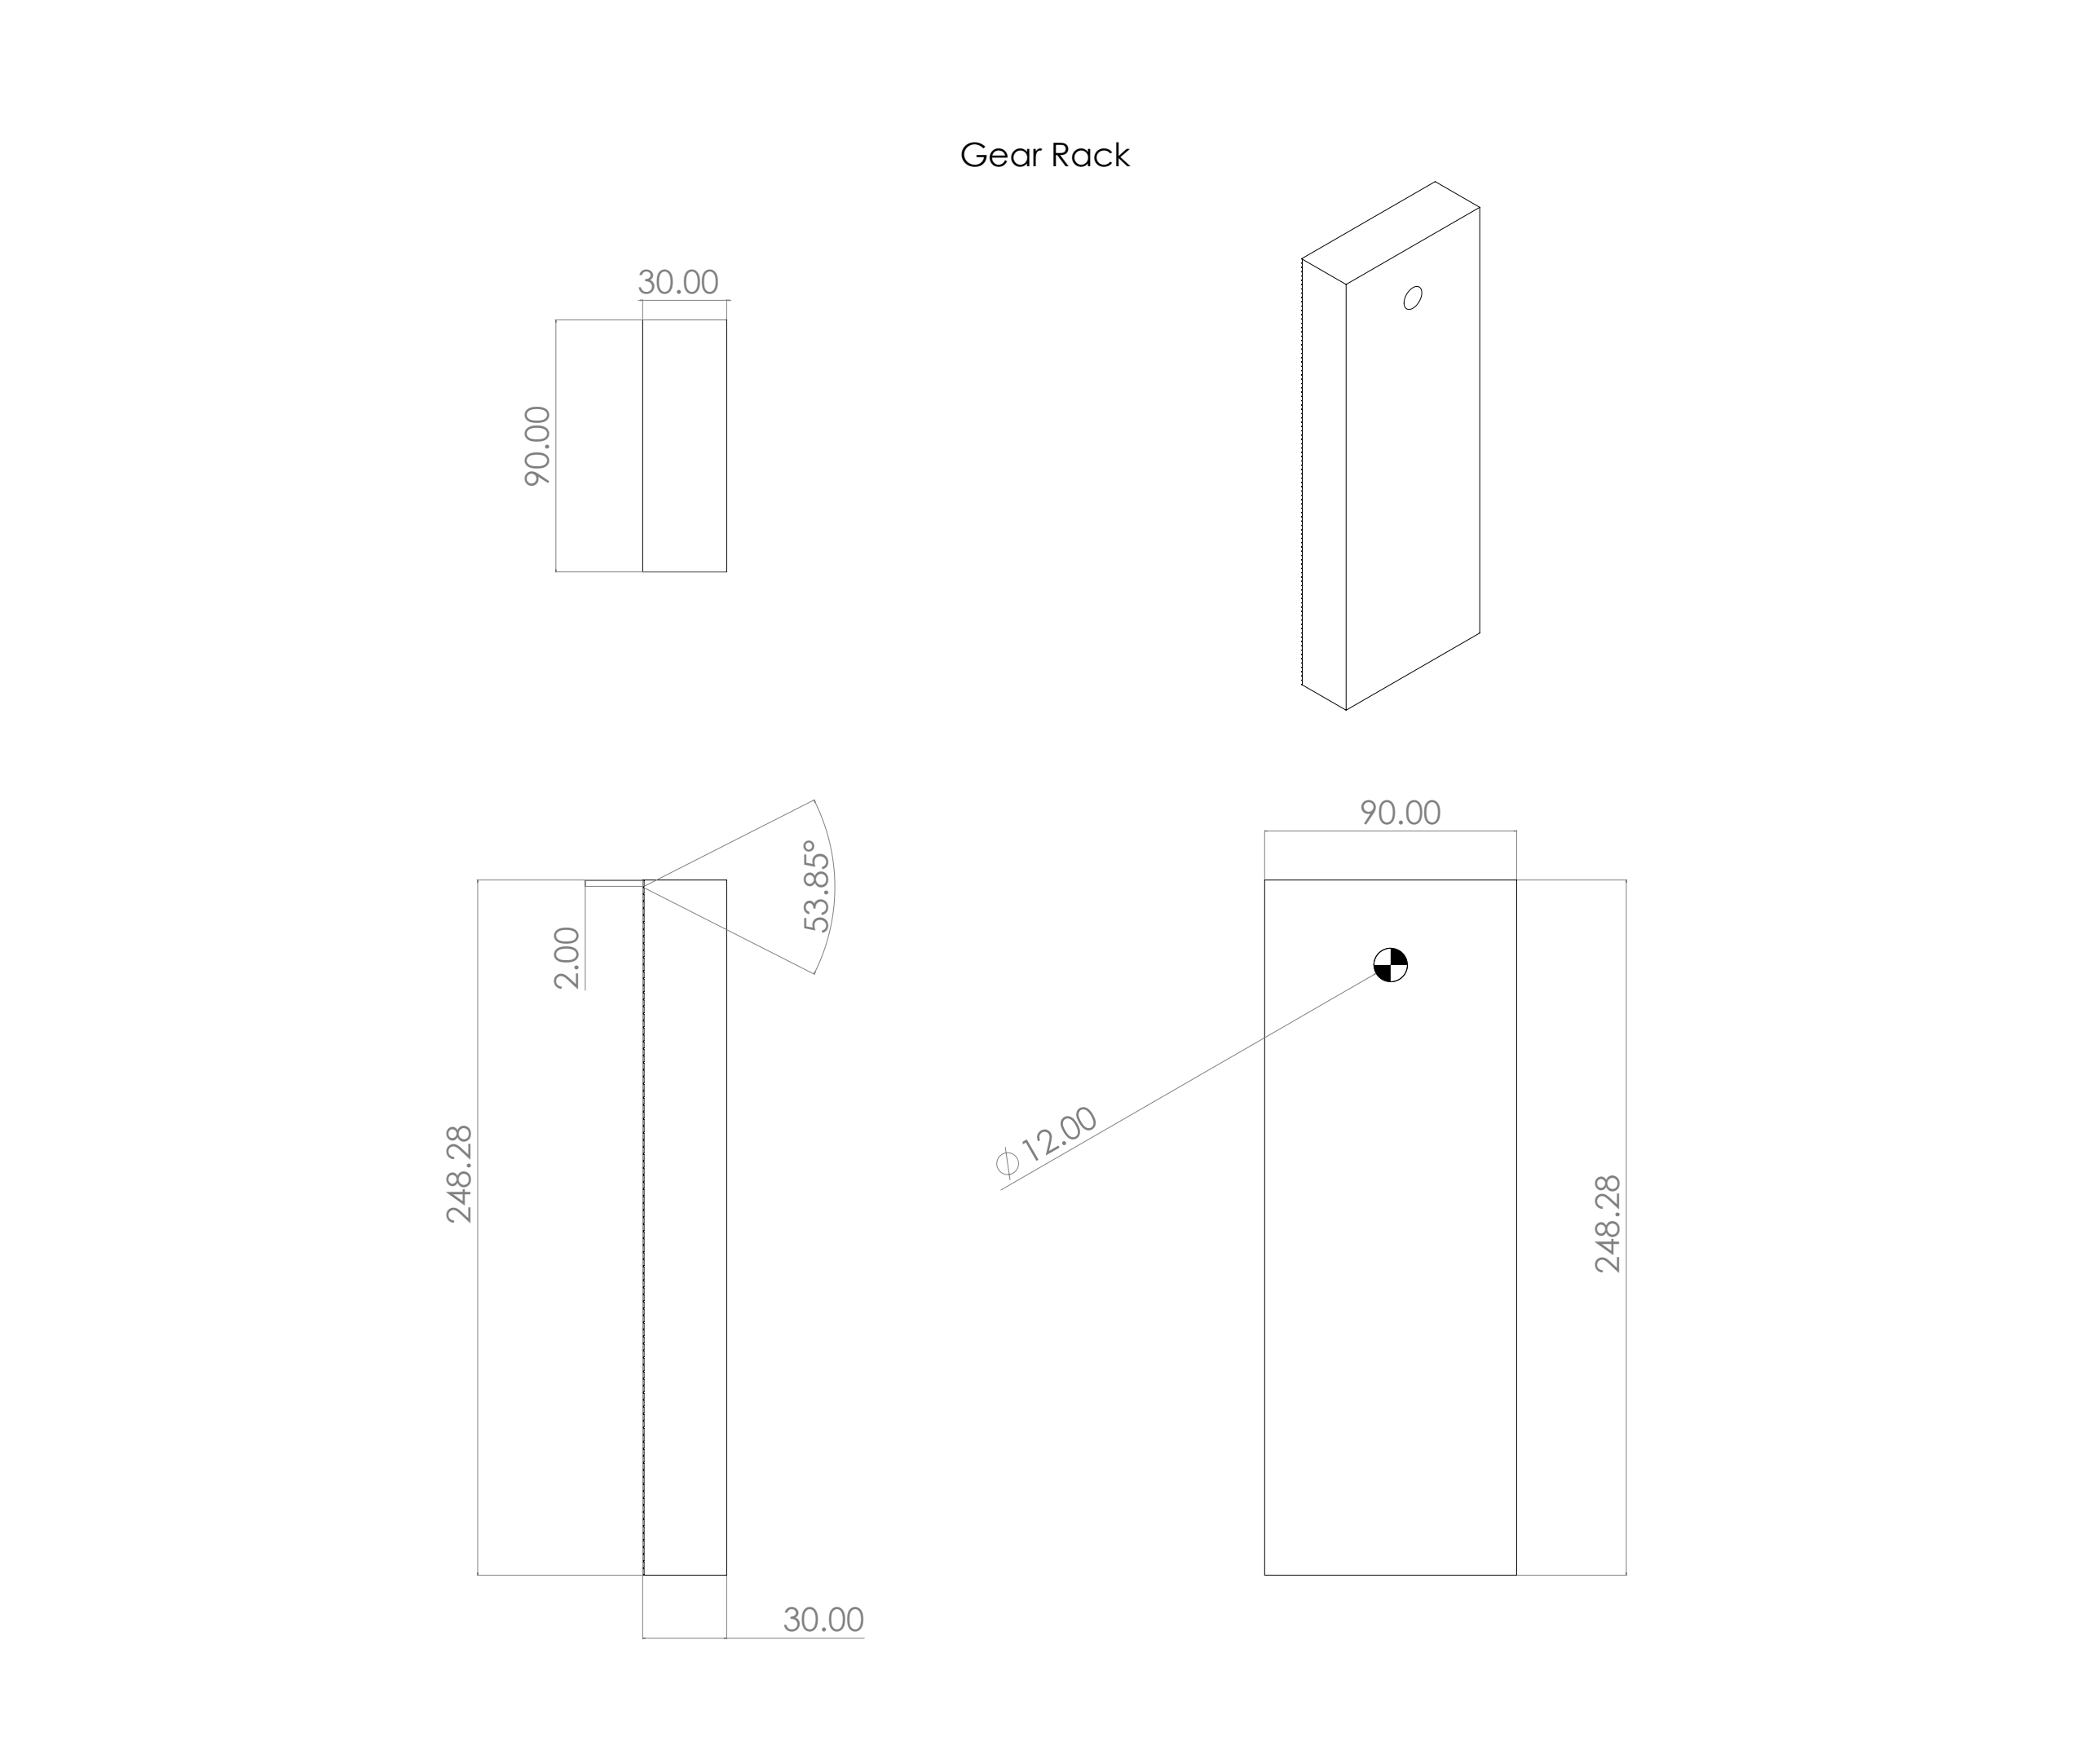
ISO-10303-21;
HEADER;
FILE_DESCRIPTION (('STEP AP214'),
    '1' );
FILE_NAME ('Gear Rack.step',
    '2026-10-24T00:09:50',
    ( '' ),
    ( '' ),
    'SwSTEP 2.0',
    'SolidWorks 2025',
    '' );
FILE_SCHEMA (( 'AUTOMOTIVE_DESIGN' ));
ENDSEC;

DATA;
#4=ORIENTED_EDGE ( 'NONE', *, *, #26664, .T. ) ;
#8=ORIENTED_EDGE ( 'NONE', *, *, #11531, .F. ) ;
#19=EDGE_CURVE ( 'NONE', #26943, #26049, #15367, .T. ) ;
#20=CARTESIAN_POINT ( 'NONE',  ( 157.4999999999998579, 83.32081209086616980, 45.00000000000000000 ) ) ;
#25=CARTESIAN_POINT ( 'NONE',  ( 187.4999999999996305, 288.9665627064425166, 45.00000000000000000 ) ) ;
#27=ORIENTED_EDGE ( 'NONE', *, *, #22527, .F. ) ;
#29=CARTESIAN_POINT ( 'NONE',  ( 157.4999999999998579, 105.8916871584295478, 45.00000000000000000 ) ) ;
#30=CARTESIAN_POINT ( 'NONE',  ( 158.0000000000016485, 50.46449948952111697, 45.00000000000000000 ) ) ;
#31=LINE ( 'NONE', #28308, #26698 ) ;
#33=ORIENTED_EDGE ( 'NONE', *, *, #12258, .T. ) ;
#34=EDGE_CURVE ( 'NONE', #22143, #25491, #9030, .T. ) ;
#35=DIRECTION ( 'NONE',  ( -0.8916010070293783896, -0.4528218681382319422, 0.000000000000000000 ) ) ;
#36=VECTOR ( 'NONE', #4972, 999.9999999999998863 ) ;
#37=CARTESIAN_POINT ( 'NONE',  ( 158.0000000000006821, 140.7479997597746433, 45.00000000000000000 ) ) ;
#39=ORIENTED_EDGE ( 'NONE', *, *, #23270, .T. ) ;
#41=EDGE_CURVE ( 'NONE', #5835, #23775, #13490, .T. ) ;
#48=FACE_OUTER_BOUND ( 'NONE', #22018, .T. ) ;
#49=ORIENTED_EDGE ( 'NONE', *, *, #10620, .T. ) ;
#54=EDGE_CURVE ( 'NONE', #1139, #21808, #13638, .T. ) ;
#56=CARTESIAN_POINT ( 'NONE',  ( 158.0000000000000568, 203.4448749474510407, 45.00000000000000000 ) ) ;
#57=CARTESIAN_POINT ( 'NONE',  ( 158.0000000000006821, 138.7479997597746433, 45.00000000000000000 ) ) ;
#58=DIRECTION ( 'NONE',  ( -0.000000000000000000, -0.000000000000000000, -1.000000000000000000 ) ) ;
#60=LINE ( 'NONE', #17580, #15416 ) ;
#61=VERTEX_POINT ( 'NONE', #7448 ) ;
#62=DIRECTION ( 'NONE',  ( 0.000000000000000000, 0.000000000000000000, 1.000000000000000000 ) ) ;
#64=FACE_OUTER_BOUND ( 'NONE', #25797, .T. ) ;
#65=CARTESIAN_POINT ( 'NONE',  ( 157.4999999999998579, 93.35231212089433939, 45.00000000000000000 ) ) ;
#68=CARTESIAN_POINT ( 'NONE',  ( 157.4999999999998579, 98.36806213590843129, -45.00000000000000000 ) ) ;
#70=VECTOR ( 'NONE', #14918, 1000.000000000000114 ) ;
#77=VECTOR ( 'NONE', #23464, 999.9999999999998863 ) ;
#81=ORIENTED_EDGE ( 'NONE', *, *, #14673, .T. ) ;
#83=VERTEX_POINT ( 'NONE', #22814 ) ;
#85=ORIENTED_EDGE ( 'NONE', *, *, #17813, .T. ) ;
#87=ORIENTED_EDGE ( 'NONE', *, *, #18331, .F. ) ;
#91=AXIS2_PLACEMENT_3D ( 'NONE', #3202, #20878, #24911 ) ;
#92=DIRECTION ( 'NONE',  ( 0.8916010070295410372, -0.4528218681379115873, 0.000000000000000000 ) ) ;
#96=LINE ( 'NONE', #11159, #22961 ) ;
#100=DIRECTION ( 'NONE',  ( 0.000000000000000000, -1.000000000000000000, 0.000000000000000000 ) ) ;
#105=PLANE ( 'NONE',  #22522 ) ;
#106=DIRECTION ( 'NONE',  ( 0.8916010070293283185, 0.4528218681383305855, 0.000000000000000000 ) ) ;
#107=CARTESIAN_POINT ( 'NONE',  ( 158.0000000000012221, 88.59049960963380954, -45.00000000000000000 ) ) ;
#110=ORIENTED_EDGE ( 'NONE', *, *, #7705, .T. ) ;
#111=EDGE_CURVE ( 'NONE', #4742, #22382, #9467, .T. ) ;
#112=VECTOR ( 'NONE', #9793, 1000.000000000000000 ) ;
#114=EDGE_LOOP ( 'NONE', ( #13763, #3696, #24044, #20717 ) ) ;
#116=ORIENTED_EDGE ( 'NONE', *, *, #27781, .F. ) ;
#123=DIRECTION ( 'NONE',  ( 0.8916010070293710621, -0.4528218681382463195, 0.000000000000000000 ) ) ;
#127=VECTOR ( 'NONE', #25950, 1000.000000000000000 ) ;
#129=LINE ( 'NONE', #12656, #21109 ) ;
#131=VECTOR ( 'NONE', #4235, 1000.000000000000000 ) ;
#137=FACE_OUTER_BOUND ( 'NONE', #15642, .T. ) ;
#138=VECTOR ( 'NONE', #24642, 1000.000000000000000 ) ;
#143=LINE ( 'NONE', #23706, #15280 ) ;
#150=DIRECTION ( 'NONE',  ( 0.000000000000000000, -1.000000000000000000, 0.000000000000000000 ) ) ;
#151=ORIENTED_EDGE ( 'NONE', *, *, #11275, .F. ) ;
#152=VERTEX_POINT ( 'NONE', #25244 ) ;
#153=VECTOR ( 'NONE', #12581, 1000.000000000000000 ) ;
#161=CARTESIAN_POINT ( 'NONE',  ( 157.9999999999996589, 279.1890001801680796, 45.00000000000000000 ) ) ;
#162=ORIENTED_EDGE ( 'NONE', *, *, #25176, .F. ) ;
#167=VECTOR ( 'NONE', #6302, 1000.000000000000000 ) ;
#169=EDGE_CURVE ( 'NONE', #1220, #7618, #16907, .T. ) ;
#170=VERTEX_POINT ( 'NONE', #23513 ) ;
#172=DIRECTION ( 'NONE',  ( 0.8916010070298353574, -0.4528218681373320509, 0.000000000000000000 ) ) ;
#174=CARTESIAN_POINT ( 'NONE',  ( 158.0000000000004832, 161.3188748273380213, 45.00000000000000000 ) ) ;
#176=VECTOR ( 'NONE', #1198, 1000.000000000000000 ) ;
#179=LINE ( 'NONE', #13127, #5008 ) ;
#180=ADVANCED_FACE ( 'NONE', ( #3827 ), #7726, .F. ) ;
#189=EDGE_LOOP ( 'NONE', ( #11478, #20043, #1558, #19553 ) ) ;
#190=VECTOR ( 'NONE', #9323, 1000.000000000000227 ) ;
#191=ORIENTED_EDGE ( 'NONE', *, *, #11968, .F. ) ;
#199=CARTESIAN_POINT ( 'NONE',  ( 157.4999999999997442, 253.8563126013445697, -45.00000000000000000 ) ) ;
#200=CARTESIAN_POINT ( 'NONE',  ( 158.0000000000017053, 45.44874947450702507, 45.00000000000000000 ) ) ;
#207=EDGE_LOOP ( 'NONE', ( #12910, #1760, #26526, #6163 ) ) ;
#208=LINE ( 'NONE', #21895, #12696 ) ;
#216=CARTESIAN_POINT ( 'NONE',  ( 158.0000000000001421, 191.4133749174225443, 45.00000000000000000 ) ) ;
#217=LINE ( 'NONE', #22769, #1813 ) ;
#219=ORIENTED_EDGE ( 'NONE', *, *, #15468, .T. ) ;
#222=VECTOR ( 'NONE', #16891, 1000.000000000000000 ) ;
#224=ADVANCED_FACE ( 'NONE', ( #25661 ), #17044, .F. ) ;
#226=VERTEX_POINT ( 'NONE', #23659 ) ;
#228=FACE_OUTER_BOUND ( 'NONE', #26705, .T. ) ;
#229=ORIENTED_EDGE ( 'NONE', *, *, #19889, .T. ) ;
#231=DIRECTION ( 'NONE',  ( 1.000000000000000000, 0.000000000000000000, -0.000000000000000000 ) ) ;
#233=ORIENTED_EDGE ( 'NONE', *, *, #12489, .T. ) ;
#237=VECTOR ( 'NONE', #8756, 1000.000000000000000 ) ;
#244=DIRECTION ( 'NONE',  ( -0.000000000000000000, -0.000000000000000000, -1.000000000000000000 ) ) ;
#247=CARTESIAN_POINT ( 'NONE',  ( 158.0000000000007674, 133.2243747372535267, -45.00000000000000000 ) ) ;
#248=CARTESIAN_POINT ( 'NONE',  ( 158.0000000000003411, 173.8582498648732440, -45.00000000000000000 ) ) ;
#249=LINE ( 'NONE', #6703, #21167 ) ;
#252=ORIENTED_EDGE ( 'NONE', *, *, #25685, .T. ) ;
#258=VECTOR ( 'NONE', #9581, 1000.000000000000000 ) ;
#265=ORIENTED_EDGE ( 'NONE', *, *, #8156, .T. ) ;
#271=CARTESIAN_POINT ( 'NONE',  ( 157.4999999999998579, 183.6358123911478799, 45.00000000000000000 ) ) ;
#273=VECTOR ( 'NONE', #6730, 1000.000000000000000 ) ;
#276=EDGE_CURVE ( 'NONE', #11934, #27327, #6832, .T. ) ;
#278=EDGE_CURVE ( 'NONE', #18107, #2726, #15475, .T. ) ;
#281=PLANE ( 'NONE',  #14960 ) ;
#284=CARTESIAN_POINT ( 'NONE',  ( 157.4999999999998579, 163.5728123310915407, 45.00000000000000000 ) ) ;
#287=LINE ( 'NONE', #25846, #26979 ) ;
#289=LINE ( 'NONE', #2568, #5884 ) ;
#293=ORIENTED_EDGE ( 'NONE', *, *, #15468, .F. ) ;
#296=DIRECTION ( 'NONE',  ( -0.000000000000000000, -0.000000000000000000, -1.000000000000000000 ) ) ;
#298=ORIENTED_EDGE ( 'NONE', *, *, #15430, .T. ) ;
#299=ORIENTED_EDGE ( 'NONE', *, *, #27948, .T. ) ;
#300=VECTOR ( 'NONE', #28359, 1000.000000000000000 ) ;
#302=LINE ( 'NONE', #15395, #9767 ) ;
#306=ORIENTED_EDGE ( 'NONE', *, *, #8739, .F. ) ;
#307=CARTESIAN_POINT ( 'NONE',  ( 157.4999999999996589, 276.4271876689075498, 45.00000000000000000 ) ) ;
#314=ADVANCED_FACE ( 'NONE', ( #8712 ), #4110, .F. ) ;
#321=PLANE ( 'NONE',  #16025 ) ;
#326=DIRECTION ( 'NONE',  ( -0.8916010070300282031, 0.4528218681369524101, 0.000000000000000000 ) ) ;
#329=ORIENTED_EDGE ( 'NONE', *, *, #12094, .T. ) ;
#330=ORIENTED_EDGE ( 'NONE', *, *, #4768, .T. ) ;
#333=ORIENTED_EDGE ( 'NONE', *, *, #4508, .T. ) ;
#334=VECTOR ( 'NONE', #5178, 1000.000000000000000 ) ;
#344=ADVANCED_FACE ( 'NONE', ( #18569 ), #902, .F. ) ;
#345=FACE_OUTER_BOUND ( 'NONE', #10535, .T. ) ;
#346=DIRECTION ( 'NONE',  ( 1.000000000000000000, 0.000000000000000000, -0.000000000000000000 ) ) ;
#350=PLANE ( 'NONE',  #14058 ) ;
#351=ORIENTED_EDGE ( 'NONE', *, *, #20821, .F. ) ;
#353=LINE ( 'NONE', #9111, #26676 ) ;
#354=CARTESIAN_POINT ( 'NONE',  ( 158.0000000000009095, 118.6849996997183041, -45.00000000000000000 ) ) ;
#355=CARTESIAN_POINT ( 'NONE',  ( 158.0000000000011937, 91.09837461714084839, 45.00000000000000000 ) ) ;
#357=ORIENTED_EDGE ( 'NONE', *, *, #17681, .T. ) ;
#358=CARTESIAN_POINT ( 'NONE',  ( 157.4999999999998579, 75.79718706834503905, -45.00000000000000000 ) ) ;
#359=ORIENTED_EDGE ( 'NONE', *, *, #19187, .F. ) ;
#360=LINE ( 'NONE', #2786, #27655 ) ;
#363=ORIENTED_EDGE ( 'NONE', *, *, #1797, .T. ) ;
#364=DIRECTION ( 'NONE',  ( -0.000000000000000000, -0.000000000000000000, -1.000000000000000000 ) ) ;
#367=CARTESIAN_POINT ( 'NONE',  ( 158.0000000000009948, 110.6534996696901345, 45.00000000000000000 ) ) ;
#369=DIRECTION ( 'NONE',  ( 0.4528218681382713551, -0.8916010070293584056, 0.000000000000000000 ) ) ;
#372=VERTEX_POINT ( 'NONE', #14405 ) ;
#374=ORIENTED_EDGE ( 'NONE', *, *, #24300, .F. ) ;
#375=VECTOR ( 'NONE', #26131, 1000.000000000000000 ) ;
#376=EDGE_CURVE ( 'NONE', #12778, #5204, #20994, .T. ) ;
#378=VERTEX_POINT ( 'NONE', #12116 ) ;
#382=DIRECTION ( 'NONE',  ( 0.4528218681372921939, 0.8916010070298556744, -0.000000000000000000 ) ) ;
#386=EDGE_CURVE ( 'NONE', #7620, #226, #11835, .T. ) ;
#387=VECTOR ( 'NONE', #7151, 1000.000000000000000 ) ;
#389=LINE ( 'NONE', #22364, #14037 ) ;
#390=CARTESIAN_POINT ( 'NONE',  ( 158.0000000000001990, 188.3976249024084666, 45.00000000000000000 ) ) ;
#391=LINE ( 'NONE', #13469, #619 ) ;
#392=EDGE_LOOP ( 'NONE', ( #28228, #13403, #15144, #3135 ) ) ;
#394=AXIS2_PLACEMENT_3D ( 'NONE', #22078, #2964, #5263 ) ;
#397=DIRECTION ( 'NONE',  ( -0.8916010070293711731, 0.4528218681382463751, 0.000000000000000000 ) ) ;
#405=ORIENTED_EDGE ( 'NONE', *, *, #27601, .F. ) ;
#410=VERTEX_POINT ( 'NONE', #9531 ) ;
#412=PLANE ( 'NONE',  #4933 ) ;
#413=LINE ( 'NONE', #26684, #6547 ) ;
#418=EDGE_CURVE ( 'NONE', #905, #12668, #18291, .T. ) ;
#422=EDGE_CURVE ( 'NONE', #9422, #12999, #20714, .T. ) ;
#423=CARTESIAN_POINT ( 'NONE',  ( 158.0000000000015348, 58.49599951954928656, -45.00000000000000000 ) ) ;
#424=CARTESIAN_POINT ( 'NONE',  ( 158.0000000000016485, 48.46449948952110987, -45.00000000000000000 ) ) ;
#432=CARTESIAN_POINT ( 'NONE',  ( 158.0000000000015632, 57.98812451204224061, 45.00000000000000000 ) ) ;
#435=EDGE_LOOP ( 'NONE', ( #624, #23156, #10826, #824 ) ) ;
#436=EDGE_CURVE ( 'NONE', #9697, #410, #7928, .T. ) ;
#437=DIRECTION ( 'NONE',  ( -0.000000000000000000, 0.000000000000000000, -1.000000000000000000 ) ) ;
#448=EDGE_CURVE ( 'NONE', #7332, #22290, #1039, .T. ) ;
#450=LINE ( 'NONE', #307, #16398 ) ;
#454=DIRECTION ( 'NONE',  ( 0.000000000000000000, -1.000000000000000000, 0.000000000000000000 ) ) ;
#455=LINE ( 'NONE', #4177, #5667 ) ;
#456=VECTOR ( 'NONE', #13195, 1000.000000000000000 ) ;
#458=LINE ( 'NONE', #9217, #23812 ) ;
#461=DIRECTION ( 'NONE',  ( 1.000000000000000000, 0.000000000000000000, -0.000000000000000000 ) ) ;
#464=CARTESIAN_POINT ( 'NONE',  ( 158.0000000000012790, 83.57474959461971764, -45.00000000000000000 ) ) ;
#465=VERTEX_POINT ( 'NONE', #23870 ) ;
#477=VERTEX_POINT ( 'NONE', #6332 ) ;
#478=ORIENTED_EDGE ( 'NONE', *, *, #3698, .F. ) ;
#479=DIRECTION ( 'NONE',  ( -0.8916010070298252543, 0.4528218681373520904, 0.000000000000000000 ) ) ;
#482=CARTESIAN_POINT ( 'NONE',  ( 157.4999999999998579, 63.25781203080982351, 45.00000000000000000 ) ) ;
#485=VECTOR ( 'NONE', #5220, 999.9999999999998863 ) ;
#486=EDGE_CURVE ( 'NONE', #2468, #22451, #19269, .T. ) ;
#487=CARTESIAN_POINT ( 'NONE',  ( 158.0000000000007390, 135.7322497447605656, -45.00000000000000000 ) ) ;
#495=EDGE_CURVE ( 'NONE', #465, #26764, #24012, .T. ) ;
#497=DIRECTION ( 'NONE',  ( -0.8916010070293783896, -0.4528218681382319422, 0.000000000000000000 ) ) ;
#503=DIRECTION ( 'NONE',  ( -0.000000000000000000, -0.000000000000000000, -1.000000000000000000 ) ) ;
#507=CARTESIAN_POINT ( 'NONE',  ( 158.0000000000009663, 113.1613746771971876, 45.00000000000000000 ) ) ;
#510=ADVANCED_FACE ( 'NONE', ( #1873 ), #18986, .F. ) ;
#513=EDGE_LOOP ( 'NONE', ( #20470, #9702, #23689, #21030 ) ) ;
#514=EDGE_CURVE ( 'NONE', #16325, #12071, #12961, .T. ) ;
#518=PLANE ( 'NONE',  #26438 ) ;
#524=LINE ( 'NONE', #27357, #13105 ) ;
#526=CARTESIAN_POINT ( 'NONE',  ( 158.0000000000002274, 183.8897498949014278, 45.00000000000000000 ) ) ;
#532=CARTESIAN_POINT ( 'NONE',  ( 157.4999999999998579, 105.8916871584295478, -45.00000000000000000 ) ) ;
#534=LINE ( 'NONE', #11755, #24010 ) ;
#537=CARTESIAN_POINT ( 'NONE',  ( 157.4999999999998010, 241.3169375638095460, -45.00000000000000000 ) ) ;
#540=CARTESIAN_POINT ( 'NONE',  ( 157.4999999999998579, 191.1594374136689964, -45.00000000000000000 ) ) ;
#542=PLANE ( 'NONE',  #20720 ) ;
#543=VERTEX_POINT ( 'NONE', #17395 ) ;
#546=EDGE_CURVE ( 'NONE', #991, #20740, #6197, .T. ) ;
#547=CARTESIAN_POINT ( 'NONE',  ( 157.4999999999998579, 153.5413123010633853, 45.00000000000000000 ) ) ;
#548=VERTEX_POINT ( 'NONE', #21136 ) ;
#552=ORIENTED_EDGE ( 'NONE', *, *, #17681, .F. ) ;
#563=CARTESIAN_POINT ( 'NONE',  ( 157.9999999999996874, 268.6496251426330559, -45.00000000000000000 ) ) ;
#564=LINE ( 'NONE', #17941, #18623 ) ;
#569=CARTESIAN_POINT ( 'NONE',  ( 157.9999999999998010, 238.5551250525490161, 45.00000000000000000 ) ) ;
#571=VECTOR ( 'NONE', #26169, 1000.000000000000227 ) ;
#574=CARTESIAN_POINT ( 'NONE',  ( 158.0000000000013358, 78.55899957960562574, -45.00000000000000000 ) ) ;
#577=ORIENTED_EDGE ( 'NONE', *, *, #22638, .T. ) ;
#579=DIRECTION ( 'NONE',  ( -0.8916010070293783896, -0.4528218681382319422, 0.000000000000000000 ) ) ;
#580=AXIS2_PLACEMENT_3D ( 'NONE', #3424, #12354, #8027 ) ;
#582=ORIENTED_EDGE ( 'NONE', *, *, #19199, .T. ) ;
#583=VERTEX_POINT ( 'NONE', #15541 ) ;
#585=EDGE_CURVE ( 'NONE', #16172, #22496, #15834, .T. ) ;
#588=CARTESIAN_POINT ( 'NONE',  ( 157.9999999999998010, 236.5551250525490161, -45.00000000000000000 ) ) ;
#590=EDGE_LOOP ( 'NONE', ( #18071, #20954, #25827, #7929 ) ) ;
#602=EDGE_CURVE ( 'NONE', #11526, #18196, #21990, .T. ) ;
#608=EDGE_CURVE ( 'NONE', #5724, #21166, #15684, .T. ) ;
#615=VECTOR ( 'NONE', #20884, 1000.000000000000114 ) ;
#619=VECTOR ( 'NONE', #22222, 1000.000000000000000 ) ;
#620=VERTEX_POINT ( 'NONE', #11079 ) ;
#624=ORIENTED_EDGE ( 'NONE', *, *, #701, .T. ) ;
#628=DIRECTION ( 'NONE',  ( 0.4528218681370924092, 0.8916010070299572599, -0.000000000000000000 ) ) ;
#632=VECTOR ( 'NONE', #24895, 1000.000000000000000 ) ;
#633=DIRECTION ( 'NONE',  ( 1.000000000000000000, 0.000000000000000000, -0.000000000000000000 ) ) ;
#643=CARTESIAN_POINT ( 'NONE',  ( 158.0000000000003126, 176.3661248723802828, 45.00000000000000000 ) ) ;
#646=ORIENTED_EDGE ( 'NONE', *, *, #18826, .T. ) ;
#648=ORIENTED_EDGE ( 'NONE', *, *, #18190, .T. ) ;
#650=LINE ( 'NONE', #20465, #20665 ) ;
#652=ORIENTED_EDGE ( 'NONE', *, *, #23081, .T. ) ;
#655=VECTOR ( 'NONE', #25630, 1000.000000000000000 ) ;
#659=ORIENTED_EDGE ( 'NONE', *, *, #1539, .T. ) ;
#660=VECTOR ( 'NONE', #1060, 1000.000000000000114 ) ;
#664=EDGE_CURVE ( 'NONE', #22382, #5522, #13383, .T. ) ;
#666=ORIENTED_EDGE ( 'NONE', *, *, #14204, .T. ) ;
#670=EDGE_CURVE ( 'NONE', #15969, #22271, #11226, .T. ) ;
#679=CARTESIAN_POINT ( 'NONE',  ( 158.0000000000009379, 116.1771246922112653, 45.00000000000000000 ) ) ;
#685=DIRECTION ( 'NONE',  ( 1.000000000000000000, 0.000000000000000000, -0.000000000000000000 ) ) ;
#689=VERTEX_POINT ( 'NONE', #9212 ) ;
#692=VECTOR ( 'NONE', #27394, 1000.000000000000114 ) ;
#693=ORIENTED_EDGE ( 'NONE', *, *, #10754, .F. ) ;
#695=VERTEX_POINT ( 'NONE', #161 ) ;
#697=ORIENTED_EDGE ( 'NONE', *, *, #18565, .F. ) ;
#699=DIRECTION ( 'NONE',  ( 0.4528218681376512400, -0.8916010070296733758, 0.000000000000000000 ) ) ;
#701=EDGE_CURVE ( 'NONE', #9383, #10330, #21856, .T. ) ;
#711=CARTESIAN_POINT ( 'NONE',  ( 157.4999999999998579, 105.8916871584295478, 45.00000000000000000 ) ) ;
#712=CARTESIAN_POINT ( 'NONE',  ( 157.4999999999998579, 188.6515624061619576, 45.00000000000000000 ) ) ;
#713=CARTESIAN_POINT ( 'NONE',  ( 157.4999999999998579, 75.79718706834503905, 45.00000000000000000 ) ) ;
#723=ORIENTED_EDGE ( 'NONE', *, *, #775, .T. ) ;
#725=ORIENTED_EDGE ( 'NONE', *, *, #13975, .T. ) ;
#727=FACE_OUTER_BOUND ( 'NONE', #4250, .T. ) ;
#729=VERTEX_POINT ( 'NONE', #20 ) ;
#730=ORIENTED_EDGE ( 'NONE', *, *, #11239, .F. ) ;
#733=VECTOR ( 'NONE', #6685, 1000.000000000000227 ) ;
#734=CARTESIAN_POINT ( 'NONE',  ( 158.0000000000005400, 156.3031248123239436, 45.00000000000000000 ) ) ;
#735=EDGE_CURVE ( 'NONE', #14776, #17184, #8778, .T. ) ;
#736=CARTESIAN_POINT ( 'NONE',  ( 157.9999999999996589, 276.1732501651540588, 45.00000000000000000 ) ) ;
#738=AXIS2_PLACEMENT_3D ( 'NONE', #16780, #14771, #23524 ) ;
#741=LINE ( 'NONE', #5326, #18696 ) ;
#744=ADVANCED_FACE ( 'NONE', ( #5030 ), #27419, .F. ) ;
#745=LINE ( 'NONE', #26587, #14618 ) ;
#747=LINE ( 'NONE', #24592, #112 ) ;
#748=CARTESIAN_POINT ( 'NONE',  ( 157.4999999999998295, 228.7775625262745223, 45.00000000000000000 ) ) ;
#749=VERTEX_POINT ( 'NONE', #25137 ) ;
#753=CARTESIAN_POINT ( 'NONE',  ( 158.0000000000009095, 118.6849996997183041, 45.00000000000000000 ) ) ;
#756=ORIENTED_EDGE ( 'NONE', *, *, #4498, .T. ) ;
#758=EDGE_CURVE ( 'NONE', #11111, #19970, #7626, .T. ) ;
#759=LINE ( 'NONE', #16277, #22117 ) ;
#767=FACE_OUTER_BOUND ( 'NONE', #3565, .T. ) ;
#768=ORIENTED_EDGE ( 'NONE', *, *, #27927, .F. ) ;
#775=EDGE_CURVE ( 'NONE', #20816, #23826, #7896, .T. ) ;
#778=ORIENTED_EDGE ( 'NONE', *, *, #27716, .F. ) ;
#784=EDGE_LOOP ( 'NONE', ( #27213, #18467, #26244, #20332 ) ) ;
#785=DIRECTION ( 'NONE',  ( 0.000000000000000000, -1.000000000000000000, 0.000000000000000000 ) ) ;
#787=LINE ( 'NONE', #12142, #8871 ) ;
#791=DIRECTION ( 'NONE',  ( -0.000000000000000000, -0.000000000000000000, -1.000000000000000000 ) ) ;
#793=VECTOR ( 'NONE', #14680, 1000.000000000000000 ) ;
#794=EDGE_CURVE ( 'NONE', #15105, #2405, #20829, .T. ) ;
#798=ORIENTED_EDGE ( 'NONE', *, *, #12480, .F. ) ;
#799=EDGE_CURVE ( 'NONE', #12071, #26896, #5455, .T. ) ;
#800=VERTEX_POINT ( 'NONE', #13821 ) ;
#805=ORIENTED_EDGE ( 'NONE', *, *, #5908, .F. ) ;
#806=ORIENTED_EDGE ( 'NONE', *, *, #17778, .T. ) ;
#813=FACE_OUTER_BOUND ( 'NONE', #28354, .T. ) ;
#814=CARTESIAN_POINT ( 'NONE',  ( 158.0000000000003126, 176.3661248723802828, 45.00000000000000000 ) ) ;
#816=EDGE_CURVE ( 'NONE', #10360, #6691, #22989, .T. ) ;
#818=DIRECTION ( 'NONE',  ( 0.8916010070293510781, -0.4528218681382856770, 0.000000000000000000 ) ) ;
#824=ORIENTED_EDGE ( 'NONE', *, *, #23421, .T. ) ;
#826=LINE ( 'NONE', #12322, #17561 ) ;
#828=CARTESIAN_POINT ( 'NONE',  ( 158.0000000000009095, 118.6849996997183041, -45.00000000000000000 ) ) ;
#829=ORIENTED_EDGE ( 'NONE', *, *, #22521, .F. ) ;
#833=ORIENTED_EDGE ( 'NONE', *, *, #27551, .T. ) ;
#836=LINE ( 'NONE', #15335, #13752 ) ;
#837=DIRECTION ( 'NONE',  ( 0.8916010070295106171, -0.4528218681379715393, 0.000000000000000000 ) ) ;
#838=VECTOR ( 'NONE', #12878, 1000.000000000000000 ) ;
#839=DIRECTION ( 'NONE',  ( 0.8916010070300181001, -0.4528218681369723941, 0.000000000000000000 ) ) ;
#843=AXIS2_PLACEMENT_3D ( 'NONE', #16057, #23075, #9861 ) ;
#845=DIRECTION ( 'NONE',  ( 0.8916010070293383105, -0.4528218681383106015, 0.000000000000000000 ) ) ;
#849=DIRECTION ( 'NONE',  ( 1.000000000000000000, 0.000000000000000000, -0.000000000000000000 ) ) ;
#855=VERTEX_POINT ( 'NONE', #3153 ) ;
#856=ORIENTED_EDGE ( 'NONE', *, *, #8614, .F. ) ;
#857=DIRECTION ( 'NONE',  ( -0.000000000000000000, -0.000000000000000000, -1.000000000000000000 ) ) ;
#858=VECTOR ( 'NONE', #5187, 1000.000000000000227 ) ;
#867=VECTOR ( 'NONE', #14346, 1000.000000000000227 ) ;
#869=ORIENTED_EDGE ( 'NONE', *, *, #14849, .F. ) ;
#872=DIRECTION ( 'NONE',  ( -0.8916010070299673629, 0.4528218681370723142, 0.000000000000000000 ) ) ;
#876=PLANE ( 'NONE',  #27398 ) ;
#879=FACE_OUTER_BOUND ( 'NONE', #7048, .T. ) ;
#880=FACE_OUTER_BOUND ( 'NONE', #24338, .T. ) ;
#882=FACE_OUTER_BOUND ( 'NONE', #28083, .T. ) ;
#883=VERTEX_POINT ( 'NONE', #24724 ) ;
#885=EDGE_CURVE ( 'NONE', #13594, #27610, #20406, .T. ) ;
#890=ORIENTED_EDGE ( 'NONE', *, *, #18434, .F. ) ;
#892=AXIS2_PLACEMENT_3D ( 'NONE', #17470, #382, #19632 ) ;
#897=ORIENTED_EDGE ( 'NONE', *, *, #21725, .F. ) ;
#898=CARTESIAN_POINT ( 'NONE',  ( 157.9999999999998010, 236.0472500450420341, 45.00000000000000000 ) ) ;
#899=VECTOR ( 'NONE', #15523, 1000.000000000000000 ) ;
#901=DIRECTION ( 'NONE',  ( 0.000000000000000000, -1.000000000000000000, 0.000000000000000000 ) ) ;
#902=PLANE ( 'NONE',  #17386 ) ;
#904=LINE ( 'NONE', #22604, #27037 ) ;
#905=VERTEX_POINT ( 'NONE', #16805 ) ;
#906=CARTESIAN_POINT ( 'NONE',  ( 157.4999999999998579, 125.9546872184859012, -45.00000000000000000 ) ) ;
#908=FACE_OUTER_BOUND ( 'NONE', #24115, .T. ) ;
#918=DIRECTION ( 'NONE',  ( 0.000000000000000000, -1.000000000000000000, 0.000000000000000000 ) ) ;
#923=ORIENTED_EDGE ( 'NONE', *, *, #23688, .T. ) ;
#924=EDGE_CURVE ( 'NONE', #19307, #27610, #27839, .T. ) ;
#926=DIRECTION ( 'NONE',  ( -0.8916010070293409751, -0.4528218681383056610, 0.000000000000000000 ) ) ;
#927=CARTESIAN_POINT ( 'NONE',  ( 158.0000000000008527, 123.7007497147323960, 45.00000000000000000 ) ) ;
#930=ORIENTED_EDGE ( 'NONE', *, *, #5858, .F. ) ;
#931=CARTESIAN_POINT ( 'NONE',  ( 158.0000000000012221, 88.59049960963380954, 45.00000000000000000 ) ) ;
#934=ORIENTED_EDGE ( 'NONE', *, *, #23204, .T. ) ;
#935=CARTESIAN_POINT ( 'NONE',  ( 157.4999999999998579, 171.0964373536126573, -45.00000000000000000 ) ) ;
#936=ORIENTED_EDGE ( 'NONE', *, *, #5812, .F. ) ;
#939=ADVANCED_FACE ( 'NONE', ( #16943 ), #28267, .F. ) ;
#940=ORIENTED_EDGE ( 'NONE', *, *, #27692, .F. ) ;
#941=ORIENTED_EDGE ( 'NONE', *, *, #23394, .T. ) ;
#942=CARTESIAN_POINT ( 'NONE',  ( 158.0000000000014495, 66.01962454207041731, 45.00000000000000000 ) ) ;
#949=DIRECTION ( 'NONE',  ( 0.000000000000000000, -1.000000000000000000, 0.000000000000000000 ) ) ;
#954=LINE ( 'NONE', #12451, #19901 ) ;
#956=EDGE_CURVE ( 'NONE', #7560, #13193, #23407, .T. ) ;
#957=AXIS2_PLACEMENT_3D ( 'NONE', #27536, #849, #25400 ) ;
#958=DIRECTION ( 'NONE',  ( 0.4528218681379303501, -0.8916010070295316003, 0.000000000000000000 ) ) ;
#959=DIRECTION ( 'NONE',  ( 0.000000000000000000, -1.000000000000000000, 0.000000000000000000 ) ) ;
#965=ORIENTED_EDGE ( 'NONE', *, *, #5174, .F. ) ;
#966=DIRECTION ( 'NONE',  ( -0.000000000000000000, -0.000000000000000000, -1.000000000000000000 ) ) ;
#969=VERTEX_POINT ( 'NONE', #17222 ) ;
#972=CARTESIAN_POINT ( 'NONE',  ( 157.9999999999996589, 278.6811251726610976, 45.00000000000000000 ) ) ;
#975=FACE_OUTER_BOUND ( 'NONE', #15503, .T. ) ;
#976=DIRECTION ( 'NONE',  ( -0.000000000000000000, 0.000000000000000000, -1.000000000000000000 ) ) ;
#981=CARTESIAN_POINT ( 'NONE',  ( 158.0000000000016769, 47.95662448201407102, 45.00000000000000000 ) ) ;
#982=DIRECTION ( 'NONE',  ( -0.000000000000000000, 0.000000000000000000, -1.000000000000000000 ) ) ;
#983=EDGE_CURVE ( 'NONE', #14755, #9116, #3862, .T. ) ;
#991=VERTEX_POINT ( 'NONE', #4002 ) ;
#992=ORIENTED_EDGE ( 'NONE', *, *, #15561, .F. ) ;
#996=VECTOR ( 'NONE', #5623, 1000.000000000000000 ) ;
#1003=EDGE_CURVE ( 'NONE', #18388, #2119, #10337, .T. ) ;
#1005=CARTESIAN_POINT ( 'NONE',  ( 157.9999999999999716, 210.9684999699701393, 45.00000000000000000 ) ) ;
#1007=AXIS2_PLACEMENT_3D ( 'NONE', #4086, #12870, #21613 ) ;
#1013=CARTESIAN_POINT ( 'NONE',  ( 157.9999999999997442, 254.1102501050980322, 45.00000000000000000 ) ) ;
#1016=ADVANCED_FACE ( 'NONE', ( #21677 ), #10767, .F. ) ;
#1021=LINE ( 'NONE', #26890, #24051 ) ;
#1022=ORIENTED_EDGE ( 'NONE', *, *, #15495, .T. ) ;
#1023=CARTESIAN_POINT ( 'NONE',  ( 157.9999999999998010, 238.5551250525490161, 45.00000000000000000 ) ) ;
#1025=CARTESIAN_POINT ( 'NONE',  ( 158.0000000000009948, 108.6534996696901345, 45.00000000000000000 ) ) ;
#1035=ORIENTED_EDGE ( 'NONE', *, *, #2765, .F. ) ;
#1039=LINE ( 'NONE', #9809, #10502 ) ;
#1042=ORIENTED_EDGE ( 'NONE', *, *, #1210, .T. ) ;
#1043=DIRECTION ( 'NONE',  ( 0.8916010070293584056, -0.4528218681382712996, 0.000000000000000000 ) ) ;
#1044=ADVANCED_FACE ( 'NONE', ( #22244 ), #4850, .F. ) ;
#1047=DIRECTION ( 'NONE',  ( 0.8916010070298258094, 0.4528218681373508137, 0.000000000000000000 ) ) ;
#1049=CARTESIAN_POINT ( 'NONE',  ( 157.9999999999998295, 226.0157500150140208, -45.00000000000000000 ) ) ;
#1052=FACE_OUTER_BOUND ( 'NONE', #20368, .T. ) ;
#1056=CARTESIAN_POINT ( 'NONE',  ( 157.4999999999996874, 271.4114376538935289, 45.00000000000000000 ) ) ;
#1057=ADVANCED_FACE ( 'NONE', ( #26541 ), #2408, .F. ) ;
#1060=DIRECTION ( 'NONE',  ( -0.8916010070297446521, -0.4528218681375106858, 0.000000000000000000 ) ) ;
#1066=PLANE ( 'NONE',  #8262 ) ;
#1067=LINE ( 'NONE', #21162, #5729 ) ;
#1069=LINE ( 'NONE', #18869, #7867 ) ;
#1073=EDGE_LOOP ( 'NONE', ( #5385, #17781, #693, #27335 ) ) ;
#1076=FACE_OUTER_BOUND ( 'NONE', #21023, .T. ) ;
#1078=AXIS2_PLACEMENT_3D ( 'NONE', #16858, #26030, #8234 ) ;
#1086=DIRECTION ( 'NONE',  ( 0.4528218681371510290, -0.8916010070299273949, 0.000000000000000000 ) ) ;
#1088=DIRECTION ( 'NONE',  ( -0.000000000000000000, -0.000000000000000000, -1.000000000000000000 ) ) ;
#1089=LINE ( 'NONE', #13758, #13150 ) ;
#1091=LINE ( 'NONE', #12310, #4041 ) ;
#1095=EDGE_CURVE ( 'NONE', #18723, #12774, #4427, .T. ) ;
#1101=VECTOR ( 'NONE', #18023, 1000.000000000000000 ) ;
#1103=FACE_OUTER_BOUND ( 'NONE', #1724, .T. ) ;
#1104=ORIENTED_EDGE ( 'NONE', *, *, #11937, .F. ) ;
#1106=EDGE_LOOP ( 'NONE', ( #25794, #23031, #16354, #299 ) ) ;
#1108=ORIENTED_EDGE ( 'NONE', *, *, #8766, .T. ) ;
#1109=ADVANCED_FACE ( 'NONE', ( #4709 ), #13494, .F. ) ;
#1110=ORIENTED_EDGE ( 'NONE', *, *, #10106, .T. ) ;
#1111=VERTEX_POINT ( 'NONE', #20083 ) ;
#1114=VECTOR ( 'NONE', #25456, 1000.000000000000000 ) ;
#1119=CARTESIAN_POINT ( 'NONE',  ( 157.4999999999997442, 251.3484375938375024, 45.00000000000000000 ) ) ;
#1127=EDGE_LOOP ( 'NONE', ( #28264, #5730, #17065, #9026 ) ) ;
#1129=LINE ( 'NONE', #5860, #6839 ) ;
#1132=VERTEX_POINT ( 'NONE', #26686 ) ;
#1133=ORIENTED_EDGE ( 'NONE', *, *, #12866, .F. ) ;
#1134=VECTOR ( 'NONE', #17507, 1000.000000000000000 ) ;
#1137=ORIENTED_EDGE ( 'NONE', *, *, #10876, .F. ) ;
#1138=AXIS2_PLACEMENT_3D ( 'NONE', #15635, #24526, #24378 ) ;
#1139=VERTEX_POINT ( 'NONE', #23978 ) ;
#1140=ORIENTED_EDGE ( 'NONE', *, *, #15633, .F. ) ;
#1142=DIRECTION ( 'NONE',  ( -0.000000000000000000, -0.000000000000000000, -1.000000000000000000 ) ) ;
#1144=DIRECTION ( 'NONE',  ( -0.000000000000000000, 0.000000000000000000, -1.000000000000000000 ) ) ;
#1149=EDGE_CURVE ( 'NONE', #12999, #26726, #19664, .T. ) ;
#1151=LINE ( 'NONE', #27287, #12102 ) ;
#1155=DIRECTION ( 'NONE',  ( -0.8916010070298455714, 0.4528218681373120669, 0.000000000000000000 ) ) ;
#1158=CARTESIAN_POINT ( 'NONE',  ( 158.0000000000013642, 76.05112457209858690, -45.00000000000000000 ) ) ;
#1160=FACE_OUTER_BOUND ( 'NONE', #21524, .T. ) ;
#1161=ORIENTED_EDGE ( 'NONE', *, *, #20118, .T. ) ;
#1169=VECTOR ( 'NONE', #12343, 1000.000000000000114 ) ;
#1173=ORIENTED_EDGE ( 'NONE', *, *, #21099, .F. ) ;
#1175=VECTOR ( 'NONE', #2149, 1000.000000000000000 ) ;
#1176=VERTEX_POINT ( 'NONE', #7595 ) ;
#1177=DIRECTION ( 'NONE',  ( 1.000000000000000000, 0.000000000000000000, -0.000000000000000000 ) ) ;
#1178=ADVANCED_FACE ( 'NONE', ( #975 ), #7163, .F. ) ;
#1179=LINE ( 'NONE', #2764, #6588 ) ;
#1180=EDGE_CURVE ( 'NONE', #20032, #27491, #12053, .T. ) ;
#1188=PLANE ( 'NONE',  #15906 ) ;
#1189=FACE_OUTER_BOUND ( 'NONE', #15125, .T. ) ;
#1191=CARTESIAN_POINT ( 'NONE',  ( 158.0000000000006537, 143.7637497747887210, 45.00000000000000000 ) ) ;
#1195=VECTOR ( 'NONE', #9893, 999.9999999999998863 ) ;
#1198=DIRECTION ( 'NONE',  ( 0.000000000000000000, -1.000000000000000000, 0.000000000000000000 ) ) ;
#1200=CARTESIAN_POINT ( 'NONE',  ( 158.0000000000002558, 181.3818748873943889, 45.00000000000000000 ) ) ;
#1203=DIRECTION ( 'NONE',  ( 0.000000000000000000, -1.000000000000000000, 0.000000000000000000 ) ) ;
#1204=CARTESIAN_POINT ( 'NONE',  ( 157.4999999999994600, 216.2381874887387880, 45.00000000000000000 ) ) ;
#1205=LINE ( 'NONE', #27617, #12642 ) ;
#1210=EDGE_CURVE ( 'NONE', #1637, #378, #24687, .T. ) ;
#1213=VERTEX_POINT ( 'NONE', #25106 ) ;
#1215=VERTEX_POINT ( 'NONE', #5423 ) ;
#1217=LINE ( 'NONE', #19159, #2597 ) ;
#1220=VERTEX_POINT ( 'NONE', #27527 ) ;
#1221=AXIS2_PLACEMENT_3D ( 'NONE', #23489, #21469, #12729 ) ;
#1228=LINE ( 'NONE', #27227, #22752 ) ;
#1230=LINE ( 'NONE', #8267, #18652 ) ;
#1231=LINE ( 'NONE', #27231, #25754 ) ;
#1232=CARTESIAN_POINT ( 'NONE',  ( 157.4999999999998579, 70.78143705333094715, 45.00000000000000000 ) ) ;
#1237=DIRECTION ( 'NONE',  ( 0.8916010070299476009, 0.4528218681371110610, 0.000000000000000000 ) ) ;
#1243=ADVANCED_FACE ( 'NONE', ( #8010 ), #21077, .F. ) ;
#1245=EDGE_LOOP ( 'NONE', ( #25978, #17736, #1694, #18857 ) ) ;
#1246=CARTESIAN_POINT ( 'NONE',  ( 157.9999999999997726, 241.5708750675630370, 45.00000000000000000 ) ) ;
#1247=VERTEX_POINT ( 'NONE', #25391 ) ;
#1248=ORIENTED_EDGE ( 'NONE', *, *, #11493, .F. ) ;
#1253=AXIS2_PLACEMENT_3D ( 'NONE', #5028, #2731, #7342 ) ;
#1255=LINE ( 'NONE', #14202, #4246 ) ;
#1257=ADVANCED_FACE ( 'NONE', ( #23241 ), #3544, .F. ) ;
#1261=LINE ( 'NONE', #14075, #17692 ) ;
#1262=DIRECTION ( 'NONE',  ( -0.8916010070293584056, -0.4528218681382712996, 0.000000000000000000 ) ) ;
#1268=EDGE_CURVE ( 'NONE', #17639, #6857, #22211, .T. ) ;
#1276=CARTESIAN_POINT ( 'NONE',  ( 157.4999999999998579, 133.4783122410070462, 45.00000000000000000 ) ) ;
#1278=ORIENTED_EDGE ( 'NONE', *, *, #5594, .F. ) ;
#1280=ORIENTED_EDGE ( 'NONE', *, *, #8213, .T. ) ;
#1282=ORIENTED_EDGE ( 'NONE', *, *, #6019, .F. ) ;
#1287=VECTOR ( 'NONE', #11569, 1000.000000000000114 ) ;
#1290=LINE ( 'NONE', #16530, #20353 ) ;
#1293=LINE ( 'NONE', #10066, #1770 ) ;
#1298=LINE ( 'NONE', #23416, #27454 ) ;
#1299=DIRECTION ( 'NONE',  ( 0.4528218681383106015, 0.8916010070293384215, -0.000000000000000000 ) ) ;
#1301=EDGE_LOOP ( 'NONE', ( #17738, #10843, #12432, #22637 ) ) ;
#1307=EDGE_LOOP ( 'NONE', ( #3003, #20995, #26783, #10191 ) ) ;
#1313=VERTEX_POINT ( 'NONE', #10737 ) ;
#1314=ORIENTED_EDGE ( 'NONE', *, *, #22173, .F. ) ;
#1319=ORIENTED_EDGE ( 'NONE', *, *, #26487, .F. ) ;
#1322=ORIENTED_EDGE ( 'NONE', *, *, #21568, .T. ) ;
#1325=AXIS2_PLACEMENT_3D ( 'NONE', #11381, #2888, #5185 ) ;
#1327=FACE_OUTER_BOUND ( 'NONE', #26257, .T. ) ;
#1328=LINE ( 'NONE', #10097, #20457 ) ;
#1330=VECTOR ( 'NONE', #18427, 1000.000000000000000 ) ;
#1334=PLANE ( 'NONE',  #24695 ) ;
#1336=CARTESIAN_POINT ( 'NONE',  ( 158.0000000000010232, 106.1456246621830957, -45.00000000000000000 ) ) ;
#1337=DIRECTION ( 'NONE',  ( 0.000000000000000000, -1.000000000000000000, 0.000000000000000000 ) ) ;
#1338=ORIENTED_EDGE ( 'NONE', *, *, #20073, .T. ) ;
#1340=DIRECTION ( 'NONE',  ( -0.000000000000000000, -0.000000000000000000, -1.000000000000000000 ) ) ;
#1347=VERTEX_POINT ( 'NONE', #26229 ) ;
#1349=VECTOR ( 'NONE', #19200, 1000.000000000000000 ) ;
#1351=ORIENTED_EDGE ( 'NONE', *, *, #1668, .F. ) ;
#1353=CARTESIAN_POINT ( 'NONE',  ( 187.4999999999996305, 40.68693696324645970, 45.00000000000000000 ) ) ;
#1356=VERTEX_POINT ( 'NONE', #6560 ) ;
#1363=LINE ( 'NONE', #16328, #16208 ) ;
#1365=EDGE_CURVE ( 'NONE', #5280, #14759, #17614, .T. ) ;
#1367=DIRECTION ( 'NONE',  ( 0.8916010070295719014, -0.4528218681378510246, 0.000000000000000000 ) ) ;
#1370=DIRECTION ( 'NONE',  ( -0.000000000000000000, -0.000000000000000000, -1.000000000000000000 ) ) ;
#1371=CARTESIAN_POINT ( 'NONE',  ( 157.9999999999996305, 286.2047501951820436, 45.00000000000000000 ) ) ;
#1380=EDGE_CURVE ( 'NONE', #2545, #17167, #15192, .T. ) ;
#1382=DIRECTION ( 'NONE',  ( 0.8916010070300383061, -0.4528218681369324261, 0.000000000000000000 ) ) ;
#1384=LINE ( 'NONE', #10152, #19373 ) ;
#1387=VERTEX_POINT ( 'NONE', #28234 ) ;
#1392=ORIENTED_EDGE ( 'NONE', *, *, #17687, .F. ) ;
#1398=LINE ( 'NONE', #17195, #2292 ) ;
#1399=CARTESIAN_POINT ( 'NONE',  ( 157.4999999999998579, 191.1594374136689964, 45.00000000000000000 ) ) ;
#1400=EDGE_CURVE ( 'NONE', #16387, #24950, #26086, .T. ) ;
#1405=LINE ( 'NONE', #10177, #13351 ) ;
#1406=CARTESIAN_POINT ( 'NONE',  ( 158.0000000000007390, 135.7322497447605656, 45.00000000000000000 ) ) ;
#1410=EDGE_CURVE ( 'NONE', #13433, #14089, #4258, .T. ) ;
#1413=ORIENTED_EDGE ( 'NONE', *, *, #22527, .T. ) ;
#1420=VERTEX_POINT ( 'NONE', #16047 ) ;
#1424=VECTOR ( 'NONE', #10347, 1000.000000000000000 ) ;
#1428=EDGE_CURVE ( 'NONE', #11694, #24469, #24800, .T. ) ;
#1431=DIRECTION ( 'NONE',  ( -0.000000000000000000, -0.000000000000000000, -1.000000000000000000 ) ) ;
#1434=LINE ( 'NONE', #10346, #2698 ) ;
#1436=LINE ( 'NONE', #20978, #10652 ) ;
#1437=ORIENTED_EDGE ( 'NONE', *, *, #22794, .T. ) ;
#1438=VECTOR ( 'NONE', #8418, 1000.000000000000000 ) ;
#1441=EDGE_CURVE ( 'NONE', #27071, #21404, #16329, .T. ) ;
#1444=VERTEX_POINT ( 'NONE', #7129 ) ;
#1453=DIRECTION ( 'NONE',  ( 0.4528218681382713551, 0.8916010070293584056, -0.000000000000000000 ) ) ;
#1454=EDGE_CURVE ( 'NONE', #6404, #25224, #9712, .T. ) ;
#1455=VECTOR ( 'NONE', #19141, 1000.000000000000000 ) ;
#1456=DIRECTION ( 'NONE',  ( -0.000000000000000000, -0.000000000000000000, -1.000000000000000000 ) ) ;
#1458=ORIENTED_EDGE ( 'NONE', *, *, #9523, .F. ) ;
#1461=VECTOR ( 'NONE', #24885, 1000.000000000000000 ) ;
#1465=DIRECTION ( 'NONE',  ( 0.8916010070297547552, 0.4528218681374907018, 0.000000000000000000 ) ) ;
#1473=DIRECTION ( 'NONE',  ( 1.000000000000000000, -0.000000000000000000, -0.000000000000000000 ) ) ;
#1474=DIRECTION ( 'NONE',  ( -0.8916010070298258094, -0.4528218681373508137, 0.000000000000000000 ) ) ;
#1477=ORIENTED_EDGE ( 'NONE', *, *, #23081, .F. ) ;
#1480=VERTEX_POINT ( 'NONE', #7274 ) ;
#1483=DIRECTION ( 'NONE',  ( -0.000000000000000000, -0.000000000000000000, -1.000000000000000000 ) ) ;
#1489=ORIENTED_EDGE ( 'NONE', *, *, #27303, .F. ) ;
#1490=VECTOR ( 'NONE', #17807, 1000.000000000000000 ) ;
#1494=ORIENTED_EDGE ( 'NONE', *, *, #12522, .F. ) ;
#1496=ORIENTED_EDGE ( 'NONE', *, *, #26575, .T. ) ;
#1499=AXIS2_PLACEMENT_3D ( 'NONE', #7927, #16556, #3745 ) ;
#1500=LINE ( 'NONE', #14726, #16224 ) ;
#1502=VECTOR ( 'NONE', #13508, 1000.000000000000000 ) ;
#1503=CARTESIAN_POINT ( 'NONE',  ( 158.0000000000012506, 88.08262460212675649, 45.00000000000000000 ) ) ;
#1505=LINE ( 'NONE', #25358, #23863 ) ;
#1507=VECTOR ( 'NONE', #23226, 1000.000000000000000 ) ;
#1509=CARTESIAN_POINT ( 'NONE',  ( 157.4999999999998579, 158.5570623160774630, -45.00000000000000000 ) ) ;
#1511=LINE ( 'NONE', #14593, #11785 ) ;
#1512=LINE ( 'NONE', #3944, #4648 ) ;
#1517=DIRECTION ( 'NONE',  ( 0.4528218681383106015, 0.8916010070293384215, -0.000000000000000000 ) ) ;
#1521=ORIENTED_EDGE ( 'NONE', *, *, #20800, .F. ) ;
#1525=ORIENTED_EDGE ( 'NONE', *, *, #23009, .F. ) ;
#1526=ADVANCED_FACE ( 'NONE', ( #5388 ), #5107, .F. ) ;
#1531=LINE ( 'NONE', #10581, #12226 ) ;
#1533=EDGE_CURVE ( 'NONE', #27544, #6317, #524, .T. ) ;
#1534=VERTEX_POINT ( 'NONE', #14171 ) ;
#1537=DIRECTION ( 'NONE',  ( 0.8916010070296530587, 0.4528218681376912080, 0.000000000000000000 ) ) ;
#1539=EDGE_CURVE ( 'NONE', #18389, #14865, #22924, .T. ) ;
#1546=VECTOR ( 'NONE', #16501, 1000.000000000000000 ) ;
#1555=PLANE ( 'NONE',  #27926 ) ;
#1557=ORIENTED_EDGE ( 'NONE', *, *, #9327, .F. ) ;
#1558=ORIENTED_EDGE ( 'NONE', *, *, #24325, .F. ) ;
#1560=ORIENTED_EDGE ( 'NONE', *, *, #25133, .T. ) ;
#1561=ORIENTED_EDGE ( 'NONE', *, *, #19792, .F. ) ;
#1562=ORIENTED_EDGE ( 'NONE', *, *, #20866, .T. ) ;
#1566=VECTOR ( 'NONE', #4191, 1000.000000000000000 ) ;
#1568=VERTEX_POINT ( 'NONE', #14449 ) ;
#1573=CARTESIAN_POINT ( 'NONE',  ( 158.0000000000017337, 42.94087446699998623, 45.00000000000000000 ) ) ;
#1576=PLANE ( 'NONE',  #17380 ) ;
#1581=CARTESIAN_POINT ( 'NONE',  ( 158.0000000000004547, 165.8267498348450886, 45.00000000000000000 ) ) ;
#1584=ORIENTED_EDGE ( 'NONE', *, *, #16537, .F. ) ;
#1585=DIRECTION ( 'NONE',  ( -0.000000000000000000, -0.000000000000000000, -1.000000000000000000 ) ) ;
#1587=ORIENTED_EDGE ( 'NONE', *, *, #169, .F. ) ;
#1589=ORIENTED_EDGE ( 'NONE', *, *, #23458, .F. ) ;
#1591=DIRECTION ( 'NONE',  ( 0.4528218681372521703, 0.8916010070298759915, -0.000000000000000000 ) ) ;
#1592=DIRECTION ( 'NONE',  ( -0.8916010070294808632, -0.4528218681380302146, 0.000000000000000000 ) ) ;
#1593=ORIENTED_EDGE ( 'NONE', *, *, #22913, .T. ) ;
#1594=AXIS2_PLACEMENT_3D ( 'NONE', #11454, #27087, #16189 ) ;
#1597=CARTESIAN_POINT ( 'NONE',  ( 157.9999999999997726, 243.5708750675630370, -45.00000000000000000 ) ) ;
#1598=CARTESIAN_POINT ( 'NONE',  ( 157.4999999999998579, 65.76568703831686946, 45.00000000000000000 ) ) ;
#1599=DIRECTION ( 'NONE',  ( -0.8916010070297953893, -0.4528218681374107657, 0.000000000000000000 ) ) ;
#1602=VERTEX_POINT ( 'NONE', #25629 ) ;
#1605=EDGE_CURVE ( 'NONE', #1132, #25965, #23343, .T. ) ;
#1608=PLANE ( 'NONE',  #17319 ) ;
#1612=CARTESIAN_POINT ( 'NONE',  ( 158.0000000000014211, 71.03537455708449500, 45.00000000000000000 ) ) ;
#1614=PLANE ( 'NONE',  #24868 ) ;
#1615=LINE ( 'NONE', #19142, #16708 ) ;
#1626=PLANE ( 'NONE',  #24440 ) ;
#1627=VECTOR ( 'NONE', #17436, 1000.000000000000000 ) ;
#1628=EDGE_LOOP ( 'NONE', ( #28305, #27759, #13384, #15254 ) ) ;
#1633=LINE ( 'NONE', #10545, #15004 ) ;
#1637=VERTEX_POINT ( 'NONE', #23622 ) ;
#1638=AXIS2_PLACEMENT_3D ( 'NONE', #16135, #26603, #15998 ) ;
#1639=CARTESIAN_POINT ( 'NONE',  ( 157.9999999999996305, 281.6968751876750616, 45.00000000000000000 ) ) ;
#1640=EDGE_CURVE ( 'NONE', #13707, #5522, #3935, .T. ) ;
#1642=DIRECTION ( 'NONE',  ( 0.8916010070299374979, 0.4528218681371309895, 0.000000000000000000 ) ) ;
#1648=ORIENTED_EDGE ( 'NONE', *, *, #22288, .T. ) ;
#1652=CARTESIAN_POINT ( 'NONE',  ( 158.0000000000000853, 198.4291249324366504, -45.00000000000000000 ) ) ;
#1653=VERTEX_POINT ( 'NONE', #12442 ) ;
#1660=ORIENTED_EDGE ( 'NONE', *, *, #12229, .T. ) ;
#1663=ADVANCED_FACE ( 'NONE', ( #12583 ), #27911, .F. ) ;
#1665=ORIENTED_EDGE ( 'NONE', *, *, #26664, .F. ) ;
#1668=EDGE_CURVE ( 'NONE', #12610, #1602, #6094, .T. ) ;
#1670=VERTEX_POINT ( 'NONE', #14875 ) ;
#1671=FACE_OUTER_BOUND ( 'NONE', #20428, .T. ) ;
#1672=ORIENTED_EDGE ( 'NONE', *, *, #24020, .T. ) ;
#1681=DIRECTION ( 'NONE',  ( 0.8916010070297745171, -0.4528218681374519550, 0.000000000000000000 ) ) ;
#1684=DIRECTION ( 'NONE',  ( 1.000000000000000000, 0.000000000000000000, -0.000000000000000000 ) ) ;
#1685=CARTESIAN_POINT ( 'NONE',  ( 157.9999999999997442, 253.6023750975910502, -45.00000000000000000 ) ) ;
#1688=DIRECTION ( 'NONE',  ( -0.000000000000000000, -0.000000000000000000, -1.000000000000000000 ) ) ;
#1690=DIRECTION ( 'NONE',  ( 0.8916010070293283185, 0.4528218681383305855, 0.000000000000000000 ) ) ;
#1694=ORIENTED_EDGE ( 'NONE', *, *, #19190, .F. ) ;
#1698=ORIENTED_EDGE ( 'NONE', *, *, #3838, .T. ) ;
#1700=AXIS2_PLACEMENT_3D ( 'NONE', #16971, #14830, #16696 ) ;
#1702=CLOSED_SHELL ( 'NONE', ( #5037, #14678, #23234, #5502, #24283, #14938, #2265, #6554, #3871, #2199, #13933, #9365, #2896, #4437, #25882, #26524, #5267, #4378, #12675, #6374, #8968, #4779, #26328, #344, #6068, #9450, #12969, #18762, #20514, #6727, #1875, #10853, #18742, #5392, #13194, #12582, #19277, #18166, #19085, #10440, #18221, #18566, #25618, #12253, #14647, #10464, #17080, #19475, #15268, #9869, #23580, #6182, #21632, #24409, #1526, #6628, #10736, #19240, #3927, #7253, #24780, #18626, #19478, #24983, #23988, #16736, #15592, #10260, #23262, #15724, #26552, #13560, #22249, #180, #22593, #10691, #3798, #23786, #25039, #26910, #4809, #21961, #7831, #14753, #24354, #19010, #19761, #17454, #20021, #7354, #8581, #19145, #314, #2624, #8857, #25494, #939, #25019, #9129, #2966, #27152, #26925, #14259, #12894, #3707, #12651, #19439, #10937, #17272, #5615, #22983, #19660, #26651, #10955, #27873, #5324, #1915, #28026, #21153, #11826, #13205, #6460, #11114, #9036, #18486, #25249, #11745, #7152, #18596, #28329, #25125, #16182, #19441, #16215, #22230, #8313, #15900, #15073, #8508, #9344, #1243, #3247, #25582, #7338, #20421, #23414, #15097, #3922, #13722, #23619, #25027, #1178, #10674, #6214, #9098, #17169, #2398, #14100, #12721, #17965, #5525, #28323, #510, #15748, #26744, #9981, #6234, #23359, #13048, #1044, #6299, #224, #21750, #3083, #21148, #22875, #25886, #15159, #19007, #1057, #6980, #2584, #26022, #4016, #22674, #7351, #21783, #27274, #4794, #17226, #19758, #21928, #27153, #4612, #19467, #13247, #5694, #9082, #9434, #19499, #4868, #25515, #1257, #26488, #26113, #4151, #26822, #3805, #10457, #4468, #21309, #4634, #14273, #21906, #1016, #28194, #8459, #4106, #1109, #5454, #7777, #12803, #2308, #15557, #7607, #2112, #15237, #23165, #3246, #8094, #19637, #13237, #26392, #24327, #27246, #4082, #14612, #27495, #4346, #17624, #20076, #17132, #18759, #6232, #9507, #18288, #2132, #10414, #7489, #27770, #3054, #4015, #20011, #26666, #24896, #16228, #15401, #4271, #21454, #2267, #6874, #23913, #8462, #15657, #3665, #23687, #14364, #4337, #24772, #22826, #21896, #3302, #22051, #25792, #27461, #16196, #17007, #744, #25723, #17686, #20797, #16970, #1663, #24481, #27557, #6400, #25152, #23760, #16430, #25953, #7550, #12743, #21257, #9536, #28213, #16597, #25935, #5106, #24730, #5420, #4153, #2602, #18380, #9162, #15369, #14626 ) ) ;
#1703=ORIENTED_EDGE ( 'NONE', *, *, #14809, .T. ) ;
#1705=ORIENTED_EDGE ( 'NONE', *, *, #12376, .F. ) ;
#1706=DIRECTION ( 'NONE',  ( 0.8916010070295207202, -0.4528218681379515553, 0.000000000000000000 ) ) ;
#1709=DIRECTION ( 'NONE',  ( 0.8916010070293584056, -0.4528218681382712996, 0.000000000000000000 ) ) ;
#1724=EDGE_LOOP ( 'NONE', ( #4109, #22118, #13477, #16625 ) ) ;
#1726=ORIENTED_EDGE ( 'NONE', *, *, #608, .T. ) ;
#1738=EDGE_LOOP ( 'NONE', ( #12101, #20635, #18877, #24759 ) ) ;
#1740=VECTOR ( 'NONE', #966, 1000.000000000000000 ) ;
#1741=CARTESIAN_POINT ( 'NONE',  ( 158.0000000000010232, 106.1456246621830957, -45.00000000000000000 ) ) ;
#1744=VECTOR ( 'NONE', #26376, 1000.000000000000000 ) ;
#1747=CARTESIAN_POINT ( 'NONE',  ( 157.4999999999998579, 78.30506207585207790, 45.00000000000000000 ) ) ;
#1749=CARTESIAN_POINT ( 'NONE',  ( 157.4999999999998295, 228.7775625262745223, -45.00000000000000000 ) ) ;
#1755=DIRECTION ( 'NONE',  ( 0.8916010070294395629, -0.4528218681381114274, 0.000000000000000000 ) ) ;
#1757=ORIENTED_EDGE ( 'NONE', *, *, #20832, .T. ) ;
#1759=FACE_OUTER_BOUND ( 'NONE', #21101, .T. ) ;
#1760=ORIENTED_EDGE ( 'NONE', *, *, #5776, .F. ) ;
#1761=EDGE_CURVE ( 'NONE', #21329, #13313, #21888, .T. ) ;
#1769=VECTOR ( 'NONE', #4087, 1000.000000000000000 ) ;
#1770=VECTOR ( 'NONE', #27706, 1000.000000000000000 ) ;
#1771=ORIENTED_EDGE ( 'NONE', *, *, #23602, .T. ) ;
#1776=PLANE ( 'NONE',  #8728 ) ;
#1778=CARTESIAN_POINT ( 'NONE',  ( 157.4999999999997726, 246.3326875788235384, -45.00000000000000000 ) ) ;
#1779=EDGE_CURVE ( 'NONE', #9971, #24116, #6235, .T. ) ;
#1781=ORIENTED_EDGE ( 'NONE', *, *, #17710, .F. ) ;
#1783=LINE ( 'NONE', #3806, #16806 ) ;
#1786=CARTESIAN_POINT ( 'NONE',  ( 157.4999999999998579, 196.1751874286831026, 45.00000000000000000 ) ) ;
#1787=DIRECTION ( 'NONE',  ( -0.8916010070293383105, -0.4528218681383106015, 0.000000000000000000 ) ) ;
#1793=PLANE ( 'NONE',  #9859 ) ;
#1795=VERTEX_POINT ( 'NONE', #17718 ) ;
#1796=VECTOR ( 'NONE', #3292, 1000.000000000000000 ) ;
#1797=EDGE_CURVE ( 'NONE', #18321, #16168, #19453, .T. ) ;
#1798=LINE ( 'NONE', #17313, #12537 ) ;
#1801=CARTESIAN_POINT ( 'NONE',  ( 157.9999999999997726, 243.5708750675630370, 45.00000000000000000 ) ) ;
#1805=VECTOR ( 'NONE', #9490, 1000.000000000000114 ) ;
#1806=VECTOR ( 'NONE', #25098, 1000.000000000000000 ) ;
#1813=VECTOR ( 'NONE', #24340, 1000.000000000000114 ) ;
#1823=DIRECTION ( 'NONE',  ( -0.8916010070293584056, 0.4528218681382713551, 0.000000000000000000 ) ) ;
#1825=DIRECTION ( 'NONE',  ( 0.8916010070293584056, -0.4528218681382712996, 0.000000000000000000 ) ) ;
#1827=VECTOR ( 'NONE', #25631, 1000.000000000000000 ) ;
#1828=CARTESIAN_POINT ( 'NONE',  ( 158.0000000000011937, 93.09837461714084839, -45.00000000000000000 ) ) ;
#1829=DIRECTION ( 'NONE',  ( -0.8916010070296936929, -0.4528218681376112165, 0.000000000000000000 ) ) ;
#1830=CARTESIAN_POINT ( 'NONE',  ( 157.9999999999996874, 266.6496251426330559, 45.00000000000000000 ) ) ;
#1835=ORIENTED_EDGE ( 'NONE', *, *, #7098, .T. ) ;
#1836=ORIENTED_EDGE ( 'NONE', *, *, #4245, .T. ) ;
#1837=ORIENTED_EDGE ( 'NONE', *, *, #8083, .F. ) ;
#1839=EDGE_LOOP ( 'NONE', ( #24486, #23427, #15466, #10507 ) ) ;
#1841=DIRECTION ( 'NONE',  ( 0.000000000000000000, -1.000000000000000000, 0.000000000000000000 ) ) ;
#1845=DIRECTION ( 'NONE',  ( 0.4528218681377511601, 0.8916010070296226386, -0.000000000000000000 ) ) ;
#1847=AXIS2_PLACEMENT_3D ( 'NONE', #23597, #26024, #27887 ) ;
#1850=CARTESIAN_POINT ( 'NONE',  ( 158.0000000000003411, 175.8582498648732440, 45.00000000000000000 ) ) ;
#1857=ORIENTED_EDGE ( 'NONE', *, *, #15799, .T. ) ;
#1860=DIRECTION ( 'NONE',  ( -0.8916010070293783896, 0.4528218681382319422, 0.000000000000000000 ) ) ;
#1864=ORIENTED_EDGE ( 'NONE', *, *, #11211, .F. ) ;
#1867=EDGE_CURVE ( 'NONE', #20330, #25368, #19872, .T. ) ;
#1873=FACE_OUTER_BOUND ( 'NONE', #25346, .T. ) ;
#1874=VERTEX_POINT ( 'NONE', #13418 ) ;
#1875=ADVANCED_FACE ( 'NONE', ( #345 ), #14134, .F. ) ;
#1880=EDGE_CURVE ( 'NONE', #16325, #26049, #22463, .T. ) ;
#1881=VECTOR ( 'NONE', #15054, 1000.000000000000000 ) ;
#1883=DIRECTION ( 'NONE',  ( -0.8916010070299268397, 0.4528218681371523058, 0.000000000000000000 ) ) ;
#1886=CARTESIAN_POINT ( 'NONE',  ( 157.4999999999996589, 281.4429376839215138, -45.00000000000000000 ) ) ;
#1888=EDGE_LOOP ( 'NONE', ( #7302, #12887 ) ) ;
#1890=LINE ( 'NONE', #24028, #11986 ) ;
#1891=LINE ( 'NONE', #10668, #22112 ) ;
#1893=ORIENTED_EDGE ( 'NONE', *, *, #17759, .T. ) ;
#1894=LINE ( 'NONE', #19851, #17393 ) ;
#1898=ORIENTED_EDGE ( 'NONE', *, *, #11888, .T. ) ;
#1900=DIRECTION ( 'NONE',  ( -0.000000000000000000, -0.000000000000000000, -1.000000000000000000 ) ) ;
#1902=AXIS2_PLACEMENT_3D ( 'NONE', #7946, #10109, #6209 ) ;
#1905=VERTEX_POINT ( 'NONE', #22318 ) ;
#1906=VECTOR ( 'NONE', #23751, 1000.000000000000000 ) ;
#1908=VERTEX_POINT ( 'NONE', #16150 ) ;
#1911=EDGE_CURVE ( 'NONE', #10196, #24950, #3053, .T. ) ;
#1915=ADVANCED_FACE ( 'NONE', ( #908 ), #24473, .F. ) ;
#1917=LINE ( 'NONE', #10698, #3383 ) ;
#1922=ORIENTED_EDGE ( 'NONE', *, *, #27086, .T. ) ;
#1925=CARTESIAN_POINT ( 'NONE',  ( 157.4999999999998579, 123.4468122109788482, 45.00000000000000000 ) ) ;
#1926=VECTOR ( 'NONE', #10361, 1000.000000000000000 ) ;
#1928=CARTESIAN_POINT ( 'NONE',  ( 157.9999999999999147, 213.9842499849850697, -45.00000000000000000 ) ) ;
#1933=CARTESIAN_POINT ( 'NONE',  ( 157.4999999999998579, 65.76568703831686946, 45.00000000000000000 ) ) ;
#1934=CARTESIAN_POINT ( 'NONE',  ( 158.0000000000002558, 183.3818748873943889, -45.00000000000000000 ) ) ;
#1935=CARTESIAN_POINT ( 'NONE',  ( 157.4999999999998010, 241.3169375638095460, 45.00000000000000000 ) ) ;
#1938=ORIENTED_EDGE ( 'NONE', *, *, #7675, .F. ) ;
#1942=ORIENTED_EDGE ( 'NONE', *, *, #3569, .F. ) ;
#1943=VERTEX_POINT ( 'NONE', #4921 ) ;
#1949=ORIENTED_EDGE ( 'NONE', *, *, #2985, .F. ) ;
#1952=LINE ( 'NONE', #12471, #4085 ) ;
#1953=DIRECTION ( 'NONE',  ( -0.8916010070296124246, 0.4528218681377710886, 0.000000000000000000 ) ) ;
#1956=DIRECTION ( 'NONE',  ( -0.000000000000000000, 0.000000000000000000, -1.000000000000000000 ) ) ;
#1960=EDGE_CURVE ( 'NONE', #19398, #28117, #22608, .T. ) ;
#1963=DIRECTION ( 'NONE',  ( -0.8916010070299875689, 0.4528218681370324017, 0.000000000000000000 ) ) ;
#1965=PLANE ( 'NONE',  #18741 ) ;
#1968=VECTOR ( 'NONE', #7525, 1000.000000000000000 ) ;
#1970=CARTESIAN_POINT ( 'NONE',  ( 158.0000000000009663, 113.1613746771971876, 45.00000000000000000 ) ) ;
#1975=EDGE_CURVE ( 'NONE', #3327, #9386, #24902, .T. ) ;
#1979=ORIENTED_EDGE ( 'NONE', *, *, #26840, .T. ) ;
#1981=VERTEX_POINT ( 'NONE', #9398 ) ;
#1982=VERTEX_POINT ( 'NONE', #20445 ) ;
#1983=ORIENTED_EDGE ( 'NONE', *, *, #10135, .F. ) ;
#1985=ORIENTED_EDGE ( 'NONE', *, *, #28042, .T. ) ;
#1986=VECTOR ( 'NONE', #24400, 1000.000000000000000 ) ;
#1987=CARTESIAN_POINT ( 'NONE',  ( 158.0000000000001705, 190.9054999099155054, 45.00000000000000000 ) ) ;
#1989=DIRECTION ( 'NONE',  ( 0.8916010070293383105, -0.4528218681383106015, 0.000000000000000000 ) ) ;
#1996=EDGE_CURVE ( 'NONE', #19047, #23530, #18298, .T. ) ;
#1998=LINE ( 'NONE', #8899, #22392 ) ;
#1999=DIRECTION ( 'NONE',  ( 1.000000000000000000, 0.000000000000000000, -0.000000000000000000 ) ) ;
#2006=VECTOR ( 'NONE', #26913, 1000.000000000000227 ) ;
#2011=VECTOR ( 'NONE', #1337, 1000.000000000000000 ) ;
#2015=EDGE_CURVE ( 'NONE', #21206, #27854, #20721, .T. ) ;
#2017=PLANE ( 'NONE',  #8080 ) ;
#2022=LINE ( 'NONE', #10798, #27634 ) ;
#2023=VECTOR ( 'NONE', #1142, 1000.000000000000000 ) ;
#2025=ORIENTED_EDGE ( 'NONE', *, *, #1880, .T. ) ;
#2029=DIRECTION ( 'NONE',  ( 0.000000000000000000, -1.000000000000000000, 0.000000000000000000 ) ) ;
#2034=ORIENTED_EDGE ( 'NONE', *, *, #19694, .T. ) ;
#2036=FACE_OUTER_BOUND ( 'NONE', #4668, .T. ) ;
#2039=ORIENTED_EDGE ( 'NONE', *, *, #19310, .F. ) ;
#2047=EDGE_CURVE ( 'NONE', #13726, #5026, #18575, .T. ) ;
#2048=CARTESIAN_POINT ( 'NONE',  ( 157.4999999999998579, 193.6673124211760353, 45.00000000000000000 ) ) ;
#2051=ORIENTED_EDGE ( 'NONE', *, *, #11624, .T. ) ;
#2053=ORIENTED_EDGE ( 'NONE', *, *, #2765, .T. ) ;
#2054=FACE_OUTER_BOUND ( 'NONE', #7891, .T. ) ;
#2067=EDGE_LOOP ( 'NONE', ( #1560, #12873, #23006, #5591 ) ) ;
#2072=DIRECTION ( 'NONE',  ( 0.000000000000000000, -1.000000000000000000, 0.000000000000000000 ) ) ;
#2077=DIRECTION ( 'NONE',  ( -0.8916010070293384215, 0.4528218681383106015, 0.000000000000000000 ) ) ;
#2078=DIRECTION ( 'NONE',  ( 0.8916010070294199119, 0.4528218681381501742, 0.000000000000000000 ) ) ;
#2079=DIRECTION ( 'NONE',  ( 0.4528218681381700472, -0.8916010070294099199, 0.000000000000000000 ) ) ;
#2081=VERTEX_POINT ( 'NONE', #23305 ) ;
#2086=DIRECTION ( 'NONE',  ( 0.000000000000000000, -1.000000000000000000, 0.000000000000000000 ) ) ;
#2087=EDGE_LOOP ( 'NONE', ( #4456, #24594, #552, #27769 ) ) ;
#2088=AXIS2_PLACEMENT_3D ( 'NONE', #6259, #23790, #2363 ) ;
#2093=ORIENTED_EDGE ( 'NONE', *, *, #23944, .T. ) ;
#2097=DIRECTION ( 'NONE',  ( -0.8916010070294605461, -0.4528218681380702382, 0.000000000000000000 ) ) ;
#2099=PLANE ( 'NONE',  #25254 ) ;
#2102=FACE_OUTER_BOUND ( 'NONE', #2087, .T. ) ;
#2105=EDGE_CURVE ( 'NONE', #6230, #3625, #10237, .T. ) ;
#2107=FACE_OUTER_BOUND ( 'NONE', #26223, .T. ) ;
#2109=VECTOR ( 'NONE', #6827, 1000.000000000000227 ) ;
#2110=EDGE_LOOP ( 'NONE', ( #12716, #23879, #5558, #10573 ) ) ;
#2111=DIRECTION ( 'NONE',  ( -0.000000000000000000, 0.000000000000000000, -1.000000000000000000 ) ) ;
#2112=ADVANCED_FACE ( 'NONE', ( #4297 ), #26126, .F. ) ;
#2113=LINE ( 'NONE', #10750, #15570 ) ;
#2115=AXIS2_PLACEMENT_3D ( 'NONE', #26238, #17621, #22363 ) ;
#2119=VERTEX_POINT ( 'NONE', #14274 ) ;
#2123=VERTEX_POINT ( 'NONE', #12124 ) ;
#2124=EDGE_CURVE ( 'NONE', #22290, #17151, #18849, .T. ) ;
#2125=ORIENTED_EDGE ( 'NONE', *, *, #4425, .T. ) ;
#2131=CARTESIAN_POINT ( 'NONE',  ( 157.9999999999996589, 279.1890001801680796, 45.00000000000000000 ) ) ;
#2132=ADVANCED_FACE ( 'NONE', ( #28272 ), #7797, .F. ) ;
#2134=DIRECTION ( 'NONE',  ( -0.000000000000000000, -0.000000000000000000, -1.000000000000000000 ) ) ;
#2138=DIRECTION ( 'NONE',  ( 0.4528218681382319422, 0.8916010070293783896, -0.000000000000000000 ) ) ;
#2146=EDGE_LOOP ( 'NONE', ( #5903, #27907, #19160, #4136 ) ) ;
#2147=AXIS2_PLACEMENT_3D ( 'NONE', #7925, #1177, #18702 ) ;
#2149=DIRECTION ( 'NONE',  ( 0.8916010070296733758, -0.4528218681376511845, 0.000000000000000000 ) ) ;
#2150=ORIENTED_EDGE ( 'NONE', *, *, #26551, .F. ) ;
#2157=FACE_OUTER_BOUND ( 'NONE', #3072, .T. ) ;
#2161=ORIENTED_EDGE ( 'NONE', *, *, #12174, .T. ) ;
#2163=ORIENTED_EDGE ( 'NONE', *, *, #23541, .F. ) ;
#2164=AXIS2_PLACEMENT_3D ( 'NONE', #17497, #17357, #21675 ) ;
#2165=LINE ( 'NONE', #20122, #16244 ) ;
#2167=LINE ( 'NONE', #25, #5708 ) ;
#2169=EDGE_CURVE ( 'NONE', #27071, #14580, #10770, .T. ) ;
#2176=ORIENTED_EDGE ( 'NONE', *, *, #8706, .F. ) ;
#2177=CARTESIAN_POINT ( 'NONE',  ( 157.4999999999998579, 45.70268697826052318, 45.00000000000000000 ) ) ;
#2185=ORIENTED_EDGE ( 'NONE', *, *, #19938, .F. ) ;
#2186=ORIENTED_EDGE ( 'NONE', *, *, #278, .T. ) ;
#2188=PLANE ( 'NONE',  #12575 ) ;
#2190=EDGE_LOOP ( 'NONE', ( #11825, #16793, #16024, #14263 ) ) ;
#2197=EDGE_CURVE ( 'NONE', #4442, #24279, #18091, .T. ) ;
#2199=ADVANCED_FACE ( 'NONE', ( #24548 ), #17791, .F. ) ;
#2202=EDGE_LOOP ( 'NONE', ( #8838, #14033, #21840, #5413 ) ) ;
#2205=DIRECTION ( 'NONE',  ( 0.4528218681382519262, -0.8916010070293682865, 0.000000000000000000 ) ) ;
#2208=PLANE ( 'NONE',  #21967 ) ;
#2209=VECTOR ( 'NONE', #5749, 1000.000000000000000 ) ;
#2212=CARTESIAN_POINT ( 'NONE',  ( 157.4999999999996305, 283.9508126914284958, -45.00000000000000000 ) ) ;
#2213=DIRECTION ( 'NONE',  ( 0.8916010070294098089, 0.4528218681381699917, 0.000000000000000000 ) ) ;
#2215=ORIENTED_EDGE ( 'NONE', *, *, #16315, .T. ) ;
#2219=EDGE_CURVE ( 'NONE', #5556, #2475, #2413, .T. ) ;
#2221=VECTOR ( 'NONE', #20588, 1000.000000000000000 ) ;
#2222=ORIENTED_EDGE ( 'NONE', *, *, #8741, .F. ) ;
#2223=ORIENTED_EDGE ( 'NONE', *, *, #794, .T. ) ;
#2225=EDGE_CURVE ( 'NONE', #26896, #21202, #2272, .T. ) ;
#2233=DIRECTION ( 'NONE',  ( -0.8916010070295112833, -0.4528218681379702626, 0.000000000000000000 ) ) ;
#2238=PLANE ( 'NONE',  #28064 ) ;
#2240=CARTESIAN_POINT ( 'NONE',  ( 157.4999999999998579, 138.4940622560211239, -45.00000000000000000 ) ) ;
#2241=CARTESIAN_POINT ( 'NONE',  ( 157.4999999999998579, 183.6358123911478799, 45.00000000000000000 ) ) ;
#2243=CARTESIAN_POINT ( 'NONE',  ( 158.0000000000008527, 125.7007497147323818, 45.00000000000000000 ) ) ;
#2244=LINE ( 'NONE', #11027, #18518 ) ;
#2250=DIRECTION ( 'NONE',  ( 1.000000000000000000, 0.000000000000000000, -0.000000000000000000 ) ) ;
#2252=ORIENTED_EDGE ( 'NONE', *, *, #26243, .F. ) ;
#2253=VECTOR ( 'NONE', #12899, 1000.000000000000000 ) ;
#2256=ORIENTED_EDGE ( 'NONE', *, *, #24363, .F. ) ;
#2259=ORIENTED_EDGE ( 'NONE', *, *, #19337, .T. ) ;
#2261=ORIENTED_EDGE ( 'NONE', *, *, #16658, .F. ) ;
#2265=ADVANCED_FACE ( 'NONE', ( #4714 ), #281, .F. ) ;
#2267=ADVANCED_FACE ( 'NONE', ( #22248 ), #19806, .F. ) ;
#2271=CARTESIAN_POINT ( 'NONE',  ( 157.4999999999998579, 153.5413123010633853, 45.00000000000000000 ) ) ;
#2272=LINE ( 'NONE', #11196, #26887 ) ;
#2273=VECTOR ( 'NONE', #1585, 1000.000000000000000 ) ;
#2275=LINE ( 'NONE', #24263, #2562 ) ;
#2277=LINE ( 'NONE', #25988, #14141 ) ;
#2282=CARTESIAN_POINT ( 'NONE',  ( 158.0000000000004263, 166.3346248423521274, 45.00000000000000000 ) ) ;
#2283=LINE ( 'NONE', #19815, #21231 ) ;
#2284=ORIENTED_EDGE ( 'NONE', *, *, #18083, .F. ) ;
#2287=DIRECTION ( 'NONE',  ( 0.8916010070299267287, -0.4528218681371523058, 0.000000000000000000 ) ) ;
#2289=ORIENTED_EDGE ( 'NONE', *, *, #14950, .T. ) ;
#2292=VECTOR ( 'NONE', #21360, 1000.000000000000000 ) ;
#2293=FACE_OUTER_BOUND ( 'NONE', #20733, .T. ) ;
#2297=EDGE_CURVE ( 'NONE', #6857, #21241, #564, .T. ) ;
#2300=ORIENTED_EDGE ( 'NONE', *, *, #5170, .T. ) ;
#2305=VERTEX_POINT ( 'NONE', #9328 ) ;
#2308=ADVANCED_FACE ( 'NONE', ( #4431 ), #13217, .F. ) ;
#2309=DIRECTION ( 'NONE',  ( 0.8916010070297643031, -0.4528218681374719945, 0.000000000000000000 ) ) ;
#2312=CARTESIAN_POINT ( 'NONE',  ( 158.0000000000016485, 48.46449948952110987, 45.00000000000000000 ) ) ;
#2314=ORIENTED_EDGE ( 'NONE', *, *, #16923, .F. ) ;
#2315=DIRECTION ( 'NONE',  ( -0.8916010070298258094, -0.4528218681373508137, 0.000000000000000000 ) ) ;
#2320=DIRECTION ( 'NONE',  ( 0.000000000000000000, 0.000000000000000000, 1.000000000000000000 ) ) ;
#2323=EDGE_CURVE ( 'NONE', #4885, #25224, #1261, .T. ) ;
#2326=VERTEX_POINT ( 'NONE', #7598 ) ;
#2334=CARTESIAN_POINT ( 'NONE',  ( 158.0000000000006821, 138.7479997597746433, 45.00000000000000000 ) ) ;
#2335=VECTOR ( 'NONE', #10779, 1000.000000000000000 ) ;
#2337=LINE ( 'NONE', #20160, #8911 ) ;
#2338=LINE ( 'NONE', #11118, #10822 ) ;
#2339=DIRECTION ( 'NONE',  ( 1.000000000000000000, 0.000000000000000000, -0.000000000000000000 ) ) ;
#2341=DIRECTION ( 'NONE',  ( 0.8916010070293409751, 0.4528218681383056610, 0.000000000000000000 ) ) ;
#2344=DIRECTION ( 'NONE',  ( -0.8916010070294808632, -0.4528218681380302146, 0.000000000000000000 ) ) ;
#2348=ORIENTED_EDGE ( 'NONE', *, *, #21810, .T. ) ;
#2349=PLANE ( 'NONE',  #8686 ) ;
#2350=ORIENTED_EDGE ( 'NONE', *, *, #20216, .T. ) ;
#2352=PLANE ( 'NONE',  #12553 ) ;
#2356=DIRECTION ( 'NONE',  ( -0.000000000000000000, -0.000000000000000000, -1.000000000000000000 ) ) ;
#2361=LINE ( 'NONE', #22199, #26753 ) ;
#2362=ORIENTED_EDGE ( 'NONE', *, *, #6195, .F. ) ;
#2363=DIRECTION ( 'NONE',  ( 0.8916010070293384215, 0.4528218681383106015, 0.000000000000000000 ) ) ;
#2367=EDGE_CURVE ( 'NONE', #19053, #19430, #18514, .T. ) ;
#2368=CARTESIAN_POINT ( 'NONE',  ( 157.9999999999996589, 281.1890001801680796, 45.00000000000000000 ) ) ;
#2369=EDGE_CURVE ( 'NONE', #4844, #19307, #27531, .T. ) ;
#2371=VERTEX_POINT ( 'NONE', #12057 ) ;
#2375=CARTESIAN_POINT ( 'NONE',  ( 158.0000000000003695, 173.3503748573662051, 45.00000000000000000 ) ) ;
#2376=CARTESIAN_POINT ( 'NONE',  ( 158.0000000000003979, 168.8424998498591663, 45.00000000000000000 ) ) ;
#2380=CARTESIAN_POINT ( 'NONE',  ( 157.4999999999998579, 130.9704372334999789, 45.00000000000000000 ) ) ;
#2382=PLANE ( 'NONE',  #4391 ) ;
#2383=LINE ( 'NONE', #390, #12473 ) ;
#2384=FACE_OUTER_BOUND ( 'NONE', #23508, .T. ) ;
#2387=FACE_OUTER_BOUND ( 'NONE', #11764, .T. ) ;
#2388=CARTESIAN_POINT ( 'NONE',  ( 158.0000000000008527, 125.7007497147323818, -45.00000000000000000 ) ) ;
#2394=CARTESIAN_POINT ( 'NONE',  ( 158.0000000000008242, 126.2086247222394206, 45.00000000000000000 ) ) ;
#2395=ORIENTED_EDGE ( 'NONE', *, *, #3174, .F. ) ;
#2398=ADVANCED_FACE ( 'NONE', ( #16503 ), #5572, .F. ) ;
#2399=AXIS2_PLACEMENT_3D ( 'NONE', #6474, #4591, #17246 ) ;
#2400=ORIENTED_EDGE ( 'NONE', *, *, #10977, .F. ) ;
#2405=VERTEX_POINT ( 'NONE', #6138 ) ;
#2407=CARTESIAN_POINT ( 'NONE',  ( 158.0000000000016485, 48.46449948952110987, 45.00000000000000000 ) ) ;
#2408=PLANE ( 'NONE',  #18350 ) ;
#2413=LINE ( 'NONE', #11053, #273 ) ;
#2415=DIRECTION ( 'NONE',  ( 0.8916010070297439860, -0.4528218681375119070, 0.000000000000000000 ) ) ;
#2418=CARTESIAN_POINT ( 'NONE',  ( 157.4999999999998010, 238.8090625563025071, 45.00000000000000000 ) ) ;
#2420=AXIS2_PLACEMENT_3D ( 'NONE', #16589, #18182, #27211 ) ;
#2422=FACE_OUTER_BOUND ( 'NONE', #26292, .T. ) ;
#2423=CARTESIAN_POINT ( 'NONE',  ( 157.4999999999998579, 163.5728123310915407, -45.00000000000000000 ) ) ;
#2430=PLANE ( 'NONE',  #21216 ) ;
#2432=EDGE_LOOP ( 'NONE', ( #11207, #2400, #2694, #11717 ) ) ;
#2433=ORIENTED_EDGE ( 'NONE', *, *, #21835, .T. ) ;
#2437=VECTOR ( 'NONE', #18315, 1000.000000000000000 ) ;
#2440=EDGE_CURVE ( 'NONE', #13140, #21319, #25669, .T. ) ;
#2441=ORIENTED_EDGE ( 'NONE', *, *, #26628, .T. ) ;
#2444=DIRECTION ( 'NONE',  ( 0.8916010070298759915, -0.4528218681372521703, 0.000000000000000000 ) ) ;
#2451=ORIENTED_EDGE ( 'NONE', *, *, #8729, .F. ) ;
#2452=FACE_OUTER_BOUND ( 'NONE', #26418, .T. ) ;
#2455=LINE ( 'NONE', #11241, #12022 ) ;
#2458=EDGE_LOOP ( 'NONE', ( #3140, #24563, #17382, #22591 ) ) ;
#2459=DIRECTION ( 'NONE',  ( -0.000000000000000000, -0.000000000000000000, -1.000000000000000000 ) ) ;
#2466=LINE ( 'NONE', #11255, #21190 ) ;
#2468=VERTEX_POINT ( 'NONE', #11311 ) ;
#2473=CARTESIAN_POINT ( 'NONE',  ( 157.4999999999998579, 48.21056198576756202, 45.00000000000000000 ) ) ;
#2474=ORIENTED_EDGE ( 'NONE', *, *, #4505, .T. ) ;
#2475=VERTEX_POINT ( 'NONE', #2380 ) ;
#2479=LINE ( 'NONE', #24618, #2006 ) ;
#2481=CARTESIAN_POINT ( 'NONE',  ( 157.4999999999998579, 148.5255622860493077, 45.00000000000000000 ) ) ;
#2482=EDGE_CURVE ( 'NONE', #7477, #12854, #26372, .T. ) ;
#2483=PLANE ( 'NONE',  #10574 ) ;
#2485=VERTEX_POINT ( 'NONE', #11160 ) ;
#2487=DIRECTION ( 'NONE',  ( -0.8916010070293711731, 0.4528218681382463751, 0.000000000000000000 ) ) ;
#2489=LINE ( 'NONE', #355, #13034 ) ;
#2492=PLANE ( 'NONE',  #18775 ) ;
#2499=LINE ( 'NONE', #11289, #12946 ) ;
#2500=VECTOR ( 'NONE', #3983, 1000.000000000000114 ) ;
#2503=ORIENTED_EDGE ( 'NONE', *, *, #5389, .T. ) ;
#2505=EDGE_LOOP ( 'NONE', ( #25413, #21714, #11992, #1413 ) ) ;
#2506=ORIENTED_EDGE ( 'NONE', *, *, #14809, .F. ) ;
#2511=ORIENTED_EDGE ( 'NONE', *, *, #17869, .T. ) ;
#2512=ORIENTED_EDGE ( 'NONE', *, *, #21278, .F. ) ;
#2516=CARTESIAN_POINT ( 'NONE',  ( 158.0000000000003695, 171.3503748573662051, 45.00000000000000000 ) ) ;
#2518=EDGE_CURVE ( 'NONE', #4042, #12076, #28372, .T. ) ;
#2520=CARTESIAN_POINT ( 'NONE',  ( 158.0000000000005684, 151.2873747973098659, 45.00000000000000000 ) ) ;
#2522=LINE ( 'NONE', #20055, #15925 ) ;
#2523=CARTESIAN_POINT ( 'NONE',  ( 158.0000000000004547, 163.8267498348450886, -45.00000000000000000 ) ) ;
#2524=DIRECTION ( 'NONE',  ( -0.000000000000000000, -0.000000000000000000, -1.000000000000000000 ) ) ;
#2526=LINE ( 'NONE', #11317, #4741 ) ;
#2529=DIRECTION ( 'NONE',  ( -0.000000000000000000, 0.000000000000000000, -1.000000000000000000 ) ) ;
#2531=DIRECTION ( 'NONE',  ( 0.8916010070295316003, 0.4528218681379303501, 0.000000000000000000 ) ) ;
#2535=PLANE ( 'NONE',  #5122 ) ;
#2538=VECTOR ( 'NONE', #14754, 1000.000000000000000 ) ;
#2539=DIRECTION ( 'NONE',  ( -0.8916010070293783896, 0.4528218681382319422, 0.000000000000000000 ) ) ;
#2540=ORIENTED_EDGE ( 'NONE', *, *, #25553, .F. ) ;
#2541=PLANE ( 'NONE',  #19229 ) ;
#2544=ORIENTED_EDGE ( 'NONE', *, *, #9974, .F. ) ;
#2545=VERTEX_POINT ( 'NONE', #11021 ) ;
#2546=EDGE_CURVE ( 'NONE', #17690, #17812, #22215, .T. ) ;
#2547=ORIENTED_EDGE ( 'NONE', *, *, #10246, .T. ) ;
#2548=VERTEX_POINT ( 'NONE', #2520 ) ;
#2551=CARTESIAN_POINT ( 'NONE',  ( 157.4999999999997726, 246.3326875788235384, -45.00000000000000000 ) ) ;
#2552=CARTESIAN_POINT ( 'NONE',  ( 158.0000000000009948, 110.6534996696901345, 45.00000000000000000 ) ) ;
#2553=VECTOR ( 'NONE', #18994, 1000.000000000000227 ) ;
#2555=AXIS2_PLACEMENT_3D ( 'NONE', #17000, #3360, #27765 ) ;
#2559=CARTESIAN_POINT ( 'NONE',  ( 157.4999999999998579, 75.79718706834503905, 45.00000000000000000 ) ) ;
#2561=DIRECTION ( 'NONE',  ( 0.8916010070293383105, -0.4528218681383106015, 0.000000000000000000 ) ) ;
#2562=VECTOR ( 'NONE', #2415, 1000.000000000000227 ) ;
#2568=CARTESIAN_POINT ( 'NONE',  ( 157.4999999999998579, 70.78143705333094715, -45.00000000000000000 ) ) ;
#2569=CARTESIAN_POINT ( 'NONE',  ( 157.9999999999998863, 218.4921249924925348, 45.00000000000000000 ) ) ;
#2579=EDGE_LOOP ( 'NONE', ( #9769, #6866, #219 ) ) ;
#2581=ORIENTED_EDGE ( 'NONE', *, *, #25702, .T. ) ;
#2582=CARTESIAN_POINT ( 'NONE',  ( 158.0000000000011653, 95.60624962464788723, 45.00000000000000000 ) ) ;
#2583=DIRECTION ( 'NONE',  ( 0.8916010070293584056, -0.4528218681382712996, 0.000000000000000000 ) ) ;
#2584=ADVANCED_FACE ( 'NONE', ( #15769 ), #8719, .F. ) ;
#2585=VERTEX_POINT ( 'NONE', #6563 ) ;
#2588=LINE ( 'NONE', #11370, #27832 ) ;
#2597=VECTOR ( 'NONE', #8108, 1000.000000000000000 ) ;
#2600=ORIENTED_EDGE ( 'NONE', *, *, #12084, .T. ) ;
#2601=LINE ( 'NONE', #9651, #18752 ) ;
#2602=ADVANCED_FACE ( 'NONE', ( #11748 ), #18342, .F. ) ;
#2604=LINE ( 'NONE', #15847, #15708 ) ;
#2606=EDGE_LOOP ( 'NONE', ( #8460, #6398, #1942, #7606 ) ) ;
#2607=CARTESIAN_POINT ( 'NONE',  ( 158.0000000000016769, 45.95662448201407102, 45.00000000000000000 ) ) ;
#2609=CARTESIAN_POINT ( 'NONE',  ( 158.0000000000005969, 150.7794997898028271, 45.00000000000000000 ) ) ;
#2610=EDGE_LOOP ( 'NONE', ( #18879, #22337, #17926, #19287 ) ) ;
#2613=CARTESIAN_POINT ( 'NONE',  ( 157.9999999999997158, 256.6181251126050711, -45.00000000000000000 ) ) ;
#2616=ORIENTED_EDGE ( 'NONE', *, *, #4768, .F. ) ;
#2618=VECTOR ( 'NONE', #17782, 1000.000000000000227 ) ;
#2619=DIRECTION ( 'NONE',  ( -0.000000000000000000, -0.000000000000000000, -1.000000000000000000 ) ) ;
#2622=EDGE_LOOP ( 'NONE', ( #6693, #15964, #9841, #25577 ) ) ;
#2624=ADVANCED_FACE ( 'NONE', ( #5396 ), #9441, .F. ) ;
#2629=LINE ( 'NONE', #18579, #19751 ) ;
#2631=AXIS2_PLACEMENT_3D ( 'NONE', #16120, #11677, #24731 ) ;
#2633=LINE ( 'NONE', #27057, #8637 ) ;
#2636=CARTESIAN_POINT ( 'NONE',  ( 158.0000000000013074, 83.06687458711267880, -45.00000000000000000 ) ) ;
#2637=DIRECTION ( 'NONE',  ( -0.000000000000000000, 0.000000000000000000, -1.000000000000000000 ) ) ;
#2638=CARTESIAN_POINT ( 'NONE',  ( 157.9999999999996589, 271.6653751576470768, 45.00000000000000000 ) ) ;
#2643=EDGE_CURVE ( 'NONE', #14501, #16770, #18055, .T. ) ;
#2644=DIRECTION ( 'NONE',  ( -0.8916010070293783896, 0.4528218681382319422, 0.000000000000000000 ) ) ;
#2645=FACE_OUTER_BOUND ( 'NONE', #28388, .T. ) ;
#2647=VERTEX_POINT ( 'NONE', #13904 ) ;
#2648=CARTESIAN_POINT ( 'NONE',  ( 157.9999999999998010, 234.0472500450420341, 45.00000000000000000 ) ) ;
#2650=ORIENTED_EDGE ( 'NONE', *, *, #12288, .T. ) ;
#2653=DIRECTION ( 'NONE',  ( 0.8916010070293584056, 0.4528218681382713551, 0.000000000000000000 ) ) ;
#2655=EDGE_CURVE ( 'NONE', #23386, #26778, #26812, .T. ) ;
#2658=ORIENTED_EDGE ( 'NONE', *, *, #3507, .F. ) ;
#2659=VECTOR ( 'NONE', #22110, 1000.000000000000000 ) ;
#2668=DIRECTION ( 'NONE',  ( 0.4528218681377111920, 0.8916010070296429557, -0.000000000000000000 ) ) ;
#2678=EDGE_CURVE ( 'NONE', #26178, #16274, #14311, .T. ) ;
#2683=DIRECTION ( 'NONE',  ( 0.8916010070297244461, 0.4528218681375507093, 0.000000000000000000 ) ) ;
#2685=DIRECTION ( 'NONE',  ( 0.4528218681376112720, -0.8916010070296936929, 0.000000000000000000 ) ) ;
#2689=ORIENTED_EDGE ( 'NONE', *, *, #2015, .F. ) ;
#2690=EDGE_CURVE ( 'NONE', #8556, #9050, #1228, .T. ) ;
#2692=ORIENTED_EDGE ( 'NONE', *, *, #7895, .F. ) ;
#2694=ORIENTED_EDGE ( 'NONE', *, *, #22102, .F. ) ;
#2696=CARTESIAN_POINT ( 'NONE',  ( 158.0000000000016485, 50.46449948952111697, 45.00000000000000000 ) ) ;
#2698=VECTOR ( 'NONE', #25850, 1000.000000000000000 ) ;
#2702=CARTESIAN_POINT ( 'NONE',  ( 157.9999999999998863, 218.4921249924925348, -45.00000000000000000 ) ) ;
#2705=DIRECTION ( 'NONE',  ( 0.8916010070295817824, -0.4528218681378317623, 0.000000000000000000 ) ) ;
#2709=DIRECTION ( 'NONE',  ( 0.8916010070294598799, -0.4528218681380714594, 0.000000000000000000 ) ) ;
#2719=ORIENTED_EDGE ( 'NONE', *, *, #19437, .F. ) ;
#2722=LINE ( 'NONE', #15961, #25807 ) ;
#2723=VERTEX_POINT ( 'NONE', #3233 ) ;
#2726=VERTEX_POINT ( 'NONE', #12019 ) ;
#2727=LINE ( 'NONE', #24857, #11603 ) ;
#2729=ORIENTED_EDGE ( 'NONE', *, *, #25118, .T. ) ;
#2731=DIRECTION ( 'NONE',  ( 0.4528218681381114274, 0.8916010070294396739, -0.000000000000000000 ) ) ;
#2733=VECTOR ( 'NONE', #15131, 1000.000000000000000 ) ;
#2738=VECTOR ( 'NONE', #20211, 1000.000000000000000 ) ;
#2742=ORIENTED_EDGE ( 'NONE', *, *, #20084, .T. ) ;
#2743=CARTESIAN_POINT ( 'NONE',  ( 157.4999999999998579, 173.6043123611196961, 45.00000000000000000 ) ) ;
#2744=CARTESIAN_POINT ( 'NONE',  ( 157.4999999999998579, 186.1436873986549188, -45.00000000000000000 ) ) ;
#2747=ORIENTED_EDGE ( 'NONE', *, *, #18498, .F. ) ;
#2749=VECTOR ( 'NONE', #22212, 1000.000000000000000 ) ;
#2752=CARTESIAN_POINT ( 'NONE',  ( 157.9999999999996589, 276.1732501651540588, 45.00000000000000000 ) ) ;
#2754=EDGE_LOOP ( 'NONE', ( #2125, #21029, #23401, #26672 ) ) ;
#2755=AXIS2_PLACEMENT_3D ( 'NONE', #10625, #15513, #6729 ) ;
#2756=CARTESIAN_POINT ( 'NONE',  ( 158.0000000000011084, 100.6219996396619791, -45.00000000000000000 ) ) ;
#2759=EDGE_CURVE ( 'NONE', #21594, #12113, #12588, .T. ) ;
#2760=ORIENTED_EDGE ( 'NONE', *, *, #14624, .F. ) ;
#2763=EDGE_CURVE ( 'NONE', #9667, #19459, #5816, .T. ) ;
#2764=CARTESIAN_POINT ( 'NONE',  ( 157.9999999999998010, 238.5551250525490161, 45.00000000000000000 ) ) ;
#2765=EDGE_CURVE ( 'NONE', #16796, #20071, #12306, .T. ) ;
#2766=EDGE_LOOP ( 'NONE', ( #16076, #1248, #23199, #17925 ) ) ;
#2767=CARTESIAN_POINT ( 'NONE',  ( 158.0000000000006253, 146.2716247822957598, -45.00000000000000000 ) ) ;
#2768=VERTEX_POINT ( 'NONE', #12726 ) ;
#2769=DIRECTION ( 'NONE',  ( -0.000000000000000000, -0.000000000000000000, -1.000000000000000000 ) ) ;
#2775=DIRECTION ( 'NONE',  ( -0.8916010070296940260, -0.4528218681376106058, 0.000000000000000000 ) ) ;
#2776=VECTOR ( 'NONE', #15227, 1000.000000000000000 ) ;
#2781=DIRECTION ( 'NONE',  ( 0.4528218681375306698, -0.8916010070297345491, 0.000000000000000000 ) ) ;
#2786=CARTESIAN_POINT ( 'NONE',  ( 157.9999999999997726, 246.0787500750700474, 45.00000000000000000 ) ) ;
#2789=ORIENTED_EDGE ( 'NONE', *, *, #758, .F. ) ;
#2794=EDGE_CURVE ( 'NONE', #16382, #12868, #16604, .T. ) ;
#2795=VECTOR ( 'NONE', #23029, 1000.000000000000000 ) ;
#2797=ORIENTED_EDGE ( 'NONE', *, *, #24019, .F. ) ;
#2799=VERTEX_POINT ( 'NONE', #19169 ) ;
#2806=ORIENTED_EDGE ( 'NONE', *, *, #28361, .T. ) ;
#2809=DIRECTION ( 'NONE',  ( 0.4528218681376712240, -0.8916010070296632728, 0.000000000000000000 ) ) ;
#2810=CARTESIAN_POINT ( 'NONE',  ( 157.4999999999998579, 141.0019372635281627, 45.00000000000000000 ) ) ;
#2811=CARTESIAN_POINT ( 'NONE',  ( 187.4999999999996305, 40.68693696324645970, 45.00000000000000000 ) ) ;
#2816=CARTESIAN_POINT ( 'NONE',  ( 158.0000000000017053, 45.44874947450702507, 45.00000000000000000 ) ) ;
#2820=FACE_OUTER_BOUND ( 'NONE', #14547, .T. ) ;
#2836=AXIS2_PLACEMENT_3D ( 'NONE', #4769, #6783, #21876 ) ;
#2840=LINE ( 'NONE', #20225, #20756 ) ;
#2856=EDGE_CURVE ( 'NONE', #16854, #11176, #25917, .T. ) ;
#2859=DIRECTION ( 'NONE',  ( -0.000000000000000000, -0.000000000000000000, -1.000000000000000000 ) ) ;
#2861=CARTESIAN_POINT ( 'NONE',  ( 157.4999999999998295, 218.7460624962465090, 45.00000000000000000 ) ) ;
#2869=ORIENTED_EDGE ( 'NONE', *, *, #26398, .T. ) ;
#2871=CARTESIAN_POINT ( 'NONE',  ( 157.9999999999996874, 264.1417501351260171, 45.00000000000000000 ) ) ;
#2877=DIRECTION ( 'NONE',  ( 0.8916010070293584056, -0.4528218681382712996, 0.000000000000000000 ) ) ;
#2880=VECTOR ( 'NONE', #26856, 1000.000000000000114 ) ;
#2881=CARTESIAN_POINT ( 'NONE',  ( 157.4999999999998579, 88.33656210588026170, 45.00000000000000000 ) ) ;
#2882=ORIENTED_EDGE ( 'NONE', *, *, #28094, .F. ) ;
#2883=LINE ( 'NONE', #26579, #15567 ) ;
#2888=DIRECTION ( 'NONE',  ( 0.4528218681369517995, -0.8916010070300285362, 0.000000000000000000 ) ) ;
#2892=DIRECTION ( 'NONE',  ( -0.8916010070295820045, -0.4528218681378310406, 0.000000000000000000 ) ) ;
#2894=PLANE ( 'NONE',  #6162 ) ;
#2896=ADVANCED_FACE ( 'NONE', ( #15306 ), #350, .F. ) ;
#2914=PLANE ( 'NONE',  #24752 ) ;
#2920=CARTESIAN_POINT ( 'NONE',  ( 157.4999999999998010, 238.8090625563025071, -45.00000000000000000 ) ) ;
#2926=ORIENTED_EDGE ( 'NONE', *, *, #20422, .F. ) ;
#2928=EDGE_CURVE ( 'NONE', #26764, #20915, #60, .T. ) ;
#2931=LINE ( 'NONE', #25742, #1566 ) ;
#2933=LINE ( 'NONE', #11854, #21069 ) ;
#2942=ORIENTED_EDGE ( 'NONE', *, *, #14191, .T. ) ;
#2949=CARTESIAN_POINT ( 'NONE',  ( 157.9999999999998295, 228.5236250225210313, 45.00000000000000000 ) ) ;
#2950=VERTEX_POINT ( 'NONE', #8548 ) ;
#2953=DIRECTION ( 'NONE',  ( 0.8916010070298968637, 0.4528218681372110366, 0.000000000000000000 ) ) ;
#2955=DIRECTION ( 'NONE',  ( 0.8916010070297643031, -0.4528218681374719945, 0.000000000000000000 ) ) ;
#2957=LINE ( 'NONE', #20486, #13333 ) ;
#2958=CARTESIAN_POINT ( 'NONE',  ( 158.0000000000006537, 143.2558747672816821, 45.00000000000000000 ) ) ;
#2959=DIRECTION ( 'NONE',  ( -0.000000000000000000, -0.000000000000000000, -1.000000000000000000 ) ) ;
#2961=LINE ( 'NONE', #3094, #258 ) ;
#2964=DIRECTION ( 'NONE',  ( 1.000000000000000000, -0.000000000000000000, -0.000000000000000000 ) ) ;
#2965=VERTEX_POINT ( 'NONE', #13013 ) ;
#2966=ADVANCED_FACE ( 'NONE', ( #4494 ), #22036, .F. ) ;
#2969=CARTESIAN_POINT ( 'NONE',  ( 157.4999999999998579, 48.21056198576756202, -45.00000000000000000 ) ) ;
#2970=DIRECTION ( 'NONE',  ( -0.000000000000000000, -0.000000000000000000, -1.000000000000000000 ) ) ;
#2971=ORIENTED_EDGE ( 'NONE', *, *, #602, .F. ) ;
#2974=CARTESIAN_POINT ( 'NONE',  ( 157.4999999999998579, 161.0649373235845019, 45.00000000000000000 ) ) ;
#2975=VECTOR ( 'NONE', #26273, 1000.000000000000000 ) ;
#2978=ORIENTED_EDGE ( 'NONE', *, *, #3119, .F. ) ;
#2985=EDGE_CURVE ( 'NONE', #26387, #28088, #26470, .T. ) ;
#2993=DIRECTION ( 'NONE',  ( 1.000000000000000000, 0.000000000000000000, -0.000000000000000000 ) ) ;
#2994=CARTESIAN_POINT ( 'NONE',  ( 157.4999999999998579, 186.1436873986549188, 45.00000000000000000 ) ) ;
#2995=CARTESIAN_POINT ( 'NONE',  ( 157.9999999999997726, 246.0787500750700474, -45.00000000000000000 ) ) ;
#3002=ORIENTED_EDGE ( 'NONE', *, *, #21641, .F. ) ;
#3003=ORIENTED_EDGE ( 'NONE', *, *, #16317, .T. ) ;
#3006=ORIENTED_EDGE ( 'NONE', *, *, #13984, .F. ) ;
#3007=EDGE_LOOP ( 'NONE', ( #25067, #14646, #11977, #22024 ) ) ;
#3008=CARTESIAN_POINT ( 'NONE',  ( 158.0000000000004547, 165.8267498348450886, 45.00000000000000000 ) ) ;
#3013=DIRECTION ( 'NONE',  ( 0.4528218681371123377, 0.8916010070299471568, -0.000000000000000000 ) ) ;
#3016=EDGE_CURVE ( 'NONE', #9494, #17780, #13574, .T. ) ;
#3021=EDGE_CURVE ( 'NONE', #21473, #465, #15162, .T. ) ;
#3025=LINE ( 'NONE', #11815, #5441 ) ;
#3028=FACE_OUTER_BOUND ( 'NONE', #17339, .T. ) ;
#3030=VECTOR ( 'NONE', #28227, 1000.000000000000000 ) ;
#3031=CARTESIAN_POINT ( 'NONE',  ( 157.9999999999998579, 223.5078750075070104, -45.00000000000000000 ) ) ;
#3041=VERTEX_POINT ( 'NONE', #10841 ) ;
#3049=EDGE_LOOP ( 'NONE', ( #7544, #24574, #24216, #1672 ) ) ;
#3051=CARTESIAN_POINT ( 'NONE',  ( 158.0000000000002842, 180.8739998798873501, 45.00000000000000000 ) ) ;
#3053=LINE ( 'NONE', #9103, #18156 ) ;
#3054=ADVANCED_FACE ( 'NONE', ( #5361 ), #16433, .F. ) ;
#3058=CARTESIAN_POINT ( 'NONE',  ( 157.4999999999997158, 258.8720626163585621, 45.00000000000000000 ) ) ;
#3061=DIRECTION ( 'NONE',  ( 0.4528218681383106015, -0.8916010070293384215, 0.000000000000000000 ) ) ;
#3062=LINE ( 'NONE', #25054, #4201 ) ;
#3064=EDGE_LOOP ( 'NONE', ( #24679, #9834, #9074, #1280 ) ) ;
#3066=ORIENTED_EDGE ( 'NONE', *, *, #8083, .T. ) ;
#3067=CARTESIAN_POINT ( 'NONE',  ( 158.0000000000007105, 136.2401247522676044, 45.00000000000000000 ) ) ;
#3072=EDGE_LOOP ( 'NONE', ( #18178, #16627, #23320, #26522 ) ) ;
#3079=LINE ( 'NONE', #16039, #11336 ) ;
#3081=VERTEX_POINT ( 'NONE', #9253 ) ;
#3083=ADVANCED_FACE ( 'NONE', ( #15877 ), #25050, .F. ) ;
#3084=DIRECTION ( 'NONE',  ( 0.4528218681375507093, -0.8916010070297244461, 0.000000000000000000 ) ) ;
#3085=EDGE_CURVE ( 'NONE', #24784, #22271, #7388, .T. ) ;
#3086=DIRECTION ( 'NONE',  ( -0.8916010070291696676, -0.4528218681386429467, 0.000000000000000000 ) ) ;
#3087=CARTESIAN_POINT ( 'NONE',  ( 157.9999999999998010, 234.0472500450420341, 45.00000000000000000 ) ) ;
#3094=CARTESIAN_POINT ( 'NONE',  ( 158.0000000000005400, 153.7952498048169048, 45.00000000000000000 ) ) ;
#3098=ORIENTED_EDGE ( 'NONE', *, *, #12175, .F. ) ;
#3099=CARTESIAN_POINT ( 'NONE',  ( 158.0000000000012221, 88.59049960963380954, 45.00000000000000000 ) ) ;
#3100=CARTESIAN_POINT ( 'NONE',  ( 158.0000000000015064, 61.00387452705632541, 45.00000000000000000 ) ) ;
#3102=ORIENTED_EDGE ( 'NONE', *, *, #25457, .T. ) ;
#3104=PLANE ( 'NONE',  #24460 ) ;
#3105=VERTEX_POINT ( 'NONE', #16015 ) ;
#3106=EDGE_CURVE ( 'NONE', #24374, #14709, #11566, .T. ) ;
#3107=CARTESIAN_POINT ( 'NONE',  ( 157.4999999999998579, 110.9074371734436255, 45.00000000000000000 ) ) ;
#3116=EDGE_CURVE ( 'NONE', #12076, #20506, #14007, .T. ) ;
#3119=EDGE_CURVE ( 'NONE', #26387, #27071, #27326, .T. ) ;
#3127=LINE ( 'NONE', #13942, #692 ) ;
#3134=CARTESIAN_POINT ( 'NONE',  ( 158.0000000000014779, 65.51174953456337846, 45.00000000000000000 ) ) ;
#3135=ORIENTED_EDGE ( 'NONE', *, *, #21874, .T. ) ;
#3136=ORIENTED_EDGE ( 'NONE', *, *, #25118, .F. ) ;
#3139=EDGE_LOOP ( 'NONE', ( #20259, #24153, #27974, #18916 ) ) ;
#3140=ORIENTED_EDGE ( 'NONE', *, *, #25473, .T. ) ;
#3141=EDGE_CURVE ( 'NONE', #25239, #18389, #20454, .T. ) ;
#3150=CARTESIAN_POINT ( 'NONE',  ( 157.4999999999998579, 113.4153121809506786, 45.00000000000000000 ) ) ;
#3153=CARTESIAN_POINT ( 'NONE',  ( 157.4999999999996589, 273.9193126614005678, 45.00000000000000000 ) ) ;
#3158=PLANE ( 'NONE',  #5725 ) ;
#3161=AXIS2_PLACEMENT_3D ( 'NONE', #6603, #4723, #24270 ) ;
#3162=DIRECTION ( 'NONE',  ( 0.4528218681383106015, -0.8916010070293384215, 0.000000000000000000 ) ) ;
#3167=LINE ( 'NONE', #9656, #23842 ) ;
#3174=EDGE_CURVE ( 'NONE', #5095, #17304, #27603, .T. ) ;
#3175=EDGE_CURVE ( 'NONE', #27514, #5337, #19000, .T. ) ;
#3178=DIRECTION ( 'NONE',  ( 0.000000000000000000, -1.000000000000000000, 0.000000000000000000 ) ) ;
#3180=VECTOR ( 'NONE', #10372, 1000.000000000000000 ) ;
#3181=ORIENTED_EDGE ( 'NONE', *, *, #8775, .T. ) ;
#3184=CARTESIAN_POINT ( 'NONE',  ( 158.0000000000007958, 130.7164997297464595, 45.00000000000000000 ) ) ;
#3186=ORIENTED_EDGE ( 'NONE', *, *, #27187, .T. ) ;
#3188=ORIENTED_EDGE ( 'NONE', *, *, #11568, .T. ) ;
#3194=LINE ( 'NONE', #7663, #13532 ) ;
#3195=LINE ( 'NONE', #27877, #14968 ) ;
#3196=DIRECTION ( 'NONE',  ( -0.000000000000000000, -0.000000000000000000, -1.000000000000000000 ) ) ;
#3197=DIRECTION ( 'NONE',  ( -0.000000000000000000, -0.000000000000000000, -1.000000000000000000 ) ) ;
#3198=CARTESIAN_POINT ( 'NONE',  ( 157.9999999999996589, 271.6653751576470768, 45.00000000000000000 ) ) ;
#3200=VECTOR ( 'NONE', #7699, 1000.000000000000000 ) ;
#3202=CARTESIAN_POINT ( 'NONE',  ( 157.9999999999997158, 261.6338751276190351, 45.00000000000000000 ) ) ;
#3203=FACE_OUTER_BOUND ( 'NONE', #3895, .T. ) ;
#3205=EDGE_CURVE ( 'NONE', #11076, #15637, #18257, .T. ) ;
#3206=LINE ( 'NONE', #25188, #27014 ) ;
#3207=VECTOR ( 'NONE', #22991, 1000.000000000000000 ) ;
#3208=ORIENTED_EDGE ( 'NONE', *, *, #15670, .F. ) ;
#3209=EDGE_CURVE ( 'NONE', #7922, #6186, #22844, .T. ) ;
#3214=CARTESIAN_POINT ( 'NONE',  ( 157.4999999999997726, 248.8405625863305204, 45.00000000000000000 ) ) ;
#3219=ORIENTED_EDGE ( 'NONE', *, *, #9095, .F. ) ;
#3221=DIRECTION ( 'NONE',  ( 0.8916010070295511403, -0.4528218681378915478, 0.000000000000000000 ) ) ;
#3223=VECTOR ( 'NONE', #11605, 1000.000000000000000 ) ;
#3227=VECTOR ( 'NONE', #9449, 1000.000000000000000 ) ;
#3231=DIRECTION ( 'NONE',  ( 0.4528218681386429467, -0.8916010070291696676, 0.000000000000000000 ) ) ;
#3232=LINE ( 'NONE', #11747, #9676 ) ;
#3233=CARTESIAN_POINT ( 'NONE',  ( 157.9999999999996305, 286.7126252026890256, 45.00000000000000000 ) ) ;
#3234=LINE ( 'NONE', #12020, #3321 ) ;
#3235=DIRECTION ( 'NONE',  ( -0.8916010070293584056, -0.4528218681382712996, 0.000000000000000000 ) ) ;
#3237=CARTESIAN_POINT ( 'NONE',  ( 157.4999999999996589, 278.9350626764145318, 45.00000000000000000 ) ) ;
#3244=LINE ( 'NONE', #11619, #15224 ) ;
#3246=ADVANCED_FACE ( 'NONE', ( #5597 ), #27148, .F. ) ;
#3247=ADVANCED_FACE ( 'NONE', ( #5176 ), #22568, .F. ) ;
#3250=FACE_OUTER_BOUND ( 'NONE', #15423, .T. ) ;
#3251=EDGE_CURVE ( 'NONE', #14501, #26726, #3290, .T. ) ;
#3255=ORIENTED_EDGE ( 'NONE', *, *, #6714, .F. ) ;
#3257=DIRECTION ( 'NONE',  ( -0.8916010070296632728, 0.4528218681376712240, 0.000000000000000000 ) ) ;
#3258=DIRECTION ( 'NONE',  ( 0.4528218681382713551, 0.8916010070293584056, -0.000000000000000000 ) ) ;
#3259=AXIS2_PLACEMENT_3D ( 'NONE', #14736, #14885, #19318 ) ;
#3263=LINE ( 'NONE', #9888, #1546 ) ;
#3265=DIRECTION ( 'NONE',  ( 0.8916010070297446521, 0.4528218681375106858, 0.000000000000000000 ) ) ;
#3266=CARTESIAN_POINT ( 'NONE',  ( 158.0000000000000284, 203.9527499549551806, -45.00000000000000000 ) ) ;
#3269=CARTESIAN_POINT ( 'NONE',  ( 157.4999999999998579, 186.1436873986549188, 45.00000000000000000 ) ) ;
#3276=ORIENTED_EDGE ( 'NONE', *, *, #4426, .F. ) ;
#3280=DIRECTION ( 'NONE',  ( 0.000000000000000000, -1.000000000000000000, 0.000000000000000000 ) ) ;
#3282=VERTEX_POINT ( 'NONE', #16111 ) ;
#3283=ORIENTED_EDGE ( 'NONE', *, *, #1605, .T. ) ;
#3286=ORIENTED_EDGE ( 'NONE', *, *, #11806, .T. ) ;
#3288=EDGE_LOOP ( 'NONE', ( #12041, #27248, #2971, #24568 ) ) ;
#3290=LINE ( 'NONE', #9357, #13528 ) ;
#3292=DIRECTION ( 'NONE',  ( -0.000000000000000000, -0.000000000000000000, -1.000000000000000000 ) ) ;
#3298=PLANE ( 'NONE',  #10930 ) ;
#3302=ADVANCED_FACE ( 'NONE', ( #27283 ), #20403, .F. ) ;
#3305=LINE ( 'NONE', #12099, #4692 ) ;
#3310=EDGE_CURVE ( 'NONE', #2723, #28076, #12080, .T. ) ;
#3312=ORIENTED_EDGE ( 'NONE', *, *, #18313, .F. ) ;
#3315=EDGE_LOOP ( 'NONE', ( #298, #4278, #7540, #20495 ) ) ;
#3317=VECTOR ( 'NONE', #19745, 1000.000000000000000 ) ;
#3319=CARTESIAN_POINT ( 'NONE',  ( 157.9999999999998579, 221.0000000000000284, 45.00000000000000000 ) ) ;
#3320=ORIENTED_EDGE ( 'NONE', *, *, #11587, .T. ) ;
#3321=VECTOR ( 'NONE', #1088, 1000.000000000000000 ) ;
#3322=ORIENTED_EDGE ( 'NONE', *, *, #10106, .F. ) ;
#3323=FACE_OUTER_BOUND ( 'NONE', #6619, .T. ) ;
#3324=VECTOR ( 'NONE', #12427, 1000.000000000000000 ) ;
#3327=VERTEX_POINT ( 'NONE', #22393 ) ;
#3331=DIRECTION ( 'NONE',  ( 0.000000000000000000, -1.000000000000000000, 0.000000000000000000 ) ) ;
#3332=LINE ( 'NONE', #9678, #8007 ) ;
#3333=EDGE_CURVE ( 'NONE', #17412, #14898, #11491, .T. ) ;
#3335=FACE_OUTER_BOUND ( 'NONE', #6771, .T. ) ;
#3336=VECTOR ( 'NONE', #18884, 1000.000000000000000 ) ;
#3337=CARTESIAN_POINT ( 'NONE',  ( 157.9999999999999147, 215.9842499849850697, -45.00000000000000000 ) ) ;
#3340=VERTEX_POINT ( 'NONE', #563 ) ;
#3344=CARTESIAN_POINT ( 'NONE',  ( 157.4999999999996589, 276.4271876689075498, -45.00000000000000000 ) ) ;
#3346=LINE ( 'NONE', #20460, #13963 ) ;
#3347=ORIENTED_EDGE ( 'NONE', *, *, #12084, .F. ) ;
#3351=EDGE_CURVE ( 'NONE', #12823, #2799, #13356, .T. ) ;
#3354=CARTESIAN_POINT ( 'NONE',  ( 158.0000000000008811, 123.1928747072253572, 45.00000000000000000 ) ) ;
#3355=ORIENTED_EDGE ( 'NONE', *, *, #3106, .T. ) ;
#3356=DIRECTION ( 'NONE',  ( 0.000000000000000000, -1.000000000000000000, 0.000000000000000000 ) ) ;
#3358=EDGE_CURVE ( 'NONE', #19001, #4212, #11344, .T. ) ;
#3360=DIRECTION ( 'NONE',  ( 0.4528218681379916899, 0.8916010070295005141, -0.000000000000000000 ) ) ;
#3367=VERTEX_POINT ( 'NONE', #13645 ) ;
#3371=DIRECTION ( 'NONE',  ( -0.000000000000000000, 0.000000000000000000, -1.000000000000000000 ) ) ;
#3381=CARTESIAN_POINT ( 'NONE',  ( 158.0000000000005969, 148.7794997898028271, -45.00000000000000000 ) ) ;
#3383=VECTOR ( 'NONE', #15301, 1000.000000000000000 ) ;
#3386=LINE ( 'NONE', #3668, #10307 ) ;
#3388=AXIS2_PLACEMENT_3D ( 'NONE', #9930, #8873, #4275 ) ;
#3389=ORIENTED_EDGE ( 'NONE', *, *, #3390, .T. ) ;
#3390=EDGE_CURVE ( 'NONE', #8705, #25194, #26980, .T. ) ;
#3391=EDGE_CURVE ( 'NONE', #24175, #3560, #15656, .T. ) ;
#3392=CARTESIAN_POINT ( 'NONE',  ( 157.4999999999998579, 75.79718706834503905, 45.00000000000000000 ) ) ;
#3397=EDGE_LOOP ( 'NONE', ( #27837, #13204, #25032, #12686 ) ) ;
#3398=VERTEX_POINT ( 'NONE', #27124 ) ;
#3399=CARTESIAN_POINT ( 'NONE',  ( 157.4999999999998295, 231.2854375337815327, 45.00000000000000000 ) ) ;
#3409=DIRECTION ( 'NONE',  ( -0.000000000000000000, -0.000000000000000000, -1.000000000000000000 ) ) ;
#3411=DIRECTION ( 'NONE',  ( -0.000000000000000000, -0.000000000000000000, -1.000000000000000000 ) ) ;
#3413=EDGE_CURVE ( 'NONE', #9316, #9313, #24547, .T. ) ;
#3417=ORIENTED_EDGE ( 'NONE', *, *, #3562, .T. ) ;
#3420=CARTESIAN_POINT ( 'NONE',  ( 158.0000000000006821, 138.7479997597746433, -45.00000000000000000 ) ) ;
#3422=EDGE_LOOP ( 'NONE', ( #8605, #10326, #19321, #18529 ) ) ;
#3424=CARTESIAN_POINT ( 'NONE',  ( 157.9999999999996305, 283.6968751876750616, 45.00000000000000000 ) ) ;
#3425=ORIENTED_EDGE ( 'NONE', *, *, #8352, .F. ) ;
#3434=CARTESIAN_POINT ( 'NONE',  ( 157.4999999999997158, 263.8878126313725829, 45.00000000000000000 ) ) ;
#3435=VECTOR ( 'NONE', #23064, 1000.000000000000000 ) ;
#3438=EDGE_CURVE ( 'NONE', #1247, #28076, #26690, .T. ) ;
#3441=CARTESIAN_POINT ( 'NONE',  ( 158.0000000000009948, 110.6534996696901345, -45.00000000000000000 ) ) ;
#3446=CARTESIAN_POINT ( 'NONE',  ( 157.4999999999998579, 201.1909374436971802, 45.00000000000000000 ) ) ;
#3450=CARTESIAN_POINT ( 'NONE',  ( 157.9999999999997726, 241.5708750675630370, 45.00000000000000000 ) ) ;
#3458=ORIENTED_EDGE ( 'NONE', *, *, #20779, .F. ) ;
#3459=CARTESIAN_POINT ( 'NONE',  ( 158.0000000000005400, 153.7952498048169048, -45.00000000000000000 ) ) ;
#3462=ORIENTED_EDGE ( 'NONE', *, *, #12175, .T. ) ;
#3465=ORIENTED_EDGE ( 'NONE', *, *, #2047, .T. ) ;
#3469=ORIENTED_EDGE ( 'NONE', *, *, #18144, .F. ) ;
#3471=CARTESIAN_POINT ( 'NONE',  ( 158.0000000000006537, 145.7637497747887210, -45.00000000000000000 ) ) ;
#3477=AXIS2_PLACEMENT_3D ( 'NONE', #16366, #27392, #3265 ) ;
#3478=DIRECTION ( 'NONE',  ( -0.000000000000000000, -0.000000000000000000, -1.000000000000000000 ) ) ;
#3479=CARTESIAN_POINT ( 'NONE',  ( 158.0000000000000000, 206.4606249624626457, 45.00000000000000000 ) ) ;
#3481=VECTOR ( 'NONE', #17462, 1000.000000000000000 ) ;
#3487=DIRECTION ( 'NONE',  ( -0.000000000000000000, -0.000000000000000000, -1.000000000000000000 ) ) ;
#3489=CARTESIAN_POINT ( 'NONE',  ( 158.0000000000015348, 60.49599951954928656, -45.00000000000000000 ) ) ;
#3490=VERTEX_POINT ( 'NONE', #20802 ) ;
#3492=ORIENTED_EDGE ( 'NONE', *, *, #24622, .F. ) ;
#3497=DIRECTION ( 'NONE',  ( 0.8916010070294503320, 0.4528218681380901667, 0.000000000000000000 ) ) ;
#3498=DIRECTION ( 'NONE',  ( 1.000000000000000000, 0.000000000000000000, -0.000000000000000000 ) ) ;
#3501=LINE ( 'NONE', #7822, #15418 ) ;
#3506=ORIENTED_EDGE ( 'NONE', *, *, #16241, .F. ) ;
#3507=EDGE_CURVE ( 'NONE', #24186, #13425, #22959, .T. ) ;
#3510=ORIENTED_EDGE ( 'NONE', *, *, #25914, .F. ) ;
#3511=FACE_OUTER_BOUND ( 'NONE', #22148, .T. ) ;
#3517=EDGE_CURVE ( 'NONE', #3705, #4742, #23103, .T. ) ;
#3518=CARTESIAN_POINT ( 'NONE',  ( 158.0000000000009948, 110.6534996696901345, 45.00000000000000000 ) ) ;
#3519=CARTESIAN_POINT ( 'NONE',  ( 157.9999999999998010, 233.5393750375350237, -45.00000000000000000 ) ) ;
#3528=ORIENTED_EDGE ( 'NONE', *, *, #22375, .F. ) ;
#3537=EDGE_LOOP ( 'NONE', ( #24567, #26756, #26146, #13562 ) ) ;
#3538=ORIENTED_EDGE ( 'NONE', *, *, #23405, .T. ) ;
#3541=CARTESIAN_POINT ( 'NONE',  ( 158.0000000000001705, 190.9054999099155054, -45.00000000000000000 ) ) ;
#3543=VECTOR ( 'NONE', #20510, 1000.000000000000227 ) ;
#3544=PLANE ( 'NONE',  #19254 ) ;
#3551=CARTESIAN_POINT ( 'NONE',  ( 158.0000000000007674, 133.2243747372535267, 45.00000000000000000 ) ) ;
#3555=ORIENTED_EDGE ( 'NONE', *, *, #12480, .T. ) ;
#3556=VECTOR ( 'NONE', #12408, 1000.000000000000000 ) ;
#3559=ORIENTED_EDGE ( 'NONE', *, *, #15075, .F. ) ;
#3560=VERTEX_POINT ( 'NONE', #10030 ) ;
#3562=EDGE_CURVE ( 'NONE', #8486, #12219, #18648, .T. ) ;
#3564=CARTESIAN_POINT ( 'NONE',  ( 157.4999999999998579, 100.8759371434154701, -45.00000000000000000 ) ) ;
#3565=EDGE_LOOP ( 'NONE', ( #7999, #9561, #19090, #1648 ) ) ;
#3566=ORIENTED_EDGE ( 'NONE', *, *, #6435, .F. ) ;
#3569=EDGE_CURVE ( 'NONE', #17818, #10126, #14487, .T. ) ;
#3570=ORIENTED_EDGE ( 'NONE', *, *, #1441, .T. ) ;
#3573=AXIS2_PLACEMENT_3D ( 'NONE', #1406, #16784, #25676 ) ;
#3574=AXIS2_PLACEMENT_3D ( 'NONE', #29, #26440, #11238 ) ;
#3575=DIRECTION ( 'NONE',  ( -0.8916010070297643031, 0.4528218681374719390, 0.000000000000000000 ) ) ;
#3576=CARTESIAN_POINT ( 'NONE',  ( 158.0000000000014495, 68.01962454207041731, 45.00000000000000000 ) ) ;
#3580=CARTESIAN_POINT ( 'NONE',  ( 157.4999999999996305, 288.9665627064425735, -45.00000000000000000 ) ) ;
#3581=CARTESIAN_POINT ( 'NONE',  ( 158.0000000000013074, 81.06687458711267880, 45.00000000000000000 ) ) ;
#3587=ORIENTED_EDGE ( 'NONE', *, *, #2690, .F. ) ;
#3594=ORIENTED_EDGE ( 'NONE', *, *, #2546, .F. ) ;
#3599=ORIENTED_EDGE ( 'NONE', *, *, #7895, .T. ) ;
#3603=LINE ( 'NONE', #12539, #6998 ) ;
#3604=AXIS2_PLACEMENT_3D ( 'NONE', #4755, #7064, #13687 ) ;
#3608=ORIENTED_EDGE ( 'NONE', *, *, #11326, .F. ) ;
#3609=CARTESIAN_POINT ( 'NONE',  ( 157.9999999999999432, 213.4763749774776045, 45.00000000000000000 ) ) ;
#3610=AXIS2_PLACEMENT_3D ( 'NONE', #3237, #12026, #4230 ) ;
#3612=LINE ( 'NONE', #1741, #5255 ) ;
#3615=VECTOR ( 'NONE', #23912, 1000.000000000000000 ) ;
#3616=VECTOR ( 'NONE', #13110, 1000.000000000000114 ) ;
#3617=CARTESIAN_POINT ( 'NONE',  ( 158.0000000000012506, 88.08262460212675649, 45.00000000000000000 ) ) ;
#3619=ORIENTED_EDGE ( 'NONE', *, *, #8053, .F. ) ;
#3620=EDGE_CURVE ( 'NONE', #27544, #17314, #12339, .T. ) ;
#3623=FACE_OUTER_BOUND ( 'NONE', #22567, .T. ) ;
#3624=LINE ( 'NONE', #10250, #23125 ) ;
#3625=VERTEX_POINT ( 'NONE', #25109 ) ;
#3628=VECTOR ( 'NONE', #785, 1000.000000000000000 ) ;
#3631=DIRECTION ( 'NONE',  ( 0.000000000000000000, -1.000000000000000000, 0.000000000000000000 ) ) ;
#3632=VERTEX_POINT ( 'NONE', #5426 ) ;
#3638=EDGE_CURVE ( 'NONE', #13707, #2371, #24057, .T. ) ;
#3642=EDGE_CURVE ( 'NONE', #9971, #7332, #4637, .T. ) ;
#3644=VERTEX_POINT ( 'NONE', #8816 ) ;
#3646=AXIS2_PLACEMENT_3D ( 'NONE', #18958, #19524, #3575 ) ;
#3648=ORIENTED_EDGE ( 'NONE', *, *, #21408, .F. ) ;
#3650=ORIENTED_EDGE ( 'NONE', *, *, #19190, .T. ) ;
#3656=AXIS2_PLACEMENT_3D ( 'NONE', #24205, #4373, #23925 ) ;
#3660=LINE ( 'NONE', #1925, #5134 ) ;
#3661=DIRECTION ( 'NONE',  ( -0.000000000000000000, -0.000000000000000000, -1.000000000000000000 ) ) ;
#3662=FACE_OUTER_BOUND ( 'NONE', #207, .T. ) ;
#3665=ADVANCED_FACE ( 'NONE', ( #24477 ), #26336, .F. ) ;
#3667=CARTESIAN_POINT ( 'NONE',  ( 157.4999999999998579, 108.3995621659365867, -45.00000000000000000 ) ) ;
#3668=CARTESIAN_POINT ( 'NONE',  ( 157.4999999999998579, 135.9861872485140850, -45.00000000000000000 ) ) ;
#3675=CARTESIAN_POINT ( 'NONE',  ( 157.4999999999998579, 68.27356204582390831, 45.00000000000000000 ) ) ;
#3684=LINE ( 'NONE', #21074, #13291 ) ;
#3690=VECTOR ( 'NONE', #27640, 999.9999999999998863 ) ;
#3691=CARTESIAN_POINT ( 'NONE',  ( 158.0000000000005400, 156.3031248123239436, -45.00000000000000000 ) ) ;
#3695=CARTESIAN_POINT ( 'NONE',  ( 157.4999999999998579, 193.6673124211760353, 45.00000000000000000 ) ) ;
#3696=ORIENTED_EDGE ( 'NONE', *, *, #20832, .F. ) ;
#3697=VECTOR ( 'NONE', #8789, 1000.000000000000114 ) ;
#3698=EDGE_CURVE ( 'NONE', #9601, #543, #22033, .T. ) ;
#3701=VERTEX_POINT ( 'NONE', #10982 ) ;
#3704=ORIENTED_EDGE ( 'NONE', *, *, #21821, .T. ) ;
#3705=VERTEX_POINT ( 'NONE', #6664 ) ;
#3707=ADVANCED_FACE ( 'NONE', ( #4784 ), #23520, .F. ) ;
#3711=VERTEX_POINT ( 'NONE', #19876 ) ;
#3712=ORIENTED_EDGE ( 'NONE', *, *, #7995, .T. ) ;
#3716=DIRECTION ( 'NONE',  ( -0.000000000000000000, -0.000000000000000000, -1.000000000000000000 ) ) ;
#3719=EDGE_CURVE ( 'NONE', #3632, #18947, #24326, .T. ) ;
#3721=DIRECTION ( 'NONE',  ( 1.000000000000000000, 0.000000000000000000, -0.000000000000000000 ) ) ;
#3725=DIRECTION ( 'NONE',  ( 0.4528218681381114274, 0.8916010070294396739, -0.000000000000000000 ) ) ;
#3727=LINE ( 'NONE', #27430, #23966 ) ;
#3729=VECTOR ( 'NONE', #22338, 1000.000000000000000 ) ;
#3735=ORIENTED_EDGE ( 'NONE', *, *, #12256, .F. ) ;
#3736=ORIENTED_EDGE ( 'NONE', *, *, #26187, .F. ) ;
#3738=EDGE_CURVE ( 'NONE', #18572, #23905, #9106, .T. ) ;
#3740=LINE ( 'NONE', #12111, #20474 ) ;
#3741=ORIENTED_EDGE ( 'NONE', *, *, #1380, .F. ) ;
#3742=ORIENTED_EDGE ( 'NONE', *, *, #34, .T. ) ;
#3743=CARTESIAN_POINT ( 'NONE',  ( 158.0000000000013074, 81.06687458711267880, -45.00000000000000000 ) ) ;
#3745=DIRECTION ( 'NONE',  ( 0.8916010070298664436, 0.4528218681372709331, 0.000000000000000000 ) ) ;
#3749=ORIENTED_EDGE ( 'NONE', *, *, #15508, .F. ) ;
#3750=VECTOR ( 'NONE', #10399, 1000.000000000000000 ) ;
#3757=DIRECTION ( 'NONE',  ( -0.000000000000000000, 0.000000000000000000, -1.000000000000000000 ) ) ;
#3758=CARTESIAN_POINT ( 'NONE',  ( 187.4999999999996305, 288.9665627064425166, -45.00000000000000000 ) ) ;
#3761=LINE ( 'NONE', #9957, #17474 ) ;
#3766=DIRECTION ( 'NONE',  ( 0.000000000000000000, -1.000000000000000000, 0.000000000000000000 ) ) ;
#3767=DIRECTION ( 'NONE',  ( 1.000000000000000000, 0.000000000000000000, -0.000000000000000000 ) ) ;
#3771=CARTESIAN_POINT ( 'NONE',  ( 158.0000000000016200, 50.97237449702815582, 45.00000000000000000 ) ) ;
#3772=AXIS2_PLACEMENT_3D ( 'NONE', #26442, #11092, #6637 ) ;
#3784=ORIENTED_EDGE ( 'NONE', *, *, #386, .F. ) ;
#3785=EDGE_CURVE ( 'NONE', #26726, #689, #25048, .T. ) ;
#3788=ORIENTED_EDGE ( 'NONE', *, *, #6781, .T. ) ;
#3790=EDGE_LOOP ( 'NONE', ( #18605, #869, #6825, #26339 ) ) ;
#3792=LINE ( 'NONE', #25908, #18492 ) ;
#3795=DIRECTION ( 'NONE',  ( -1.000000000000000000, 0.000000000000000000, 0.000000000000000000 ) ) ;
#3798=ADVANCED_FACE ( 'NONE', ( #3335 ), #7240, .F. ) ;
#3804=ORIENTED_EDGE ( 'NONE', *, *, #22869, .F. ) ;
#3805=ADVANCED_FACE ( 'NONE', ( #11706 ), #20451, .F. ) ;
#3806=CARTESIAN_POINT ( 'NONE',  ( 158.0000000000007105, 138.2401247522676044, -45.00000000000000000 ) ) ;
#3809=CARTESIAN_POINT ( 'NONE',  ( 158.0000000000000568, 203.4448749474510407, 45.00000000000000000 ) ) ;
#3810=ORIENTED_EDGE ( 'NONE', *, *, #9140, .F. ) ;
#3814=CARTESIAN_POINT ( 'NONE',  ( 157.9999999999997442, 253.6023750975910502, 45.00000000000000000 ) ) ;
#3820=CARTESIAN_POINT ( 'NONE',  ( 157.4999999999996305, 286.4586876989355915, 45.00000000000000000 ) ) ;
#3823=ORIENTED_EDGE ( 'NONE', *, *, #5826, .F. ) ;
#3824=CARTESIAN_POINT ( 'NONE',  ( 157.9999999999997442, 249.0945000900840398, 45.00000000000000000 ) ) ;
#3826=ORIENTED_EDGE ( 'NONE', *, *, #14419, .F. ) ;
#3827=FACE_OUTER_BOUND ( 'NONE', #114, .T. ) ;
#3828=LINE ( 'NONE', #10445, #1349 ) ;
#3829=FACE_OUTER_BOUND ( 'NONE', #21521, .T. ) ;
#3834=DIRECTION ( 'NONE',  ( 0.8916010070296124246, -0.4528218681377710886, 0.000000000000000000 ) ) ;
#3838=EDGE_CURVE ( 'NONE', #23391, #14420, #11983, .T. ) ;
#3841=VECTOR ( 'NONE', #15312, 1000.000000000000114 ) ;
#3842=PLANE ( 'NONE',  #22092 ) ;
#3847=DIRECTION ( 'NONE',  ( 0.4528218681383106015, -0.8916010070293384215, 0.000000000000000000 ) ) ;
#3852=ORIENTED_EDGE ( 'NONE', *, *, #19794, .F. ) ;
#3854=AXIS2_PLACEMENT_3D ( 'NONE', #4782, #346, #15872 ) ;
#3860=FACE_OUTER_BOUND ( 'NONE', #6967, .T. ) ;
#3861=EDGE_CURVE ( 'NONE', #620, #4812, #5073, .T. ) ;
#3862=LINE ( 'NONE', #28128, #27047 ) ;
#3863=CARTESIAN_POINT ( 'NONE',  ( 158.0000000000008527, 123.7007497147323960, 45.00000000000000000 ) ) ;
#3867=CARTESIAN_POINT ( 'NONE',  ( 157.4999999999998579, 50.71843699327460797, 45.00000000000000000 ) ) ;
#3868=CARTESIAN_POINT ( 'NONE',  ( 157.4999999999998579, 93.35231212089433939, 45.00000000000000000 ) ) ;
#3870=VECTOR ( 'NONE', #7383, 1000.000000000000227 ) ;
#3871=ADVANCED_FACE ( 'NONE', ( #7093 ), #18440, .F. ) ;
#3877=ORIENTED_EDGE ( 'NONE', *, *, #27328, .T. ) ;
#3879=LINE ( 'NONE', #13095, #7611 ) ;
#3887=VERTEX_POINT ( 'NONE', #14138 ) ;
#3892=EDGE_CURVE ( 'NONE', #11526, #24469, #22887, .T. ) ;
#3895=EDGE_LOOP ( 'NONE', ( #27175, #6055, #359, #11257 ) ) ;
#3900=CARTESIAN_POINT ( 'NONE',  ( 158.0000000000011937, 91.09837461714084839, -45.00000000000000000 ) ) ;
#3901=DIRECTION ( 'NONE',  ( 0.8916010070295112833, 0.4528218681379702626, 0.000000000000000000 ) ) ;
#3902=PLANE ( 'NONE',  #6914 ) ;
#3903=VERTEX_POINT ( 'NONE', #7665 ) ;
#3906=CYLINDRICAL_SURFACE ( 'NONE', #24238, 6.000000000000005329 ) ;
#3907=LINE ( 'NONE', #28307, #4613 ) ;
#3908=DIRECTION ( 'NONE',  ( 0.4528218681335642870, 0.8916010070317489378, -0.000000000000000000 ) ) ;
#3910=VECTOR ( 'NONE', #14590, 999.9999999999998863 ) ;
#3912=AXIS2_PLACEMENT_3D ( 'NONE', #18204, #7282, #11887 ) ;
#3913=CARTESIAN_POINT ( 'NONE',  ( 157.4999999999998579, 63.25781203080982351, -45.00000000000000000 ) ) ;
#3914=LINE ( 'NONE', #15133, #13940 ) ;
#3921=EDGE_CURVE ( 'NONE', #1653, #4329, #14840, .T. ) ;
#3922=ADVANCED_FACE ( 'NONE', ( #12548 ), #7801, .F. ) ;
#3926=EDGE_LOOP ( 'NONE', ( #4495, #12001, #18599, #329 ) ) ;
#3927=ADVANCED_FACE ( 'NONE', ( #1189 ), #27743, .F. ) ;
#3935=LINE ( 'NONE', #7975, #16766 ) ;
#3943=DIRECTION ( 'NONE',  ( 1.000000000000000000, 0.000000000000000000, -0.000000000000000000 ) ) ;
#3944=CARTESIAN_POINT ( 'NONE',  ( 157.9999999999998579, 221.5078750075070104, 45.00000000000000000 ) ) ;
#3946=CARTESIAN_POINT ( 'NONE',  ( 158.0000000000011937, 91.09837461714084839, 45.00000000000000000 ) ) ;
#3958=CARTESIAN_POINT ( 'NONE',  ( 157.4999999999996874, 266.3956876388795649, -45.00000000000000000 ) ) ;
#3959=ORIENTED_EDGE ( 'NONE', *, *, #6027, .F. ) ;
#3962=ORIENTED_EDGE ( 'NONE', *, *, #22705, .F. ) ;
#3966=EDGE_LOOP ( 'NONE', ( #11123, #5162, #4735, #15504 ) ) ;
#3980=ORIENTED_EDGE ( 'NONE', *, *, #18992, .T. ) ;
#3982=PLANE ( 'NONE',  #26133 ) ;
#3983=DIRECTION ( 'NONE',  ( -0.8916010070293383105, -0.4528218681383106015, 0.000000000000000000 ) ) ;
#3987=EDGE_LOOP ( 'NONE', ( #39, #13071, #2395, #4610 ) ) ;
#3991=EDGE_CURVE ( 'NONE', #10126, #21270, #12690, .T. ) ;
#3997=EDGE_CURVE ( 'NONE', #2768, #11694, #14692, .T. ) ;
#3998=ORIENTED_EDGE ( 'NONE', *, *, #28211, .T. ) ;
#4002=CARTESIAN_POINT ( 'NONE',  ( 158.0000000000007105, 138.2401247522676044, 45.00000000000000000 ) ) ;
#4003=DIRECTION ( 'NONE',  ( -0.000000000000000000, 0.000000000000000000, -1.000000000000000000 ) ) ;
#4006=DIRECTION ( 'NONE',  ( 1.000000000000000000, 0.000000000000000000, -0.000000000000000000 ) ) ;
#4007=VECTOR ( 'NONE', #22680, 1000.000000000000000 ) ;
#4013=ORIENTED_EDGE ( 'NONE', *, *, #9061, .F. ) ;
#4015=ADVANCED_FACE ( 'NONE', ( #18853 ), #1608, .F. ) ;
#4016=ADVANCED_FACE ( 'NONE', ( #10377 ), #25591, .F. ) ;
#4018=ORIENTED_EDGE ( 'NONE', *, *, #18662, .T. ) ;
#4020=ORIENTED_EDGE ( 'NONE', *, *, #16246, .T. ) ;
#4022=VECTOR ( 'NONE', #23990, 1000.000000000000000 ) ;
#4024=DIRECTION ( 'NONE',  ( 0.8916010070293283185, 0.4528218681383305855, 0.000000000000000000 ) ) ;
#4030=EDGE_CURVE ( 'NONE', #9386, #18364, #25734, .T. ) ;
#4032=CARTESIAN_POINT ( 'NONE',  ( 158.0000000000007105, 138.2401247522676044, 45.00000000000000000 ) ) ;
#4033=ORIENTED_EDGE ( 'NONE', *, *, #2219, .F. ) ;
#4039=DIRECTION ( 'NONE',  ( -0.000000000000000000, 0.000000000000000000, -1.000000000000000000 ) ) ;
#4040=DIRECTION ( 'NONE',  ( 0.8916010070293584056, -0.4528218681382712996, 0.000000000000000000 ) ) ;
#4041=VECTOR ( 'NONE', #25504, 1000.000000000000000 ) ;
#4042=VERTEX_POINT ( 'NONE', #12827 ) ;
#4044=AXIS2_PLACEMENT_3D ( 'NONE', #24192, #22178, #21891 ) ;
#4048=ORIENTED_EDGE ( 'NONE', *, *, #12709, .T. ) ;
#4049=CARTESIAN_POINT ( 'NONE',  ( 157.4999999999994600, 213.7303124812313513, 45.00000000000000000 ) ) ;
#4051=DIRECTION ( 'NONE',  ( 0.8916010070293383105, -0.4528218681383106015, 0.000000000000000000 ) ) ;
#4058=LINE ( 'NONE', #12848, #3750 ) ;
#4063=LINE ( 'NONE', #26458, #24164 ) ;
#4064=ORIENTED_EDGE ( 'NONE', *, *, #16923, .T. ) ;
#4070=ORIENTED_EDGE ( 'NONE', *, *, #8217, .F. ) ;
#4071=ORIENTED_EDGE ( 'NONE', *, *, #14135, .F. ) ;
#4073=VECTOR ( 'NONE', #6904, 1000.000000000000000 ) ;
#4076=CARTESIAN_POINT ( 'NONE',  ( 158.0000000000000284, 205.9527499549551806, -45.00000000000000000 ) ) ;
#4082=ADVANCED_FACE ( 'NONE', ( #6340 ), #15122, .F. ) ;
#4085=VECTOR ( 'NONE', #10734, 1000.000000000000000 ) ;
#4086=CARTESIAN_POINT ( 'NONE',  ( 157.9999999999997158, 261.1260001201120531, 45.00000000000000000 ) ) ;
#4087=DIRECTION ( 'NONE',  ( 0.000000000000000000, -1.000000000000000000, 0.000000000000000000 ) ) ;
#4089=ORIENTED_EDGE ( 'NONE', *, *, #25864, .F. ) ;
#4090=LINE ( 'NONE', #18900, #17827 ) ;
#4091=VECTOR ( 'NONE', #5721, 1000.000000000000000 ) ;
#4094=CARTESIAN_POINT ( 'NONE',  ( 157.9999999999998295, 228.5236250225210313, -45.00000000000000000 ) ) ;
#4096=CARTESIAN_POINT ( 'NONE',  ( 157.4999999999998579, 85.82868709837320864, 45.00000000000000000 ) ) ;
#4098=VECTOR ( 'NONE', #16114, 1000.000000000000227 ) ;
#4103=VERTEX_POINT ( 'NONE', #20271 ) ;
#4106=ADVANCED_FACE ( 'NONE', ( #22577 ), #876, .F. ) ;
#4109=ORIENTED_EDGE ( 'NONE', *, *, #9554, .T. ) ;
#4110=PLANE ( 'NONE',  #9070 ) ;
#4112=DIRECTION ( 'NONE',  ( -0.000000000000000000, -0.000000000000000000, -1.000000000000000000 ) ) ;
#4114=CARTESIAN_POINT ( 'NONE',  ( 158.0000000000004832, 163.3188748273380213, 45.00000000000000000 ) ) ;
#4119=DIRECTION ( 'NONE',  ( -0.000000000000000000, -0.000000000000000000, -1.000000000000000000 ) ) ;
#4120=DIRECTION ( 'NONE',  ( -0.000000000000000000, 0.000000000000000000, -1.000000000000000000 ) ) ;
#4126=LINE ( 'NONE', #1828, #456 ) ;
#4136=ORIENTED_EDGE ( 'NONE', *, *, #18117, .T. ) ;
#4140=ORIENTED_EDGE ( 'NONE', *, *, #23688, .F. ) ;
#4142=VECTOR ( 'NONE', #16154, 1000.000000000000000 ) ;
#4149=DIRECTION ( 'NONE',  ( 0.000000000000000000, -1.000000000000000000, 0.000000000000000000 ) ) ;
#4151=ADVANCED_FACE ( 'NONE', ( #27291 ), #16397, .F. ) ;
#4153=ADVANCED_FACE ( 'NONE', ( #20688 ), #25142, .F. ) ;
#4156=DIRECTION ( 'NONE',  ( 0.8916010070298462376, 0.4528218681373109011, 0.000000000000000000 ) ) ;
#4157=ORIENTED_EDGE ( 'NONE', *, *, #14392, .T. ) ;
#4158=ORIENTED_EDGE ( 'NONE', *, *, #608, .F. ) ;
#4162=VERTEX_POINT ( 'NONE', #18544 ) ;
#4165=ORIENTED_EDGE ( 'NONE', *, *, #25110, .T. ) ;
#4177=CARTESIAN_POINT ( 'NONE',  ( 158.0000000000004547, 163.8267498348450886, 45.00000000000000000 ) ) ;
#4178=EDGE_CURVE ( 'NONE', #25624, #4442, #741, .T. ) ;
#4181=CARTESIAN_POINT ( 'NONE',  ( 157.4999999999998579, 95.86018712840139244, 45.00000000000000000 ) ) ;
#4182=VECTOR ( 'NONE', #791, 1000.000000000000000 ) ;
#4183=EDGE_CURVE ( 'NONE', #14116, #11428, #27016, .T. ) ;
#4187=CARTESIAN_POINT ( 'NONE',  ( 157.4999999999998579, 143.5098122710352015, 45.00000000000000000 ) ) ;
#4189=CARTESIAN_POINT ( 'NONE',  ( 157.4999999999997442, 256.3641876088515232, 45.00000000000000000 ) ) ;
#4190=CARTESIAN_POINT ( 'NONE',  ( 158.0000000000007105, 136.2401247522676044, 45.00000000000000000 ) ) ;
#4191=DIRECTION ( 'NONE',  ( -0.000000000000000000, -0.000000000000000000, -1.000000000000000000 ) ) ;
#4192=ORIENTED_EDGE ( 'NONE', *, *, #16697, .T. ) ;
#4199=LINE ( 'NONE', #18248, #13902 ) ;
#4200=EDGE_LOOP ( 'NONE', ( #8700, #27746, #16871, #2025 ) ) ;
#4201=VECTOR ( 'NONE', #20731, 1000.000000000000000 ) ;
#4202=PLANE ( 'NONE',  #2836 ) ;
#4204=ORIENTED_EDGE ( 'NONE', *, *, #18726, .F. ) ;
#4205=AXIS2_PLACEMENT_3D ( 'NONE', #8103, #12289, #21447 ) ;
#4207=ORIENTED_EDGE ( 'NONE', *, *, #4272, .F. ) ;
#4212=VERTEX_POINT ( 'NONE', #7494 ) ;
#4214=ORIENTED_EDGE ( 'NONE', *, *, #28094, .T. ) ;
#4218=CARTESIAN_POINT ( 'NONE',  ( 157.4999999999998579, 98.36806213590843129, 45.00000000000000000 ) ) ;
#4221=CARTESIAN_POINT ( 'NONE',  ( 157.4999999999998579, 63.25781203080982351, 45.00000000000000000 ) ) ;
#4226=CARTESIAN_POINT ( 'NONE',  ( 158.0000000000006537, 143.7637497747887210, 45.00000000000000000 ) ) ;
#4227=EDGE_CURVE ( 'NONE', #27097, #17151, #458, .T. ) ;
#4228=CARTESIAN_POINT ( 'NONE',  ( 158.0000000000014779, 65.51174953456337846, 45.00000000000000000 ) ) ;
#4230=DIRECTION ( 'NONE',  ( -0.8916010070293783896, 0.4528218681382319422, 0.000000000000000000 ) ) ;
#4235=DIRECTION ( 'NONE',  ( 0.000000000000000000, -1.000000000000000000, 0.000000000000000000 ) ) ;
#4236=FACE_OUTER_BOUND ( 'NONE', #9986, .T. ) ;
#4237=CARTESIAN_POINT ( 'NONE',  ( 158.0000000000007958, 128.7164997297464595, 45.00000000000000000 ) ) ;
#4241=LINE ( 'NONE', #25649, #21237 ) ;
#4243=CARTESIAN_POINT ( 'NONE',  ( 157.4999999999998579, 181.1279373836408411, -45.00000000000000000 ) ) ;
#4244=ORIENTED_EDGE ( 'NONE', *, *, #13892, .F. ) ;
#4245=EDGE_CURVE ( 'NONE', #20893, #3887, #24585, .T. ) ;
#4246=VECTOR ( 'NONE', #12334, 1000.000000000000114 ) ;
#4247=ORIENTED_EDGE ( 'NONE', *, *, #3106, .F. ) ;
#4248=LINE ( 'NONE', #23938, #7166 ) ;
#4250=EDGE_LOOP ( 'NONE', ( #17899, #27, #24146, #6205 ) ) ;
#4256=VECTOR ( 'NONE', #4517, 1000.000000000000000 ) ;
#4257=EDGE_CURVE ( 'NONE', #21319, #8486, #23559, .T. ) ;
#4258=LINE ( 'NONE', #21791, #27727 ) ;
#4259=CARTESIAN_POINT ( 'NONE',  ( 157.4999999999997442, 253.8563126013445697, 45.00000000000000000 ) ) ;
#4260=CARTESIAN_POINT ( 'NONE',  ( 158.0000000000017337, 42.94087446699998623, 45.00000000000000000 ) ) ;
#4267=LINE ( 'NONE', #17059, #24938 ) ;
#4271=ADVANCED_FACE ( 'NONE', ( #10206 ), #23276, .F. ) ;
#4272=EDGE_CURVE ( 'NONE', #18330, #12180, #18818, .T. ) ;
#4273=VECTOR ( 'NONE', #24918, 1000.000000000000000 ) ;
#4275=DIRECTION ( 'NONE',  ( 0.8916010070299679180, 0.4528218681370710930, 0.000000000000000000 ) ) ;
#4278=ORIENTED_EDGE ( 'NONE', *, *, #14915, .F. ) ;
#4280=ORIENTED_EDGE ( 'NONE', *, *, #17709, .F. ) ;
#4282=ORIENTED_EDGE ( 'NONE', *, *, #14945, .F. ) ;
#4285=ORIENTED_EDGE ( 'NONE', *, *, #2794, .T. ) ;
#4287=VERTEX_POINT ( 'NONE', #12374 ) ;
#4288=AXIS2_PLACEMENT_3D ( 'NONE', #15263, #8927, #22138 ) ;
#4290=EDGE_CURVE ( 'NONE', #2965, #18534, #1293, .T. ) ;
#4297=FACE_OUTER_BOUND ( 'NONE', #25874, .T. ) ;
#4300=PLANE ( 'NONE',  #12768 ) ;
#4304=LINE ( 'NONE', #16956, #14750 ) ;
#4308=VECTOR ( 'NONE', #22175, 1000.000000000000000 ) ;
#4310=CARTESIAN_POINT ( 'NONE',  ( 157.9999999999997158, 261.1260001201120531, 45.00000000000000000 ) ) ;
#4312=VECTOR ( 'NONE', #26313, 1000.000000000000227 ) ;
#4314=VERTEX_POINT ( 'NONE', #16811 ) ;
#4323=ORIENTED_EDGE ( 'NONE', *, *, #19214, .T. ) ;
#4329=VERTEX_POINT ( 'NONE', #3580 ) ;
#4330=DIRECTION ( 'NONE',  ( 0.8916010070293584056, 0.4528218681382713551, 0.000000000000000000 ) ) ;
#4333=LINE ( 'NONE', #17694, #6953 ) ;
#4334=CARTESIAN_POINT ( 'NONE',  ( 157.9999999999998579, 221.5078750075070104, -45.00000000000000000 ) ) ;
#4337=ADVANCED_FACE ( 'NONE', ( #23412 ), #1576, .F. ) ;
#4341=ORIENTED_EDGE ( 'NONE', *, *, #386, .T. ) ;
#4342=VECTOR ( 'NONE', #26882, 1000.000000000000114 ) ;
#4346=ADVANCED_FACE ( 'NONE', ( #25704 ), #6025, .F. ) ;
#4348=ORIENTED_EDGE ( 'NONE', *, *, #9095, .T. ) ;
#4352=EDGE_CURVE ( 'NONE', #24036, #6606, #19245, .T. ) ;
#4353=ORIENTED_EDGE ( 'NONE', *, *, #26551, .T. ) ;
#4354=EDGE_LOOP ( 'NONE', ( #10832, #19485, #5666, #12241 ) ) ;
#4359=DIRECTION ( 'NONE',  ( -0.000000000000000000, -0.000000000000000000, -1.000000000000000000 ) ) ;
#4360=DIRECTION ( 'NONE',  ( -0.8916010070297041290, -0.4528218681375906218, 0.000000000000000000 ) ) ;
#4363=DIRECTION ( 'NONE',  ( -0.000000000000000000, -0.000000000000000000, -1.000000000000000000 ) ) ;
#4364=ORIENTED_EDGE ( 'NONE', *, *, #26079, .T. ) ;
#4365=DIRECTION ( 'NONE',  ( -0.8916010070293383105, -0.4528218681383106015, 0.000000000000000000 ) ) ;
#4367=DIRECTION ( 'NONE',  ( 0.000000000000000000, -1.000000000000000000, 0.000000000000000000 ) ) ;
#4368=FACE_OUTER_BOUND ( 'NONE', #3397, .T. ) ;
#4369=CARTESIAN_POINT ( 'NONE',  ( 157.9999999999996589, 271.6653751576470768, 45.00000000000000000 ) ) ;
#4370=ORIENTED_EDGE ( 'NONE', *, *, #10270, .F. ) ;
#4371=LINE ( 'NONE', #24487, #25190 ) ;
#4373=DIRECTION ( 'NONE',  ( 0.4528218681380514754, 0.8916010070294700940, -0.000000000000000000 ) ) ;
#4375=LINE ( 'NONE', #6396, #24854 ) ;
#4378=ADVANCED_FACE ( 'NONE', ( #5461 ), #3298, .F. ) ;
#4380=ORIENTED_EDGE ( 'NONE', *, *, #11326, .T. ) ;
#4382=ORIENTED_EDGE ( 'NONE', *, *, #19112, .T. ) ;
#4387=PLANE ( 'NONE',  #10378 ) ;
#4388=EDGE_CURVE ( 'NONE', #22451, #3081, #1998, .T. ) ;
#4389=VERTEX_POINT ( 'NONE', #14948 ) ;
#4391=AXIS2_PLACEMENT_3D ( 'NONE', #4538, #13051, #11162 ) ;
#4392=VERTEX_POINT ( 'NONE', #11201 ) ;
#4397=PLANE ( 'NONE',  #27493 ) ;
#4401=PLANE ( 'NONE',  #19570 ) ;
#4402=CARTESIAN_POINT ( 'NONE',  ( 157.4999999999998579, 55.73418700828869277, 45.00000000000000000 ) ) ;
#4403=PLANE ( 'NONE',  #26656 ) ;
#4404=CARTESIAN_POINT ( 'NONE',  ( 157.9999999999998295, 226.0157500150140208, 45.00000000000000000 ) ) ;
#4405=LINE ( 'NONE', #21507, #26296 ) ;
#4406=AXIS2_PLACEMENT_3D ( 'NONE', #2368, #231, #15609 ) ;
#4408=LINE ( 'NONE', #20061, #24819 ) ;
#4413=VERTEX_POINT ( 'NONE', #2418 ) ;
#4417=CARTESIAN_POINT ( 'NONE',  ( 158.0000000000012790, 83.57474959461971764, 45.00000000000000000 ) ) ;
#4421=ORIENTED_EDGE ( 'NONE', *, *, #21725, .T. ) ;
#4425=EDGE_CURVE ( 'NONE', #11428, #13449, #287, .T. ) ;
#4426=EDGE_CURVE ( 'NONE', #9458, #11694, #17657, .T. ) ;
#4427=LINE ( 'NONE', #8890, #5944 ) ;
#4431=FACE_OUTER_BOUND ( 'NONE', #7617, .T. ) ;
#4433=FACE_OUTER_BOUND ( 'NONE', #5415, .T. ) ;
#4434=DIRECTION ( 'NONE',  ( 0.000000000000000000, -1.000000000000000000, 0.000000000000000000 ) ) ;
#4436=EDGE_CURVE ( 'NONE', #8166, #4103, #9043, .T. ) ;
#4437=ADVANCED_FACE ( 'NONE', ( #26411 ), #21832, .F. ) ;
#4441=DIRECTION ( 'NONE',  ( 1.000000000000000000, -0.000000000000000000, -0.000000000000000000 ) ) ;
#4442=VERTEX_POINT ( 'NONE', #6171 ) ;
#4451=DIRECTION ( 'NONE',  ( -0.8916010070297542001, 0.4528218681374919785, 0.000000000000000000 ) ) ;
#4452=DIRECTION ( 'NONE',  ( -0.8916010070293283185, -0.4528218681383305855, 0.000000000000000000 ) ) ;
#4453=ORIENTED_EDGE ( 'NONE', *, *, #7211, .F. ) ;
#4455=CARTESIAN_POINT ( 'NONE',  ( 158.0000000000003411, 173.8582498648732440, 45.00000000000000000 ) ) ;
#4456=ORIENTED_EDGE ( 'NONE', *, *, #12321, .T. ) ;
#4460=FACE_OUTER_BOUND ( 'NONE', #22710, .T. ) ;
#4462=ORIENTED_EDGE ( 'NONE', *, *, #6713, .F. ) ;
#4467=ORIENTED_EDGE ( 'NONE', *, *, #4257, .F. ) ;
#4468=ADVANCED_FACE ( 'NONE', ( #23701 ), #4300, .F. ) ;
#4471=AXIS2_PLACEMENT_3D ( 'NONE', #19534, #2138, #6734 ) ;
#4476=ORIENTED_EDGE ( 'NONE', *, *, #13852, .F. ) ;
#4479=VERTEX_POINT ( 'NONE', #12934 ) ;
#4483=VECTOR ( 'NONE', #21947, 1000.000000000000114 ) ;
#4485=ORIENTED_EDGE ( 'NONE', *, *, #276, .T. ) ;
#4488=CIRCLE ( 'NONE', #4954, 6.000000000000005329 ) ;
#4491=CARTESIAN_POINT ( 'NONE',  ( 158.0000000000014211, 70.52749954957745615, 45.00000000000000000 ) ) ;
#4492=CARTESIAN_POINT ( 'NONE',  ( 158.0000000000000284, 205.9527499549551806, 45.00000000000000000 ) ) ;
#4494=FACE_OUTER_BOUND ( 'NONE', #13436, .T. ) ;
#4495=ORIENTED_EDGE ( 'NONE', *, *, #8739, .T. ) ;
#4498=EDGE_CURVE ( 'NONE', #14755, #19061, #10914, .T. ) ;
#4500=DIRECTION ( 'NONE',  ( 0.8916010070297345491, 0.4528218681375306698, 0.000000000000000000 ) ) ;
#4501=LINE ( 'NONE', #8972, #25399 ) ;
#4505=EDGE_CURVE ( 'NONE', #4212, #27414, #17508, .T. ) ;
#4507=VECTOR ( 'NONE', #8333, 1000.000000000000000 ) ;
#4508=EDGE_CURVE ( 'NONE', #19398, #22237, #2277, .T. ) ;
#4512=ORIENTED_EDGE ( 'NONE', *, *, #23837, .F. ) ;
#4513=LINE ( 'NONE', #19612, #6035 ) ;
#4517=DIRECTION ( 'NONE',  ( -0.000000000000000000, -0.000000000000000000, -1.000000000000000000 ) ) ;
#4518=ORIENTED_EDGE ( 'NONE', *, *, #9974, .T. ) ;
#4522=ORIENTED_EDGE ( 'NONE', *, *, #13546, .T. ) ;
#4523=LINE ( 'NONE', #13310, #21391 ) ;
#4530=CARTESIAN_POINT ( 'NONE',  ( 157.4999999999996589, 273.9193126614005678, 45.00000000000000000 ) ) ;
#4531=EDGE_CURVE ( 'NONE', #21598, #583, #8617, .T. ) ;
#4536=DIRECTION ( 'NONE',  ( 1.000000000000000000, 0.000000000000000000, -0.000000000000000000 ) ) ;
#4538=CARTESIAN_POINT ( 'NONE',  ( 157.9999999999997442, 256.1102501050980322, 45.00000000000000000 ) ) ;
#4540=LINE ( 'NONE', #15626, #22995 ) ;
#4543=ORIENTED_EDGE ( 'NONE', *, *, #1867, .T. ) ;
#4548=CARTESIAN_POINT ( 'NONE',  ( 157.9999999999997442, 251.6023750975910218, 45.00000000000000000 ) ) ;
#4549=FACE_OUTER_BOUND ( 'NONE', #12039, .T. ) ;
#4553=DIRECTION ( 'NONE',  ( 0.8916010070290389944, -0.4528218681389001854, 0.000000000000000000 ) ) ;
#4556=ORIENTED_EDGE ( 'NONE', *, *, #4352, .T. ) ;
#4557=AXIS2_PLACEMENT_3D ( 'NONE', #482, #628, #13708 ) ;
#4558=ORIENTED_EDGE ( 'NONE', *, *, #1454, .F. ) ;
#4569=DIRECTION ( 'NONE',  ( 0.000000000000000000, -1.000000000000000000, 0.000000000000000000 ) ) ;
#4573=DIRECTION ( 'NONE',  ( -0.000000000000000000, -0.000000000000000000, -1.000000000000000000 ) ) ;
#4577=AXIS2_PLACEMENT_3D ( 'NONE', #5968, #16756, #1237 ) ;
#4580=LINE ( 'NONE', #11205, #9247 ) ;
#4587=LINE ( 'NONE', #13232, #16771 ) ;
#4591=DIRECTION ( 'NONE',  ( 0.4528218681382319422, -0.8916010070293783896, 0.000000000000000000 ) ) ;
#4597=EDGE_CURVE ( 'NONE', #16382, #8245, #20384, .T. ) ;
#4602=EDGE_CURVE ( 'NONE', #12113, #22238, #26549, .T. ) ;
#4605=ORIENTED_EDGE ( 'NONE', *, *, #12094, .F. ) ;
#4606=CARTESIAN_POINT ( 'NONE',  ( 157.4999999999998579, 63.25781203080982351, -45.00000000000000000 ) ) ;
#4609=CARTESIAN_POINT ( 'NONE',  ( 158.0000000000000853, 196.4291249324366504, 45.00000000000000000 ) ) ;
#4610=ORIENTED_EDGE ( 'NONE', *, *, #14135, .T. ) ;
#4612=ADVANCED_FACE ( 'NONE', ( #7028 ), #26850, .F. ) ;
#4613=VECTOR ( 'NONE', #12978, 1000.000000000000114 ) ;
#4616=CARTESIAN_POINT ( 'NONE',  ( 157.4999999999998579, 141.0019372635281627, -45.00000000000000000 ) ) ;
#4617=VERTEX_POINT ( 'NONE', #24698 ) ;
#4618=( NAMED_UNIT ( * ) PLANE_ANGLE_UNIT ( ) SI_UNIT ( $, .RADIAN. ) );
#4619=VERTEX_POINT ( 'NONE', #713 ) ;
#4620=LINE ( 'NONE', #19860, #10635 ) ;
#4621=CARTESIAN_POINT ( 'NONE',  ( 157.4999999999998579, 151.0334372935563465, 45.00000000000000000 ) ) ;
#4623=VERTEX_POINT ( 'NONE', #9482 ) ;
#4625=DIRECTION ( 'NONE',  ( -0.8916010070293383105, -0.4528218681383106015, 0.000000000000000000 ) ) ;
#4634=ADVANCED_FACE ( 'NONE', ( #20525 ), #7462, .F. ) ;
#4635=DIRECTION ( 'NONE',  ( -0.000000000000000000, -0.000000000000000000, -1.000000000000000000 ) ) ;
#4637=LINE ( 'NONE', #27952, #13713 ) ;
#4640=ORIENTED_EDGE ( 'NONE', *, *, #3119, .T. ) ;
#4644=CARTESIAN_POINT ( 'NONE',  ( 158.0000000000005684, 151.2873747973098659, 45.00000000000000000 ) ) ;
#4647=VERTEX_POINT ( 'NONE', #24981 ) ;
#4648=VECTOR ( 'NONE', #27787, 999.9999999999998863 ) ;
#4657=VERTEX_POINT ( 'NONE', #24553 ) ;
#4663=ORIENTED_EDGE ( 'NONE', *, *, #15827, .F. ) ;
#4664=ORIENTED_EDGE ( 'NONE', *, *, #8488, .T. ) ;
#4665=CARTESIAN_POINT ( 'NONE',  ( 158.0000000000006537, 145.7637497747887210, 45.00000000000000000 ) ) ;
#4666=EDGE_LOOP ( 'NONE', ( #24349, #9197, #9281, #2051 ) ) ;
#4668=EDGE_LOOP ( 'NONE', ( #27210, #5943, #23758, #8744 ) ) ;
#4672=VECTOR ( 'NONE', #19004, 1000.000000000000000 ) ;
#4674=CARTESIAN_POINT ( 'NONE',  ( 157.4999999999998579, 158.5570623160774630, 45.00000000000000000 ) ) ;
#4681=DIRECTION ( 'NONE',  ( 1.000000000000000000, 0.000000000000000000, -0.000000000000000000 ) ) ;
#4682=CARTESIAN_POINT ( 'NONE',  ( 158.0000000000015916, 53.48024950453520177, 45.00000000000000000 ) ) ;
#4690=ORIENTED_EDGE ( 'NONE', *, *, #6020, .F. ) ;
#4692=VECTOR ( 'NONE', #19679, 1000.000000000000000 ) ;
#4700=ORIENTED_EDGE ( 'NONE', *, *, #26969, .F. ) ;
#4706=LINE ( 'NONE', #22386, #18014 ) ;
#4709=FACE_OUTER_BOUND ( 'NONE', #16659, .T. ) ;
#4710=LINE ( 'NONE', #13496, #18511 ) ;
#4711=VECTOR ( 'NONE', #10695, 1000.000000000000114 ) ;
#4713=CARTESIAN_POINT ( 'NONE',  ( 157.4999999999998579, 98.36806213590843129, 45.00000000000000000 ) ) ;
#4714=FACE_OUTER_BOUND ( 'NONE', #3139, .T. ) ;
#4716=LINE ( 'NONE', #13500, #27780 ) ;
#4719=CARTESIAN_POINT ( 'NONE',  ( 157.4999999999998579, 115.9231871884577174, 45.00000000000000000 ) ) ;
#4721=AXIS2_PLACEMENT_3D ( 'NONE', #22669, #14189, #9870 ) ;
#4723=DIRECTION ( 'NONE',  ( 0.4528218681376112720, 0.8916010070296936929, -0.000000000000000000 ) ) ;
#4724=CARTESIAN_POINT ( 'NONE',  ( 158.0000000000009379, 118.1771246922112653, 45.00000000000000000 ) ) ;
#4727=ORIENTED_EDGE ( 'NONE', *, *, #19536, .F. ) ;
#4733=ORIENTED_EDGE ( 'NONE', *, *, #22007, .T. ) ;
#4735=ORIENTED_EDGE ( 'NONE', *, *, #20897, .F. ) ;
#4740=VERTEX_POINT ( 'NONE', #3269 ) ;
#4741=VECTOR ( 'NONE', #24665, 1000.000000000000000 ) ;
#4742=VERTEX_POINT ( 'NONE', #7875 ) ;
#4743=DIRECTION ( 'NONE',  ( -0.8916010070298961976, 0.4528218681372121468, 0.000000000000000000 ) ) ;
#4748=CARTESIAN_POINT ( 'NONE',  ( 157.9999999999996589, 273.6653751576470768, -45.00000000000000000 ) ) ;
#4750=CARTESIAN_POINT ( 'NONE',  ( 157.9999999999999147, 213.9842499849850697, 45.00000000000000000 ) ) ;
#4753=AXIS2_PLACEMENT_3D ( 'NONE', #17156, #3795, #6377 ) ;
#4754=ORIENTED_EDGE ( 'NONE', *, *, #19042, .T. ) ;
#4755=CARTESIAN_POINT ( 'NONE',  ( 157.4999999999998579, 156.0491873085704242, 45.00000000000000000 ) ) ;
#4758=VECTOR ( 'NONE', #8691, 1000.000000000000114 ) ;
#4768=EDGE_CURVE ( 'NONE', #22350, #1387, #14631, .T. ) ;
#4769=CARTESIAN_POINT ( 'NONE',  ( 157.4999999999998010, 236.3011875487955251, 45.00000000000000000 ) ) ;
#4771=ORIENTED_EDGE ( 'NONE', *, *, #20496, .F. ) ;
#4772=EDGE_LOOP ( 'NONE', ( #17952, #10584, #25831, #2581 ) ) ;
#4779=ADVANCED_FACE ( 'NONE', ( #27819 ), #27395, .F. ) ;
#4780=EDGE_CURVE ( 'NONE', #2799, #11964, #27681, .T. ) ;
#4782=CARTESIAN_POINT ( 'NONE',  ( 158.0000000000005684, 153.2873747973098659, 45.00000000000000000 ) ) ;
#4784=FACE_OUTER_BOUND ( 'NONE', #15835, .T. ) ;
#4789=DIRECTION ( 'NONE',  ( 0.000000000000000000, -1.000000000000000000, 0.000000000000000000 ) ) ;
#4790=DIRECTION ( 'NONE',  ( -1.850371707708594366E-15, -1.000000000000000000, 0.000000000000000000 ) ) ;
#4793=VECTOR ( 'NONE', #9366, 1000.000000000000000 ) ;
#4794=ADVANCED_FACE ( 'NONE', ( #5998 ), #21085, .F. ) ;
#4795=DIRECTION ( 'NONE',  ( 0.4528218681379715949, 0.8916010070295107282, -0.000000000000000000 ) ) ;
#4796=ORIENTED_EDGE ( 'NONE', *, *, #6909, .F. ) ;
#4801=ORIENTED_EDGE ( 'NONE', *, *, #816, .F. ) ;
#4807=DIRECTION ( 'NONE',  ( 0.8916010070295213863, 0.4528218681379503341, 0.000000000000000000 ) ) ;
#4809=ADVANCED_FACE ( 'NONE', ( #2107 ), #25962, .F. ) ;
#4812=VERTEX_POINT ( 'NONE', #13055 ) ;
#4819=VECTOR ( 'NONE', #13938, 1000.000000000000000 ) ;
#4825=DIRECTION ( 'NONE',  ( -0.000000000000000000, -0.000000000000000000, -1.000000000000000000 ) ) ;
#4826=DIRECTION ( 'NONE',  ( -0.000000000000000000, -0.000000000000000000, -1.000000000000000000 ) ) ;
#4827=PLANE ( 'NONE',  #24851 ) ;
#4832=FACE_OUTER_BOUND ( 'NONE', #8951, .T. ) ;
#4834=VECTOR ( 'NONE', #26465, 1000.000000000000000 ) ;
#4835=CARTESIAN_POINT ( 'NONE',  ( 158.0000000000009663, 111.1613746771971876, 45.00000000000000000 ) ) ;
#4837=VECTOR ( 'NONE', #6279, 1000.000000000000000 ) ;
#4838=EDGE_CURVE ( 'NONE', #19459, #14606, #21934, .T. ) ;
#4840=ORIENTED_EDGE ( 'NONE', *, *, #24958, .T. ) ;
#4844=VERTEX_POINT ( 'NONE', #8589 ) ;
#4849=DIRECTION ( 'NONE',  ( -0.000000000000000000, -0.000000000000000000, -1.000000000000000000 ) ) ;
#4850=PLANE ( 'NONE',  #14666 ) ;
#4854=CARTESIAN_POINT ( 'NONE',  ( 157.9999999999997442, 249.0945000900840398, 45.00000000000000000 ) ) ;
#4856=CARTESIAN_POINT ( 'NONE',  ( 157.9999999999998863, 216.4921249924925348, 45.00000000000000000 ) ) ;
#4857=DIRECTION ( 'NONE',  ( 0.8916010070293384215, 0.4528218681383106015, 0.000000000000000000 ) ) ;
#4861=VECTOR ( 'NONE', #12126, 999.9999999999998863 ) ;
#4863=LINE ( 'NONE', #6341, #22982 ) ;
#4867=DIRECTION ( 'NONE',  ( 0.000000000000000000, -1.000000000000000000, 0.000000000000000000 ) ) ;
#4868=ADVANCED_FACE ( 'NONE', ( #19355 ), #1965, .F. ) ;
#4870=ORIENTED_EDGE ( 'NONE', *, *, #7098, .F. ) ;
#4872=LINE ( 'NONE', #7329, #1805 ) ;
#4875=CARTESIAN_POINT ( 'NONE',  ( 157.4999999999998579, 163.5728123310915407, 45.00000000000000000 ) ) ;
#4879=ORIENTED_EDGE ( 'NONE', *, *, #10062, .F. ) ;
#4884=VERTEX_POINT ( 'NONE', #6569 ) ;
#4885=VERTEX_POINT ( 'NONE', #8864 ) ;
#4887=DIRECTION ( 'NONE',  ( 0.8916010070298151513, -0.4528218681373720744, 0.000000000000000000 ) ) ;
#4888=ORIENTED_EDGE ( 'NONE', *, *, #2763, .F. ) ;
#4890=DIRECTION ( 'NONE',  ( 0.8916010070293584056, -0.4528218681382712996, 0.000000000000000000 ) ) ;
#4891=PLANE ( 'NONE',  #21767 ) ;
#4893=AXIS2_PLACEMENT_3D ( 'NONE', #7966, #21031, #23615 ) ;
#4895=EDGE_CURVE ( 'NONE', #6513, #905, #17627, .T. ) ;
#4898=DIRECTION ( 'NONE',  ( -0.000000000000000000, -0.000000000000000000, -1.000000000000000000 ) ) ;
#4901=DIRECTION ( 'NONE',  ( -0.8916010070293584056, -0.4528218681382712996, 0.000000000000000000 ) ) ;
#4902=VERTEX_POINT ( 'NONE', #23958 ) ;
#4908=EDGE_LOOP ( 'NONE', ( #16731, #13620, #20336, #8023 ) ) ;
#4911=ORIENTED_EDGE ( 'NONE', *, *, #9709, .T. ) ;
#4912=AXIS2_PLACEMENT_3D ( 'NONE', #17822, #20117, #4743 ) ;
#4913=ORIENTED_EDGE ( 'NONE', *, *, #24214, .T. ) ;
#4917=CARTESIAN_POINT ( 'NONE',  ( 157.9999999999998579, 223.5078750075070104, 45.00000000000000000 ) ) ;
#4921=CARTESIAN_POINT ( 'NONE',  ( 157.9999999999997442, 256.1102501050980322, 45.00000000000000000 ) ) ;
#4924=DIRECTION ( 'NONE',  ( -0.000000000000000000, 0.000000000000000000, -1.000000000000000000 ) ) ;
#4925=DIRECTION ( 'NONE',  ( 0.000000000000000000, -1.000000000000000000, 0.000000000000000000 ) ) ;
#4933=AXIS2_PLACEMENT_3D ( 'NONE', #17932, #699, #13348 ) ;
#4935=LINE ( 'NONE', #23037, #3628 ) ;
#4938=PLANE ( 'NONE',  #10539 ) ;
#4941=DIRECTION ( 'NONE',  ( 1.000000000000000000, 0.000000000000000000, -0.000000000000000000 ) ) ;
#4943=ORIENTED_EDGE ( 'NONE', *, *, #2856, .T. ) ;
#4951=CARTESIAN_POINT ( 'NONE',  ( 158.0000000000011084, 100.6219996396619791, 45.00000000000000000 ) ) ;
#4954=AXIS2_PLACEMENT_3D ( 'NONE', #17726, #13017, #62 ) ;
#4959=EDGE_CURVE ( 'NONE', #5337, #26387, #6845, .T. ) ;
#4962=CARTESIAN_POINT ( 'NONE',  ( 158.0000000000000853, 198.9369999399436892, 45.00000000000000000 ) ) ;
#4968=DIRECTION ( 'NONE',  ( 0.8916010070293710621, -0.4528218681382463195, 0.000000000000000000 ) ) ;
#4970=CARTESIAN_POINT ( 'NONE',  ( 157.9999999999998295, 226.5236250225210313, -45.00000000000000000 ) ) ;
#4972=DIRECTION ( 'NONE',  ( 0.8916010070293584056, -0.4528218681382712996, 0.000000000000000000 ) ) ;
#4976=FACE_OUTER_BOUND ( 'NONE', #15902, .T. ) ;
#4979=EDGE_CURVE ( 'NONE', #13140, #15105, #22512, .T. ) ;
#4984=ORIENTED_EDGE ( 'NONE', *, *, #5174, .T. ) ;
#4987=ORIENTED_EDGE ( 'NONE', *, *, #7431, .T. ) ;
#4988=EDGE_LOOP ( 'NONE', ( #26715, #14255, #27110, #24104 ) ) ;
#4996=DIRECTION ( 'NONE',  ( -0.000000000000000000, -0.000000000000000000, -1.000000000000000000 ) ) ;
#4997=VECTOR ( 'NONE', #28015, 1000.000000000000000 ) ;
#4998=EDGE_CURVE ( 'NONE', #26005, #10330, #6990, .T. ) ;
#5008=VECTOR ( 'NONE', #2315, 1000.000000000000114 ) ;
#5012=LINE ( 'NONE', #11061, #8772 ) ;
#5015=VERTEX_POINT ( 'NONE', #18206 ) ;
#5017=VECTOR ( 'NONE', #24239, 1000.000000000000000 ) ;
#5018=FACE_OUTER_BOUND ( 'NONE', #15674, .T. ) ;
#5020=ORIENTED_EDGE ( 'NONE', *, *, #418, .T. ) ;
#5026=VERTEX_POINT ( 'NONE', #22657 ) ;
#5028=CARTESIAN_POINT ( 'NONE',  ( 157.4999999999998579, 198.6830624361901414, 45.00000000000000000 ) ) ;
#5030=FACE_OUTER_BOUND ( 'NONE', #13558, .T. ) ;
#5031=ORIENTED_EDGE ( 'NONE', *, *, #486, .T. ) ;
#5036=VECTOR ( 'NONE', #23355, 1000.000000000000000 ) ;
#5037=ADVANCED_FACE ( 'NONE', ( #2384 ), #25151, .F. ) ;
#5043=DIRECTION ( 'NONE',  ( -0.000000000000000000, 0.000000000000000000, -1.000000000000000000 ) ) ;
#5054=DIRECTION ( 'NONE',  ( 0.000000000000000000, -1.000000000000000000, 0.000000000000000000 ) ) ;
#5060=EDGE_CURVE ( 'NONE', #6335, #7010, #9008, .T. ) ;
#5065=VERTEX_POINT ( 'NONE', #4682 ) ;
#5066=DIRECTION ( 'NONE',  ( 0.4528218681382912836, -0.8916010070293483025, 0.000000000000000000 ) ) ;
#5068=VECTOR ( 'NONE', #17295, 1000.000000000000000 ) ;
#5070=CARTESIAN_POINT ( 'NONE',  ( 158.0000000000010800, 103.1298746471690038, 45.00000000000000000 ) ) ;
#5071=DIRECTION ( 'NONE',  ( -0.000000000000000000, 0.000000000000000000, -1.000000000000000000 ) ) ;
#5073=LINE ( 'NONE', #15874, #26076 ) ;
#5076=DIRECTION ( 'NONE',  ( -0.000000000000000000, -0.000000000000000000, -1.000000000000000000 ) ) ;
#5078=EDGE_LOOP ( 'NONE', ( #10692, #15290, #14872, #333 ) ) ;
#5079=CARTESIAN_POINT ( 'NONE',  ( 157.4999999999998579, 103.3838121509225090, 45.00000000000000000 ) ) ;
#5081=DIRECTION ( 'NONE',  ( -0.8916010070295820045, 0.4528218681378310406, 0.000000000000000000 ) ) ;
#5087=CARTESIAN_POINT ( 'NONE',  ( 157.4999999999997726, 246.3326875788235384, 45.00000000000000000 ) ) ;
#5089=VERTEX_POINT ( 'NONE', #9583 ) ;
#5092=ORIENTED_EDGE ( 'NONE', *, *, #3991, .T. ) ;
#5095=VERTEX_POINT ( 'NONE', #2816 ) ;
#5096=CARTESIAN_POINT ( 'NONE',  ( 157.4999999999994884, 211.2224374737238577, 45.00000000000000000 ) ) ;
#5097=EDGE_LOOP ( 'NONE', ( #23585, #24538, #1561, #3389 ) ) ;
#5101=EDGE_LOOP ( 'NONE', ( #27031, #15018, #23939, #19051 ) ) ;
#5104=ORIENTED_EDGE ( 'NONE', *, *, #22981, .T. ) ;
#5105=CARTESIAN_POINT ( 'NONE',  ( 158.0000000000002842, 178.8739998798873216, 45.00000000000000000 ) ) ;
#5106=ADVANCED_FACE ( 'NONE', ( #15917 ), #24664, .F. ) ;
#5107=PLANE ( 'NONE',  #1594 ) ;
#5110=DIRECTION ( 'NONE',  ( 0.000000000000000000, -1.000000000000000000, 0.000000000000000000 ) ) ;
#5112=EDGE_CURVE ( 'NONE', #13671, #25239, #1091, .T. ) ;
#5122=AXIS2_PLACEMENT_3D ( 'NONE', #4835, #22372, #2683 ) ;
#5125=CARTESIAN_POINT ( 'NONE',  ( 157.9999999999998863, 216.4921249924925348, 45.00000000000000000 ) ) ;
#5127=AXIS2_PLACEMENT_3D ( 'NONE', #27053, #14140, #5221 ) ;
#5129=DIRECTION ( 'NONE',  ( 0.4528218681372721544, 0.8916010070298658885, -0.000000000000000000 ) ) ;
#5130=ORIENTED_EDGE ( 'NONE', *, *, #11875, .F. ) ;
#5134=VECTOR ( 'NONE', #10708, 1000.000000000000000 ) ;
#5135=ORIENTED_EDGE ( 'NONE', *, *, #19792, .T. ) ;
#5136=ORIENTED_EDGE ( 'NONE', *, *, #7953, .F. ) ;
#5141=LINE ( 'NONE', #271, #5620 ) ;
#5142=VECTOR ( 'NONE', #14747, 1000.000000000000114 ) ;
#5145=DIRECTION ( 'NONE',  ( 1.000000000000000000, 0.000000000000000000, -0.000000000000000000 ) ) ;
#5148=DIRECTION ( 'NONE',  ( 0.8916010070298252543, -0.4528218681373520904, 0.000000000000000000 ) ) ;
#5152=FACE_OUTER_BOUND ( 'NONE', #6286, .T. ) ;
#5162=ORIENTED_EDGE ( 'NONE', *, *, #4227, .F. ) ;
#5170=EDGE_CURVE ( 'NONE', #16458, #14195, #16752, .T. ) ;
#5171=DIRECTION ( 'NONE',  ( -0.000000000000000000, -0.000000000000000000, -1.000000000000000000 ) ) ;
#5173=ORIENTED_EDGE ( 'NONE', *, *, #9225, .T. ) ;
#5174=EDGE_CURVE ( 'NONE', #7228, #16274, #14595, .T. ) ;
#5175=ORIENTED_EDGE ( 'NONE', *, *, #15329, .T. ) ;
#5176=FACE_OUTER_BOUND ( 'NONE', #3288, .T. ) ;
#5177=AXIS2_PLACEMENT_3D ( 'NONE', #21215, #12756, #1537 ) ;
#5178=DIRECTION ( 'NONE',  ( -0.000000000000000000, -0.000000000000000000, -1.000000000000000000 ) ) ;
#5179=VECTOR ( 'NONE', #24987, 1000.000000000000000 ) ;
#5182=CARTESIAN_POINT ( 'NONE',  ( 157.4999999999998579, 188.6515624061619576, -45.00000000000000000 ) ) ;
#5184=LINE ( 'NONE', #27289, #4793 ) ;
#5185=DIRECTION ( 'NONE',  ( 0.8916010070300285362, 0.4528218681369517995, 0.000000000000000000 ) ) ;
#5187=DIRECTION ( 'NONE',  ( -0.8916010070291696676, -0.4528218681386429467, 0.000000000000000000 ) ) ;
#5189=DIRECTION ( 'NONE',  ( 0.8916010070293783896, -0.4528218681382319422, 0.000000000000000000 ) ) ;
#5191=ORIENTED_EDGE ( 'NONE', *, *, #25877, .T. ) ;
#5192=DIRECTION ( 'NONE',  ( 1.000000000000000000, -0.000000000000000000, -0.000000000000000000 ) ) ;
#5193=VECTOR ( 'NONE', #6498, 1000.000000000000227 ) ;
#5196=VERTEX_POINT ( 'NONE', #11890 ) ;
#5198=VECTOR ( 'NONE', #18654, 1000.000000000000000 ) ;
#5202=DIRECTION ( 'NONE',  ( -0.000000000000000000, -0.000000000000000000, -1.000000000000000000 ) ) ;
#5204=VERTEX_POINT ( 'NONE', #7839 ) ;
#5208=ORIENTED_EDGE ( 'NONE', *, *, #22819, .F. ) ;
#5211=VECTOR ( 'NONE', #15544, 1000.000000000000000 ) ;
#5212=CARTESIAN_POINT ( 'NONE',  ( 158.0000000000017337, 42.94087446699998623, -45.00000000000000000 ) ) ;
#5215=DIRECTION ( 'NONE',  ( -0.000000000000000000, -0.000000000000000000, -1.000000000000000000 ) ) ;
#5216=DIRECTION ( 'NONE',  ( 0.8916010070293783896, -0.4528218681382319422, 0.000000000000000000 ) ) ;
#5219=DIRECTION ( 'NONE',  ( 0.4528218681375906218, -0.8916010070297041290, 0.000000000000000000 ) ) ;
#5220=DIRECTION ( 'NONE',  ( 0.8916010070296531698, -0.4528218681376911525, 0.000000000000000000 ) ) ;
#5221=DIRECTION ( 'NONE',  ( -0.8916010070298862056, 0.4528218681372321863, 0.000000000000000000 ) ) ;
#5226=CARTESIAN_POINT ( 'NONE',  ( 158.0000000000003979, 168.8424998498591663, 45.00000000000000000 ) ) ;
#5230=VERTEX_POINT ( 'NONE', #7982 ) ;
#5237=EDGE_CURVE ( 'NONE', #1480, #19459, #23351, .T. ) ;
#5244=ORIENTED_EDGE ( 'NONE', *, *, #24325, .T. ) ;
#5247=DIRECTION ( 'NONE',  ( -0.000000000000000000, 0.000000000000000000, -1.000000000000000000 ) ) ;
#5255=VECTOR ( 'NONE', #25733, 1000.000000000000114 ) ;
#5258=DIRECTION ( 'NONE',  ( -0.8916010070293384215, 0.4528218681383106015, 0.000000000000000000 ) ) ;
#5260=DIRECTION ( 'NONE',  ( 0.000000000000000000, -1.000000000000000000, 0.000000000000000000 ) ) ;
#5262=LINE ( 'NONE', #7706, #6028 ) ;
#5263=DIRECTION ( 'NONE',  ( 0.000000000000000000, 0.000000000000000000, -1.000000000000000000 ) ) ;
#5265=ORIENTED_EDGE ( 'NONE', *, *, #25795, .T. ) ;
#5267=ADVANCED_FACE ( 'NONE', ( #20770 ), #22933, .F. ) ;
#5269=CARTESIAN_POINT ( 'NONE',  ( 158.0000000000004547, 163.8267498348450886, 45.00000000000000000 ) ) ;
#5270=DIRECTION ( 'NONE',  ( -0.8916010070295314893, -0.4528218681379303501, 0.000000000000000000 ) ) ;
#5272=VERTEX_POINT ( 'NONE', #15168 ) ;
#5274=ORIENTED_EDGE ( 'NONE', *, *, #13093, .F. ) ;
#5280=VERTEX_POINT ( 'NONE', #17022 ) ;
#5281=VERTEX_POINT ( 'NONE', #17443 ) ;
#5293=VECTOR ( 'NONE', #16010, 1000.000000000000000 ) ;
#5298=VECTOR ( 'NONE', #19213, 1000.000000000000000 ) ;
#5301=CARTESIAN_POINT ( 'NONE',  ( 158.0000000000014211, 73.03537455708450921, 45.00000000000000000 ) ) ;
#5304=VECTOR ( 'NONE', #14957, 1000.000000000000227 ) ;
#5307=PLANE ( 'NONE',  #580 ) ;
#5308=VERTEX_POINT ( 'NONE', #6387 ) ;
#5312=EDGE_CURVE ( 'NONE', #5313, #13707, #23636, .T. ) ;
#5313=VERTEX_POINT ( 'NONE', #10990 ) ;
#5317=VECTOR ( 'NONE', #11866, 1000.000000000000000 ) ;
#5321=VECTOR ( 'NONE', #7664, 1000.000000000000000 ) ;
#5323=EDGE_CURVE ( 'NONE', #28009, #20034, #10422, .T. ) ;
#5324=ADVANCED_FACE ( 'NONE', ( #64 ), #17585, .F. ) ;
#5325=DIRECTION ( 'NONE',  ( 0.4528218681382713551, 0.8916010070293584056, -0.000000000000000000 ) ) ;
#5326=CARTESIAN_POINT ( 'NONE',  ( 158.0000000000001137, 195.9212499249295831, 45.00000000000000000 ) ) ;
#5329=CARTESIAN_POINT ( 'NONE',  ( 157.4999999999998579, 108.3995621659365867, 45.00000000000000000 ) ) ;
#5330=DIRECTION ( 'NONE',  ( 0.4528218681376512400, 0.8916010070296733758, -0.000000000000000000 ) ) ;
#5334=DIRECTION ( 'NONE',  ( 0.8916010070293584056, -0.4528218681382712996, 0.000000000000000000 ) ) ;
#5337=VERTEX_POINT ( 'NONE', #15021 ) ;
#5341=ORIENTED_EDGE ( 'NONE', *, *, #26487, .T. ) ;
#5344=CARTESIAN_POINT ( 'NONE',  ( 157.9999999999999432, 213.4763749774776045, 45.00000000000000000 ) ) ;
#5345=ORIENTED_EDGE ( 'NONE', *, *, #1095, .F. ) ;
#5347=LINE ( 'NONE', #9094, #6274 ) ;
#5348=CARTESIAN_POINT ( 'NONE',  ( 157.4999999999998579, 95.86018712840139244, -45.00000000000000000 ) ) ;
#5350=ORIENTED_EDGE ( 'NONE', *, *, #8213, .F. ) ;
#5351=CARTESIAN_POINT ( 'NONE',  ( 158.0000000000011653, 93.60624962464788723, 45.00000000000000000 ) ) ;
#5352=VERTEX_POINT ( 'NONE', #8269 ) ;
#5353=DIRECTION ( 'NONE',  ( -0.000000000000000000, 0.000000000000000000, -1.000000000000000000 ) ) ;
#5354=DIRECTION ( 'NONE',  ( 0.4528218681383106015, -0.8916010070293384215, 0.000000000000000000 ) ) ;
#5355=CARTESIAN_POINT ( 'NONE',  ( 157.4999999999996305, 283.9508126914284958, 45.00000000000000000 ) ) ;
#5359=EDGE_CURVE ( 'NONE', #1908, #1347, #6529, .T. ) ;
#5361=FACE_OUTER_BOUND ( 'NONE', #6248, .T. ) ;
#5362=EDGE_LOOP ( 'NONE', ( #1496, #23892, #16217, #10021 ) ) ;
#5363=CARTESIAN_POINT ( 'NONE',  ( 157.9999999999997442, 251.6023750975910218, 45.00000000000000000 ) ) ;
#5366=DIRECTION ( 'NONE',  ( -0.000000000000000000, -0.000000000000000000, -1.000000000000000000 ) ) ;
#5369=ORIENTED_EDGE ( 'NONE', *, *, #19830, .T. ) ;
#5372=CARTESIAN_POINT ( 'NONE',  ( 157.4999999999998579, 178.6200623761337738, -45.00000000000000000 ) ) ;
#5373=EDGE_LOOP ( 'NONE', ( #15599, #3528, #9688, #28153 ) ) ;
#5378=VECTOR ( 'NONE', #15647, 1000.000000000000000 ) ;
#5381=VERTEX_POINT ( 'NONE', #17301 ) ;
#5383=DIRECTION ( 'NONE',  ( 0.4528218681369924892, 0.8916010070300079970, -0.000000000000000000 ) ) ;
#5385=ORIENTED_EDGE ( 'NONE', *, *, #17804, .T. ) ;
#5386=ORIENTED_EDGE ( 'NONE', *, *, #1410, .T. ) ;
#5388=FACE_OUTER_BOUND ( 'NONE', #12590, .T. ) ;
#5389=EDGE_CURVE ( 'NONE', #23544, #10546, #19604, .T. ) ;
#5390=DIRECTION ( 'NONE',  ( 0.8916010070296632728, 0.4528218681376712240, 0.000000000000000000 ) ) ;
#5392=ADVANCED_FACE ( 'NONE', ( #4368 ), #13157, .F. ) ;
#5396=FACE_OUTER_BOUND ( 'NONE', #16065, .T. ) ;
#5404=LINE ( 'NONE', #12032, #5036 ) ;
#5405=CARTESIAN_POINT ( 'NONE',  ( 158.0000000000005684, 151.2873747973098659, 45.00000000000000000 ) ) ;
#5406=CARTESIAN_POINT ( 'NONE',  ( 157.9999999999998579, 221.0000000000000284, -45.00000000000000000 ) ) ;
#5407=ORIENTED_EDGE ( 'NONE', *, *, #1761, .F. ) ;
#5409=DIRECTION ( 'NONE',  ( -0.8916010070298658885, 0.4528218681372721544, 0.000000000000000000 ) ) ;
#5411=LINE ( 'NONE', #828, #387 ) ;
#5413=ORIENTED_EDGE ( 'NONE', *, *, #10060, .T. ) ;
#5414=ORIENTED_EDGE ( 'NONE', *, *, #26964, .T. ) ;
#5415=EDGE_LOOP ( 'NONE', ( #7116, #5350, #116, #4064 ) ) ;
#5416=VERTEX_POINT ( 'NONE', #22473 ) ;
#5418=LINE ( 'NONE', #972, #28319 ) ;
#5420=ADVANCED_FACE ( 'NONE', ( #22184 ), #13724, .F. ) ;
#5423=CARTESIAN_POINT ( 'NONE',  ( 157.4999999999998579, 166.0806873385985796, 45.00000000000000000 ) ) ;
#5426=CARTESIAN_POINT ( 'NONE',  ( 157.4999999999998579, 148.5255622860493077, 45.00000000000000000 ) ) ;
#5441=VECTOR ( 'NONE', #9220, 1000.000000000000000 ) ;
#5442=DIRECTION ( 'NONE',  ( 0.8916010070296733758, -0.4528218681376511845, 0.000000000000000000 ) ) ;
#5443=ORIENTED_EDGE ( 'NONE', *, *, #14392, .F. ) ;
#5449=EDGE_CURVE ( 'NONE', #20505, #11364, #26922, .T. ) ;
#5450=ORIENTED_EDGE ( 'NONE', *, *, #25752, .F. ) ;
#5451=CARTESIAN_POINT ( 'NONE',  ( 157.4999999999997726, 248.8405625863305204, -45.00000000000000000 ) ) ;
#5452=LINE ( 'NONE', #14650, #23726 ) ;
#5454=ADVANCED_FACE ( 'NONE', ( #22622 ), #11280, .F. ) ;
#5455=LINE ( 'NONE', #12230, #6399 ) ;
#5457=LINE ( 'NONE', #12234, #3207 ) ;
#5460=CARTESIAN_POINT ( 'NONE',  ( 158.0000000000007390, 133.7322497447605656, -45.00000000000000000 ) ) ;
#5461=FACE_OUTER_BOUND ( 'NONE', #7877, .T. ) ;
#5466=DIRECTION ( 'NONE',  ( -0.000000000000000000, -0.000000000000000000, -1.000000000000000000 ) ) ;
#5467=FACE_OUTER_BOUND ( 'NONE', #16177, .T. ) ;
#5473=CARTESIAN_POINT ( 'NONE',  ( 158.0000000000000000, 206.4606249624626457, -45.00000000000000000 ) ) ;
#5474=ORIENTED_EDGE ( 'NONE', *, *, #7241, .F. ) ;
#5487=DIRECTION ( 'NONE',  ( -0.000000000000000000, -0.000000000000000000, -1.000000000000000000 ) ) ;
#5490=CARTESIAN_POINT ( 'NONE',  ( 157.4999999999998579, 171.0964373536126573, -45.00000000000000000 ) ) ;
#5492=CARTESIAN_POINT ( 'NONE',  ( 158.0000000000006537, 145.7637497747887210, 45.00000000000000000 ) ) ;
#5495=CARTESIAN_POINT ( 'NONE',  ( 158.0000000000015916, 55.48024950453520177, 45.00000000000000000 ) ) ;
#5496=DIRECTION ( 'NONE',  ( 0.8916010070293409751, 0.4528218681383056610, 0.000000000000000000 ) ) ;
#5502=ADVANCED_FACE ( 'NONE', ( #17728 ), #9258, .F. ) ;
#5503=VECTOR ( 'NONE', #24364, 1000.000000000000114 ) ;
#5505=DIRECTION ( 'NONE',  ( -0.000000000000000000, -0.000000000000000000, -1.000000000000000000 ) ) ;
#5510=ORIENTED_EDGE ( 'NONE', *, *, #10062, .T. ) ;
#5522=VERTEX_POINT ( 'NONE', #354 ) ;
#5523=EDGE_CURVE ( 'NONE', #19520, #17350, #11571, .T. ) ;
#5525=ADVANCED_FACE ( 'NONE', ( #18170 ), #7247, .F. ) ;
#5527=ORIENTED_EDGE ( 'NONE', *, *, #20503, .F. ) ;
#5535=CARTESIAN_POINT ( 'NONE',  ( 157.4999999999997158, 261.3799376238655441, -45.00000000000000000 ) ) ;
#5536=LINE ( 'NONE', #4962, #17455 ) ;
#5543=DIRECTION ( 'NONE',  ( 0.000000000000000000, -1.000000000000000000, 0.000000000000000000 ) ) ;
#5544=ORIENTED_EDGE ( 'NONE', *, *, #17499, .F. ) ;
#5556=VERTEX_POINT ( 'NONE', #18308 ) ;
#5558=ORIENTED_EDGE ( 'NONE', *, *, #13406, .F. ) ;
#5561=ORIENTED_EDGE ( 'NONE', *, *, #11675, .F. ) ;
#5565=LINE ( 'NONE', #20513, #10671 ) ;
#5566=VECTOR ( 'NONE', #26512, 1000.000000000000114 ) ;
#5569=VECTOR ( 'NONE', #7744, 1000.000000000000000 ) ;
#5572=PLANE ( 'NONE',  #23221 ) ;
#5575=DIRECTION ( 'NONE',  ( 1.000000000000000000, 0.000000000000000000, -0.000000000000000000 ) ) ;
#5576=DIRECTION ( 'NONE',  ( -0.000000000000000000, -0.000000000000000000, -1.000000000000000000 ) ) ;
#5581=CARTESIAN_POINT ( 'NONE',  ( 157.4999999999998295, 231.2854375337815327, 45.00000000000000000 ) ) ;
#5585=ORIENTED_EDGE ( 'NONE', *, *, #11957, .T. ) ;
#5590=EDGE_CURVE ( 'NONE', #24084, #16325, #27993, .T. ) ;
#5591=ORIENTED_EDGE ( 'NONE', *, *, #12296, .T. ) ;
#5592=EDGE_CURVE ( 'NONE', #14086, #6262, #1298, .T. ) ;
#5594=EDGE_CURVE ( 'NONE', #10330, #7481, #1434, .T. ) ;
#5595=ORIENTED_EDGE ( 'NONE', *, *, #20567, .T. ) ;
#5596=ORIENTED_EDGE ( 'NONE', *, *, #4895, .F. ) ;
#5597=FACE_OUTER_BOUND ( 'NONE', #28263, .T. ) ;
#5611=CARTESIAN_POINT ( 'NONE',  ( 158.0000000000013927, 73.54324956459154805, 45.00000000000000000 ) ) ;
#5615=ADVANCED_FACE ( 'NONE', ( #8048 ), #16817, .F. ) ;
#5619=ORIENTED_EDGE ( 'NONE', *, *, #20861, .T. ) ;
#5620=VECTOR ( 'NONE', #17254, 1000.000000000000000 ) ;
#5623=DIRECTION ( 'NONE',  ( -0.8916010070295820045, -0.4528218681378310406, 0.000000000000000000 ) ) ;
#5626=ORIENTED_EDGE ( 'NONE', *, *, #20964, .T. ) ;
#5629=CARTESIAN_POINT ( 'NONE',  ( 157.4999999999998579, 193.6673124211760353, -45.00000000000000000 ) ) ;
#5633=CARTESIAN_POINT ( 'NONE',  ( 157.9999999999996589, 273.6653751576470768, 45.00000000000000000 ) ) ;
#5634=ORIENTED_EDGE ( 'NONE', *, *, #799, .T. ) ;
#5637=VECTOR ( 'NONE', #5076, 1000.000000000000000 ) ;
#5638=DIRECTION ( 'NONE',  ( -0.000000000000000000, -0.000000000000000000, -1.000000000000000000 ) ) ;
#5639=DIRECTION ( 'NONE',  ( 0.4528218681374907573, -0.8916010070297548662, 0.000000000000000000 ) ) ;
#5642=CARTESIAN_POINT ( 'NONE',  ( 158.0000000000003979, 168.8424998498591663, 45.00000000000000000 ) ) ;
#5644=CARTESIAN_POINT ( 'NONE',  ( 157.4999999999998579, 173.6043123611196961, 45.00000000000000000 ) ) ;
#5650=CARTESIAN_POINT ( 'NONE',  ( 157.4999999999998579, 125.9546872184859012, 45.00000000000000000 ) ) ;
#5652=CARTESIAN_POINT ( 'NONE',  ( 158.0000000000010232, 106.1456246621830957, 45.00000000000000000 ) ) ;
#5655=VERTEX_POINT ( 'NONE', #5226 ) ;
#5657=LINE ( 'NONE', #23184, #26746 ) ;
#5660=VERTEX_POINT ( 'NONE', #23562 ) ;
#5664=DIRECTION ( 'NONE',  ( -0.000000000000000000, -0.000000000000000000, -1.000000000000000000 ) ) ;
#5666=ORIENTED_EDGE ( 'NONE', *, *, #25685, .F. ) ;
#5667=VECTOR ( 'NONE', #9069, 1000.000000000000000 ) ;
#5674=ORIENTED_EDGE ( 'NONE', *, *, #19028, .T. ) ;
#5675=VERTEX_POINT ( 'NONE', #19390 ) ;
#5676=VECTOR ( 'NONE', #18447, 1000.000000000000114 ) ;
#5682=DIRECTION ( 'NONE',  ( -0.000000000000000000, -0.000000000000000000, -1.000000000000000000 ) ) ;
#5685=DIRECTION ( 'NONE',  ( -0.000000000000000000, -0.000000000000000000, -1.000000000000000000 ) ) ;
#5686=CARTESIAN_POINT ( 'NONE',  ( 158.0000000000006253, 148.2716247822957882, 45.00000000000000000 ) ) ;
#5688=DIRECTION ( 'NONE',  ( -0.000000000000000000, 0.000000000000000000, -1.000000000000000000 ) ) ;
#5691=CARTESIAN_POINT ( 'NONE',  ( 158.0000000000010800, 101.1298746471690038, 45.00000000000000000 ) ) ;
#5694=ADVANCED_FACE ( 'NONE', ( #2422 ), #15090, .F. ) ;
#5697=VECTOR ( 'NONE', #16439, 1000.000000000000000 ) ;
#5701=PLANE ( 'NONE',  #10338 ) ;
#5706=ORIENTED_EDGE ( 'NONE', *, *, #14017, .F. ) ;
#5708=VECTOR ( 'NONE', #22141, 1000.000000000000000 ) ;
#5715=LINE ( 'NONE', #18931, #9461 ) ;
#5716=LINE ( 'NONE', #1685, #5298 ) ;
#5719=ORIENTED_EDGE ( 'NONE', *, *, #25282, .T. ) ;
#5721=DIRECTION ( 'NONE',  ( -0.000000000000000000, -0.000000000000000000, -1.000000000000000000 ) ) ;
#5724=VERTEX_POINT ( 'NONE', #8478 ) ;
#5725=AXIS2_PLACEMENT_3D ( 'NONE', #22575, #20269, #27015 ) ;
#5729=VECTOR ( 'NONE', #23323, 1000.000000000000000 ) ;
#5730=ORIENTED_EDGE ( 'NONE', *, *, #25693, .F. ) ;
#5734=LINE ( 'NONE', #9779, #15956 ) ;
#5739=DIRECTION ( 'NONE',  ( -0.000000000000000000, -0.000000000000000000, -1.000000000000000000 ) ) ;
#5741=CARTESIAN_POINT ( 'NONE',  ( 157.9999999999998579, 219.0000000000000284, 45.00000000000000000 ) ) ;
#5749=DIRECTION ( 'NONE',  ( 0.8916010070295820045, -0.4528218681378310406, 0.000000000000000000 ) ) ;
#5753=CARTESIAN_POINT ( 'NONE',  ( 157.9999999999998579, 221.5078750075070104, 45.00000000000000000 ) ) ;
#5754=EDGE_LOOP ( 'NONE', ( #17741, #15602, #4280, #18138 ) ) ;
#5757=ORIENTED_EDGE ( 'NONE', *, *, #26622, .T. ) ;
#5765=ORIENTED_EDGE ( 'NONE', *, *, #25375, .T. ) ;
#5766=VECTOR ( 'NONE', #9184, 1000.000000000000000 ) ;
#5768=CARTESIAN_POINT ( 'NONE',  ( 158.0000000000015916, 53.48024950453520177, -45.00000000000000000 ) ) ;
#5776=EDGE_CURVE ( 'NONE', #10648, #13244, #6885, .T. ) ;
#5778=FACE_OUTER_BOUND ( 'NONE', #7198, .T. ) ;
#5779=FACE_OUTER_BOUND ( 'NONE', #4908, .T. ) ;
#5780=DIRECTION ( 'NONE',  ( -0.8916010070293584056, 0.4528218681382713551, 0.000000000000000000 ) ) ;
#5781=VECTOR ( 'NONE', #25160, 1000.000000000000000 ) ;
#5782=CARTESIAN_POINT ( 'NONE',  ( 158.0000000000014211, 71.03537455708449500, 45.00000000000000000 ) ) ;
#5785=CARTESIAN_POINT ( 'NONE',  ( 167.4999999999996589, 258.6181251126050711, 1.387778780781445676E-14 ) ) ;
#5787=VECTOR ( 'NONE', #18894, 999.9999999999998863 ) ;
#5789=FACE_OUTER_BOUND ( 'NONE', #19993, .T. ) ;
#5790=LINE ( 'NONE', #17269, #12127 ) ;
#5792=LINE ( 'NONE', #25331, #18314 ) ;
#5796=LINE ( 'NONE', #1204, #20196 ) ;
#5797=CARTESIAN_POINT ( 'NONE',  ( 158.0000000000004832, 161.3188748273380213, 45.00000000000000000 ) ) ;
#5801=ORIENTED_EDGE ( 'NONE', *, *, #5312, .F. ) ;
#5802=LINE ( 'NONE', #8529, #7886 ) ;
#5804=ORIENTED_EDGE ( 'NONE', *, *, #9709, .F. ) ;
#5807=CARTESIAN_POINT ( 'NONE',  ( 157.9999999999997158, 263.6338751276190351, 45.00000000000000000 ) ) ;
#5809=ORIENTED_EDGE ( 'NONE', *, *, #7517, .F. ) ;
#5812=EDGE_CURVE ( 'NONE', #5660, #12148, #22832, .T. ) ;
#5816=LINE ( 'NONE', #1509, #12206 ) ;
#5822=VECTOR ( 'NONE', #12681, 1000.000000000000114 ) ;
#5825=VECTOR ( 'NONE', #10163, 1000.000000000000000 ) ;
#5826=EDGE_CURVE ( 'NONE', #5308, #1670, #7179, .T. ) ;
#5827=EDGE_CURVE ( 'NONE', #23450, #16902, #15950, .T. ) ;
#5828=DIRECTION ( 'NONE',  ( -0.000000000000000000, -0.000000000000000000, -1.000000000000000000 ) ) ;
#5835=VERTEX_POINT ( 'NONE', #16236 ) ;
#5836=DIRECTION ( 'NONE',  ( 0.4528218681371322663, 0.8916010070299369428, -0.000000000000000000 ) ) ;
#5837=ORIENTED_EDGE ( 'NONE', *, *, #18247, .F. ) ;
#5840=CARTESIAN_POINT ( 'NONE',  ( 157.4999999999998295, 218.7460624962465090, 45.00000000000000000 ) ) ;
#5841=EDGE_CURVE ( 'NONE', #6158, #27297, #14219, .T. ) ;
#5851=CARTESIAN_POINT ( 'NONE',  ( 158.0000000000015064, 61.00387452705632541, 45.00000000000000000 ) ) ;
#5856=CARTESIAN_POINT ( 'NONE',  ( 158.0000000000013642, 76.05112457209858690, 45.00000000000000000 ) ) ;
#5858=EDGE_CURVE ( 'NONE', #969, #16733, #22694, .T. ) ;
#5860=CARTESIAN_POINT ( 'NONE',  ( 158.0000000000001705, 188.9054999099155054, 45.00000000000000000 ) ) ;
#5869=ORIENTED_EDGE ( 'NONE', *, *, #17328, .F. ) ;
#5877=CARTESIAN_POINT ( 'NONE',  ( 157.9999999999999432, 211.4763749774776045, 45.00000000000000000 ) ) ;
#5884=VECTOR ( 'NONE', #11352, 999.9999999999998863 ) ;
#5892=AXIS2_PLACEMENT_3D ( 'NONE', #4404, #21800, #12908 ) ;
#5899=ORIENTED_EDGE ( 'NONE', *, *, #2367, .T. ) ;
#5900=CARTESIAN_POINT ( 'NONE',  ( 157.4999999999998579, 85.82868709837320864, 45.00000000000000000 ) ) ;
#5901=CARTESIAN_POINT ( 'NONE',  ( 157.4999999999998579, 43.19481197075347723, 45.00000000000000000 ) ) ;
#5903=ORIENTED_EDGE ( 'NONE', *, *, #2015, .T. ) ;
#5904=LINE ( 'NONE', #5768, #793 ) ;
#5908=EDGE_CURVE ( 'NONE', #22677, #21766, #10320, .T. ) ;
#5912=ORIENTED_EDGE ( 'NONE', *, *, #22345, .F. ) ;
#5924=FACE_OUTER_BOUND ( 'NONE', #26826, .T. ) ;
#5926=CARTESIAN_POINT ( 'NONE',  ( 157.9999999999997442, 253.6023750975910502, 45.00000000000000000 ) ) ;
#5927=CARTESIAN_POINT ( 'NONE',  ( 158.0000000000002558, 183.3818748873943889, 45.00000000000000000 ) ) ;
#5931=AXIS2_PLACEMENT_3D ( 'NONE', #7184, #11509, #13807 ) ;
#5933=CARTESIAN_POINT ( 'NONE',  ( 157.9999999999996874, 268.6496251426330559, 45.00000000000000000 ) ) ;
#5935=ORIENTED_EDGE ( 'NONE', *, *, #22521, .T. ) ;
#5939=EDGE_LOOP ( 'NONE', ( #26486, #25208, #27890, #11593 ) ) ;
#5941=DIRECTION ( 'NONE',  ( -0.8916010070294200229, -0.4528218681381501742, 0.000000000000000000 ) ) ;
#5943=ORIENTED_EDGE ( 'NONE', *, *, #24148, .F. ) ;
#5944=VECTOR ( 'NONE', #11048, 1000.000000000000114 ) ;
#5950=ORIENTED_EDGE ( 'NONE', *, *, #27441, .T. ) ;
#5951=DIRECTION ( 'NONE',  ( -0.8916010070293283185, -0.4528218681383305855, 0.000000000000000000 ) ) ;
#5952=VECTOR ( 'NONE', #7418, 1000.000000000000000 ) ;
#5955=CARTESIAN_POINT ( 'NONE',  ( 157.4999999999997726, 243.8248125713165280, -45.00000000000000000 ) ) ;
#5956=DIRECTION ( 'NONE',  ( 0.8916010070297948342, -0.4528218681374120425, 0.000000000000000000 ) ) ;
#5963=DIRECTION ( 'NONE',  ( 0.000000000000000000, -1.000000000000000000, 0.000000000000000000 ) ) ;
#5966=ORIENTED_EDGE ( 'NONE', *, *, #24671, .T. ) ;
#5968=CARTESIAN_POINT ( 'NONE',  ( 158.0000000000015916, 53.48024950453520177, 45.00000000000000000 ) ) ;
#5975=ORIENTED_EDGE ( 'NONE', *, *, #3251, .T. ) ;
#5976=LINE ( 'NONE', #19052, #2538 ) ;
#5995=FACE_OUTER_BOUND ( 'NONE', #2579, .T. ) ;
#5996=FACE_OUTER_BOUND ( 'NONE', #12465, .T. ) ;
#5997=DIRECTION ( 'NONE',  ( 0.4528218681382713551, 0.8916010070293584056, -0.000000000000000000 ) ) ;
#5998=FACE_OUTER_BOUND ( 'NONE', #2146, .T. ) ;
#6017=LINE ( 'NONE', #24122, #10444 ) ;
#6018=VECTOR ( 'NONE', #11651, 1000.000000000000000 ) ;
#6019=EDGE_CURVE ( 'NONE', #9427, #8629, #27824, .T. ) ;
#6020=EDGE_CURVE ( 'NONE', #21781, #1313, #12632, .T. ) ;
#6025=PLANE ( 'NONE',  #8674 ) ;
#6027=EDGE_CURVE ( 'NONE', #883, #21211, #1129, .T. ) ;
#6028=VECTOR ( 'NONE', #9860, 1000.000000000000000 ) ;
#6031=DIRECTION ( 'NONE',  ( 0.000000000000000000, -1.000000000000000000, 0.000000000000000000 ) ) ;
#6033=VECTOR ( 'NONE', #26754, 1000.000000000000114 ) ;
#6035=VECTOR ( 'NONE', #28350, 1000.000000000000000 ) ;
#6045=CARTESIAN_POINT ( 'NONE',  ( 157.9999999999997158, 259.1260001201120531, 45.00000000000000000 ) ) ;
#6046=DIRECTION ( 'NONE',  ( 0.4528218681376305343, -0.8916010070296839229, 0.000000000000000000 ) ) ;
#6049=DIRECTION ( 'NONE',  ( -0.8916010070293383105, -0.4528218681383106015, 0.000000000000000000 ) ) ;
#6053=EDGE_LOOP ( 'NONE', ( #14402, #26758, #191, #10471 ) ) ;
#6055=ORIENTED_EDGE ( 'NONE', *, *, #28335, .F. ) ;
#6061=DIRECTION ( 'NONE',  ( 0.8916010070299267287, -0.4528218681371523058, 0.000000000000000000 ) ) ;
#6063=ORIENTED_EDGE ( 'NONE', *, *, #17923, .T. ) ;
#6064=CARTESIAN_POINT ( 'NONE',  ( 158.0000000000003126, 178.3661248723802828, -45.00000000000000000 ) ) ;
#6067=CARTESIAN_POINT ( 'NONE',  ( 158.0000000000013642, 78.05112457209858690, -45.00000000000000000 ) ) ;
#6068=ADVANCED_FACE ( 'NONE', ( #9902 ), #1555, .F. ) ;
#6071=VECTOR ( 'NONE', #4112, 1000.000000000000000 ) ;
#6074=VECTOR ( 'NONE', #9515, 1000.000000000000000 ) ;
#6080=VECTOR ( 'NONE', #18111, 1000.000000000000000 ) ;
#6082=VECTOR ( 'NONE', #296, 1000.000000000000000 ) ;
#6083=DIRECTION ( 'NONE',  ( -0.8916010070293283185, -0.4528218681383305855, 0.000000000000000000 ) ) ;
#6089=EDGE_LOOP ( 'NONE', ( #25056, #20679, #14609, #14583 ) ) ;
#6090=EDGE_LOOP ( 'NONE', ( #9132, #21389, #28360, #12567 ) ) ;
#6094=LINE ( 'NONE', #19166, #10794 ) ;
#6095=CARTESIAN_POINT ( 'NONE',  ( 157.9999999999998010, 236.0472500450420341, 45.00000000000000000 ) ) ;
#6097=AXIS2_PLACEMENT_3D ( 'NONE', #9717, #18343, #27091 ) ;
#6098=AXIS2_PLACEMENT_3D ( 'NONE', #24675, #13199, #2539 ) ;
#6099=CARTESIAN_POINT ( 'NONE',  ( 158.0000000000000853, 200.9369999399436892, 45.00000000000000000 ) ) ;
#6103=CARTESIAN_POINT ( 'NONE',  ( 158.0000000000003126, 178.3661248723802828, 45.00000000000000000 ) ) ;
#6109=EDGE_CURVE ( 'NONE', #20915, #1874, #21804, .T. ) ;
#6111=EDGE_CURVE ( 'NONE', #22406, #23236, #2113, .T. ) ;
#6119=VECTOR ( 'NONE', #23840, 1000.000000000000114 ) ;
#6122=ORIENTED_EDGE ( 'NONE', *, *, #13524, .T. ) ;
#6123=LINE ( 'NONE', #7853, #20923 ) ;
#6126=VERTEX_POINT ( 'NONE', #10604 ) ;
#6129=VERTEX_POINT ( 'NONE', #2388 ) ;
#6130=DIRECTION ( 'NONE',  ( 0.4528218681377911836, -0.8916010070296023216, 0.000000000000000000 ) ) ;
#6138=CARTESIAN_POINT ( 'NONE',  ( 157.4999999999998579, 60.74993702330277756, -45.00000000000000000 ) ) ;
#6144=VECTOR ( 'NONE', #8410, 1000.000000000000114 ) ;
#6147=CARTESIAN_POINT ( 'NONE',  ( 157.4999999999998579, 115.9231871884577174, 45.00000000000000000 ) ) ;
#6148=ORIENTED_EDGE ( 'NONE', *, *, #17431, .F. ) ;
#6150=CARTESIAN_POINT ( 'NONE',  ( 157.9999999999999147, 215.9842499849850697, 45.00000000000000000 ) ) ;
#6152=DIRECTION ( 'NONE',  ( 0.8916010070298658885, -0.4528218681372722099, 0.000000000000000000 ) ) ;
#6154=ORIENTED_EDGE ( 'NONE', *, *, #23496, .T. ) ;
#6158=VERTEX_POINT ( 'NONE', #15352 ) ;
#6162=AXIS2_PLACEMENT_3D ( 'NONE', #27296, #3847, #9516 ) ;
#6163=ORIENTED_EDGE ( 'NONE', *, *, #25003, .T. ) ;
#6164=ORIENTED_EDGE ( 'NONE', *, *, #10246, .F. ) ;
#6170=DIRECTION ( 'NONE',  ( 0.000000000000000000, -1.000000000000000000, 0.000000000000000000 ) ) ;
#6171=CARTESIAN_POINT ( 'NONE',  ( 158.0000000000001137, 193.9212499249295831, 45.00000000000000000 ) ) ;
#6176=CARTESIAN_POINT ( 'NONE',  ( 158.0000000000005400, 156.3031248123239436, -45.00000000000000000 ) ) ;
#6179=ORIENTED_EDGE ( 'NONE', *, *, #885, .T. ) ;
#6181=EDGE_CURVE ( 'NONE', #21202, #23711, #4126, .T. ) ;
#6182=ADVANCED_FACE ( 'NONE', ( #21941 ), #3982, .F. ) ;
#6186=VERTEX_POINT ( 'NONE', #23677 ) ;
#6195=EDGE_CURVE ( 'NONE', #24666, #16446, #6708, .T. ) ;
#6197=LINE ( 'NONE', #4032, #19219 ) ;
#6200=ORIENTED_EDGE ( 'NONE', *, *, #2124, .F. ) ;
#6203=CARTESIAN_POINT ( 'NONE',  ( 158.0000000000010800, 103.1298746471690038, -45.00000000000000000 ) ) ;
#6205=ORIENTED_EDGE ( 'NONE', *, *, #17321, .T. ) ;
#6209=DIRECTION ( 'NONE',  ( 0.8916010070294605461, 0.4528218681380702382, 0.000000000000000000 ) ) ;
#6210=LINE ( 'NONE', #19005, #8915 ) ;
#6211=ORIENTED_EDGE ( 'NONE', *, *, #10135, .T. ) ;
#6214=ADVANCED_FACE ( 'NONE', ( #6283 ), #22664, .F. ) ;
#6215=CARTESIAN_POINT ( 'NONE',  ( 157.4999999999998579, 198.6830624361901414, 45.00000000000000000 ) ) ;
#6217=DIRECTION ( 'NONE',  ( -0.000000000000000000, -0.000000000000000000, -1.000000000000000000 ) ) ;
#6218=ORIENTED_EDGE ( 'NONE', *, *, #23204, .F. ) ;
#6219=DIRECTION ( 'NONE',  ( 1.000000000000000000, 0.000000000000000000, -0.000000000000000000 ) ) ;
#6220=AXIS2_PLACEMENT_3D ( 'NONE', #27300, #7912, #22865 ) ;
#6221=ORIENTED_EDGE ( 'NONE', *, *, #24606, .T. ) ;
#6222=DIRECTION ( 'NONE',  ( 0.8916010070293584056, -0.4528218681382712996, 0.000000000000000000 ) ) ;
#6224=ORIENTED_EDGE ( 'NONE', *, *, #23270, .F. ) ;
#6226=DIRECTION ( 'NONE',  ( 0.4528218681383106015, 0.8916010070293384215, -0.000000000000000000 ) ) ;
#6230=VERTEX_POINT ( 'NONE', #9158 ) ;
#6232=ADVANCED_FACE ( 'NONE', ( #4832 ), #24669, .F. ) ;
#6233=DIRECTION ( 'NONE',  ( 0.000000000000000000, -1.000000000000000000, 0.000000000000000000 ) ) ;
#6234=ADVANCED_FACE ( 'NONE', ( #7142 ), #22370, .F. ) ;
#6235=LINE ( 'NONE', #26192, #7144 ) ;
#6245=DIRECTION ( 'NONE',  ( -0.000000000000000000, -0.000000000000000000, -1.000000000000000000 ) ) ;
#6247=DIRECTION ( 'NONE',  ( 0.000000000000000000, -1.000000000000000000, 0.000000000000000000 ) ) ;
#6248=EDGE_LOOP ( 'NONE', ( #15713, #24751, #6320, #2348 ) ) ;
#6250=CARTESIAN_POINT ( 'NONE',  ( 157.4999999999998579, 156.0491873085704242, 45.00000000000000000 ) ) ;
#6251=LINE ( 'NONE', #6536, #8241 ) ;
#6253=LINE ( 'NONE', #8981, #21626 ) ;
#6254=LINE ( 'NONE', #27652, #18901 ) ;
#6256=AXIS2_PLACEMENT_3D ( 'NONE', #17110, #26150, #4024 ) ;
#6257=CARTESIAN_POINT ( 'NONE',  ( 157.9999999999997726, 243.5708750675630370, -45.00000000000000000 ) ) ;
#6258=ORIENTED_EDGE ( 'NONE', *, *, #28312, .T. ) ;
#6259=CARTESIAN_POINT ( 'NONE',  ( 157.9999999999998010, 239.0630000600560550, 45.00000000000000000 ) ) ;
#6261=AXIS2_PLACEMENT_3D ( 'NONE', #4226, #23916, #26621 ) ;
#6262=VERTEX_POINT ( 'NONE', #7291 ) ;
#6264=EDGE_LOOP ( 'NONE', ( #13399, #26499, #9027, #5719 ) ) ;
#6269=CARTESIAN_POINT ( 'NONE',  ( 157.4999999999998579, 196.1751874286831026, -45.00000000000000000 ) ) ;
#6274=VECTOR ( 'NONE', #13995, 1000.000000000000000 ) ;
#6275=LINE ( 'NONE', #16777, #11030 ) ;
#6279=DIRECTION ( 'NONE',  ( -0.000000000000000000, -0.000000000000000000, -1.000000000000000000 ) ) ;
#6282=ORIENTED_EDGE ( 'NONE', *, *, #28042, .F. ) ;
#6283=FACE_OUTER_BOUND ( 'NONE', #2505, .T. ) ;
#6284=DIRECTION ( 'NONE',  ( -0.000000000000000000, 0.000000000000000000, -1.000000000000000000 ) ) ;
#6285=FACE_OUTER_BOUND ( 'NONE', #8277, .T. ) ;
#6286=EDGE_LOOP ( 'NONE', ( #15963, #23267, #26064, #3538 ) ) ;
#6291=ORIENTED_EDGE ( 'NONE', *, *, #19938, .T. ) ;
#6295=ORIENTED_EDGE ( 'NONE', *, *, #7225, .F. ) ;
#6298=LINE ( 'NONE', #8323, #17324 ) ;
#6299=ADVANCED_FACE ( 'NONE', ( #16203 ), #11469, .F. ) ;
#6300=EDGE_CURVE ( 'NONE', #10546, #21766, #15634, .T. ) ;
#6302=DIRECTION ( 'NONE',  ( 0.000000000000000000, -1.000000000000000000, 0.000000000000000000 ) ) ;
#6307=DIRECTION ( 'NONE',  ( -0.000000000000000000, -0.000000000000000000, -1.000000000000000000 ) ) ;
#6312=LINE ( 'NONE', #1581, #21602 ) ;
#6313=FACE_OUTER_BOUND ( 'NONE', #15755, .T. ) ;
#6314=ORIENTED_EDGE ( 'NONE', *, *, #10081, .F. ) ;
#6317=VERTEX_POINT ( 'NONE', #540 ) ;
#6319=EDGE_CURVE ( 'NONE', #12718, #1480, #15781, .T. ) ;
#6320=ORIENTED_EDGE ( 'NONE', *, *, #23299, .F. ) ;
#6324=CARTESIAN_POINT ( 'NONE',  ( 157.9999999999999716, 210.9684999699701393, 45.00000000000000000 ) ) ;
#6326=VECTOR ( 'NONE', #2309, 1000.000000000000227 ) ;
#6327=ORIENTED_EDGE ( 'NONE', *, *, #1410, .F. ) ;
#6332=CARTESIAN_POINT ( 'NONE',  ( 158.0000000000003979, 168.8424998498591663, -45.00000000000000000 ) ) ;
#6333=ORIENTED_EDGE ( 'NONE', *, *, #4959, .F. ) ;
#6335=VERTEX_POINT ( 'NONE', #24525 ) ;
#6340=FACE_OUTER_BOUND ( 'NONE', #10827, .T. ) ;
#6341=CARTESIAN_POINT ( 'NONE',  ( 157.4999999999998579, 193.6673124211760353, -45.00000000000000000 ) ) ;
#6344=CARTESIAN_POINT ( 'NONE',  ( 157.9999999999998010, 236.5551250525490161, 45.00000000000000000 ) ) ;
#6345=VECTOR ( 'NONE', #27258, 1000.000000000000227 ) ;
#6351=CARTESIAN_POINT ( 'NONE',  ( 157.9999999999997442, 254.1102501050980322, -45.00000000000000000 ) ) ;
#6355=ORIENTED_EDGE ( 'NONE', *, *, #26523, .T. ) ;
#6356=CARTESIAN_POINT ( 'NONE',  ( 158.0000000000006821, 140.7479997597746433, 45.00000000000000000 ) ) ;
#6360=VECTOR ( 'NONE', #11203, 1000.000000000000000 ) ;
#6368=CARTESIAN_POINT ( 'NONE',  ( 158.0000000000007958, 128.7164997297464595, 45.00000000000000000 ) ) ;
#6372=CARTESIAN_POINT ( 'NONE',  ( 157.9999999999998295, 224.0157500150140208, 45.00000000000000000 ) ) ;
#6374=ADVANCED_FACE ( 'NONE', ( #14744 ), #23499, .F. ) ;
#6377=DIRECTION ( 'NONE',  ( 0.000000000000000000, 0.000000000000000000, 1.000000000000000000 ) ) ;
#6379=CARTESIAN_POINT ( 'NONE',  ( 158.0000000000005116, 158.8109998198309825, 45.00000000000000000 ) ) ;
#6384=CARTESIAN_POINT ( 'NONE',  ( 158.0000000000005116, 158.8109998198309825, 45.00000000000000000 ) ) ;
#6386=DIRECTION ( 'NONE',  ( 0.000000000000000000, -1.000000000000000000, 0.000000000000000000 ) ) ;
#6387=CARTESIAN_POINT ( 'NONE',  ( 158.0000000000012221, 88.59049960963380954, 45.00000000000000000 ) ) ;
#6391=CARTESIAN_POINT ( 'NONE',  ( 157.9999999999996305, 284.2047501951820436, 45.00000000000000000 ) ) ;
#6394=FACE_OUTER_BOUND ( 'NONE', #1301, .T. ) ;
#6396=CARTESIAN_POINT ( 'NONE',  ( 157.9999999999996305, 286.2047501951820436, -45.00000000000000000 ) ) ;
#6398=ORIENTED_EDGE ( 'NONE', *, *, #3991, .F. ) ;
#6399=VECTOR ( 'NONE', #7762, 1000.000000000000227 ) ;
#6400=ADVANCED_FACE ( 'NONE', ( #10429 ), #27792, .F. ) ;
#6402=ORIENTED_EDGE ( 'NONE', *, *, #18143, .T. ) ;
#6404=VERTEX_POINT ( 'NONE', #23079 ) ;
#6409=ORIENTED_EDGE ( 'NONE', *, *, #22288, .F. ) ;
#6415=AXIS2_PLACEMENT_3D ( 'NONE', #17916, #26667, #13768 ) ;
#6420=CARTESIAN_POINT ( 'NONE',  ( 158.0000000000015632, 55.98812451204224061, 45.00000000000000000 ) ) ;
#6422=CARTESIAN_POINT ( 'NONE',  ( 158.0000000000012221, 90.59049960963380954, 45.00000000000000000 ) ) ;
#6424=CARTESIAN_POINT ( 'NONE',  ( 158.0000000000009379, 116.1771246922112653, 45.00000000000000000 ) ) ;
#6426=CARTESIAN_POINT ( 'NONE',  ( 157.4999999999998579, 123.4468122109788482, 45.00000000000000000 ) ) ;
#6427=EDGE_LOOP ( 'NONE', ( #13964, #19714, #18868, #25130 ) ) ;
#6428=FACE_OUTER_BOUND ( 'NONE', #15933, .T. ) ;
#6429=AXIS2_PLACEMENT_3D ( 'NONE', #24801, #2809, #5390 ) ;
#6431=CARTESIAN_POINT ( 'NONE',  ( 158.0000000000008242, 126.2086247222394206, -45.00000000000000000 ) ) ;
#6434=EDGE_CURVE ( 'NONE', #26356, #6230, #25092, .T. ) ;
#6435=EDGE_CURVE ( 'NONE', #8321, #22143, #5404, .T. ) ;
#6438=VERTEX_POINT ( 'NONE', #3667 ) ;
#6439=CARTESIAN_POINT ( 'NONE',  ( 157.4999999999996305, 288.9665627064425735, 45.00000000000000000 ) ) ;
#6444=EDGE_LOOP ( 'NONE', ( #2742, #21071, #25603, #21574 ) ) ;
#6445=CARTESIAN_POINT ( 'NONE',  ( 158.0000000000003126, 176.3661248723802828, -45.00000000000000000 ) ) ;
#6449=VECTOR ( 'NONE', #13078, 1000.000000000000000 ) ;
#6450=CARTESIAN_POINT ( 'NONE',  ( 158.0000000000003695, 171.3503748573662051, 45.00000000000000000 ) ) ;
#6453=FACE_OUTER_BOUND ( 'NONE', #23510, .T. ) ;
#6454=LINE ( 'NONE', #19671, #1134 ) ;
#6460=ADVANCED_FACE ( 'NONE', ( #6394 ), #15173, .F. ) ;
#6461=PLANE ( 'NONE',  #14824 ) ;
#6462=ORIENTED_EDGE ( 'NONE', *, *, #25990, .T. ) ;
#6468=LINE ( 'NONE', #13372, #13114 ) ;
#6469=VERTEX_POINT ( 'NONE', #22046 ) ;
#6473=VECTOR ( 'NONE', #23994, 1000.000000000000000 ) ;
#6474=CARTESIAN_POINT ( 'NONE',  ( 157.9999999999997442, 254.1102501050980322, 45.00000000000000000 ) ) ;
#6476=ORIENTED_EDGE ( 'NONE', *, *, #15072, .T. ) ;
#6487=CARTESIAN_POINT ( 'NONE',  ( 158.0000000000014495, 66.01962454207041731, -45.00000000000000000 ) ) ;
#6489=EDGE_CURVE ( 'NONE', #8537, #1982, #6251, .T. ) ;
#6490=ORIENTED_EDGE ( 'NONE', *, *, #3085, .T. ) ;
#6493=DIRECTION ( 'NONE',  ( -0.000000000000000000, -0.000000000000000000, -1.000000000000000000 ) ) ;
#6498=DIRECTION ( 'NONE',  ( 0.8916010070300078860, -0.4528218681369923782, 0.000000000000000000 ) ) ;
#6500=ORIENTED_EDGE ( 'NONE', *, *, #19957, .T. ) ;
#6503=AXIS2_PLACEMENT_3D ( 'NONE', #19883, #15734, #20168 ) ;
#6506=ORIENTED_EDGE ( 'NONE', *, *, #3861, .F. ) ;
#6508=CARTESIAN_POINT ( 'NONE',  ( 158.0000000000002842, 180.8739998798873501, 45.00000000000000000 ) ) ;
#6511=VECTOR ( 'NONE', #21773, 1000.000000000000000 ) ;
#6513=VERTEX_POINT ( 'NONE', #26209 ) ;
#6518=DIRECTION ( 'NONE',  ( 0.000000000000000000, -1.000000000000000000, 0.000000000000000000 ) ) ;
#6521=LINE ( 'NONE', #19878, #5068 ) ;
#6526=LINE ( 'NONE', #21762, #21394 ) ;
#6527=CARTESIAN_POINT ( 'NONE',  ( 157.4999999999998579, 130.9704372334999789, -45.00000000000000000 ) ) ;
#6529=LINE ( 'NONE', #8690, #1769 ) ;
#6531=CARTESIAN_POINT ( 'NONE',  ( 157.4999999999998579, 193.6673124211760353, 45.00000000000000000 ) ) ;
#6532=EDGE_LOOP ( 'NONE', ( #14267, #27352, #15892, #7949 ) ) ;
#6536=CARTESIAN_POINT ( 'NONE',  ( 158.0000000000005116, 158.8109998198309825, 45.00000000000000000 ) ) ;
#6537=CARTESIAN_POINT ( 'NONE',  ( 158.0000000000001421, 191.4133749174225443, 45.00000000000000000 ) ) ;
#6538=CARTESIAN_POINT ( 'NONE',  ( 158.0000000000001137, 193.9212499249295831, 45.00000000000000000 ) ) ;
#6545=CARTESIAN_POINT ( 'NONE',  ( 157.9999999999998010, 238.5551250525490161, -45.00000000000000000 ) ) ;
#6546=ORIENTED_EDGE ( 'NONE', *, *, #19029, .F. ) ;
#6547=VECTOR ( 'NONE', #4849, 1000.000000000000000 ) ;
#6548=ORIENTED_EDGE ( 'NONE', *, *, #12748, .T. ) ;
#6552=VECTOR ( 'NONE', #1431, 1000.000000000000000 ) ;
#6554=ADVANCED_FACE ( 'NONE', ( #4236 ), #13024, .F. ) ;
#6560=CARTESIAN_POINT ( 'NONE',  ( 158.0000000000015916, 53.48024950453520177, -45.00000000000000000 ) ) ;
#6563=CARTESIAN_POINT ( 'NONE',  ( 157.9999999999999432, 213.4763749774776045, 45.00000000000000000 ) ) ;
#6566=CARTESIAN_POINT ( 'NONE',  ( 158.0000000000016200, 52.97237449702815582, -45.00000000000000000 ) ) ;
#6569=CARTESIAN_POINT ( 'NONE',  ( 158.0000000000015064, 63.00387452705633251, 45.00000000000000000 ) ) ;
#6570=VERTEX_POINT ( 'NONE', #1934 ) ;
#6572=CARTESIAN_POINT ( 'NONE',  ( 157.9999999999998863, 218.4921249924925348, 45.00000000000000000 ) ) ;
#6576=DIRECTION ( 'NONE',  ( -0.8916010070299268397, 0.4528218681371523058, 0.000000000000000000 ) ) ;
#6578=ORIENTED_EDGE ( 'NONE', *, *, #21278, .T. ) ;
#6580=ORIENTED_EDGE ( 'NONE', *, *, #24671, .F. ) ;
#6585=VERTEX_POINT ( 'NONE', #19469 ) ;
#6587=DIRECTION ( 'NONE',  ( -0.8916010070293584056, 0.4528218681382713551, 0.000000000000000000 ) ) ;
#6588=VECTOR ( 'NONE', #5487, 1000.000000000000000 ) ;
#6597=CARTESIAN_POINT ( 'NONE',  ( 158.0000000000014211, 70.52749954957745615, 45.00000000000000000 ) ) ;
#6602=CARTESIAN_POINT ( 'NONE',  ( 157.4999999999998295, 226.2696875187675118, -45.00000000000000000 ) ) ;
#6603=CARTESIAN_POINT ( 'NONE',  ( 157.4999999999998579, 128.4625622259929401, 45.00000000000000000 ) ) ;
#6605=DIRECTION ( 'NONE',  ( 0.4528218681373908372, -0.8916010070298056034, 0.000000000000000000 ) ) ;
#6606=VERTEX_POINT ( 'NONE', #11286 ) ;
#6615=EDGE_LOOP ( 'NONE', ( #17187, #15860, #25463, #15884 ) ) ;
#6618=DIRECTION ( 'NONE',  ( 0.4528218681379115873, 0.8916010070295411483, -0.000000000000000000 ) ) ;
#6619=EDGE_LOOP ( 'NONE', ( #1726, #7376, #16041, #18394 ) ) ;
#6622=ORIENTED_EDGE ( 'NONE', *, *, #13788, .F. ) ;
#6623=EDGE_CURVE ( 'NONE', #19117, #13806, #217, .T. ) ;
#6628=ADVANCED_FACE ( 'NONE', ( #2645 ), #4938, .F. ) ;
#6631=DIRECTION ( 'NONE',  ( 1.000000000000000000, 0.000000000000000000, -0.000000000000000000 ) ) ;
#6634=EDGE_LOOP ( 'NONE', ( #4485, #16006, #25241, #26036 ) ) ;
#6637=DIRECTION ( 'NONE',  ( -0.000000000000000000, 0.000000000000000000, -1.000000000000000000 ) ) ;
#6638=LINE ( 'NONE', #11242, #12153 ) ;
#6639=EDGE_LOOP ( 'NONE', ( #18430, #1525, #27539, #28121 ) ) ;
#6645=ORIENTED_EDGE ( 'NONE', *, *, #12584, .T. ) ;
#6647=DIRECTION ( 'NONE',  ( 0.000000000000000000, -1.000000000000000000, 0.000000000000000000 ) ) ;
#6651=ORIENTED_EDGE ( 'NONE', *, *, #16592, .F. ) ;
#6654=EDGE_CURVE ( 'NONE', #2475, #19162, #650, .T. ) ;
#6656=ORIENTED_EDGE ( 'NONE', *, *, #16032, .T. ) ;
#6657=ORIENTED_EDGE ( 'NONE', *, *, #1533, .F. ) ;
#6658=LINE ( 'NONE', #26464, #7018 ) ;
#6659=EDGE_CURVE ( 'NONE', #8035, #9517, #6955, .T. ) ;
#6660=EDGE_CURVE ( 'NONE', #7521, #6404, #22192, .T. ) ;
#6664=CARTESIAN_POINT ( 'NONE',  ( 158.0000000000008811, 121.1928747072253572, -45.00000000000000000 ) ) ;
#6667=CARTESIAN_POINT ( 'NONE',  ( 157.9999999999996305, 281.6968751876750616, 45.00000000000000000 ) ) ;
#6672=CARTESIAN_POINT ( 'NONE',  ( 158.0000000000017337, 42.94087446699998623, 45.00000000000000000 ) ) ;
#6675=CARTESIAN_POINT ( 'NONE',  ( 158.0000000000013927, 73.54324956459154805, -45.00000000000000000 ) ) ;
#6682=ORIENTED_EDGE ( 'NONE', *, *, #1268, .F. ) ;
#6684=ORIENTED_EDGE ( 'NONE', *, *, #14307, .T. ) ;
#6685=DIRECTION ( 'NONE',  ( -0.8916010070293483025, -0.4528218681382912281, 0.000000000000000000 ) ) ;
#6691=VERTEX_POINT ( 'NONE', #27066 ) ;
#6693=ORIENTED_EDGE ( 'NONE', *, *, #13132, .T. ) ;
#6701=CYLINDRICAL_SURFACE ( 'NONE', #2115, 6.000000000000005329 ) ;
#6703=CARTESIAN_POINT ( 'NONE',  ( 158.0000000000004832, 163.3188748273380213, 45.00000000000000000 ) ) ;
#6708=LINE ( 'NONE', #4548, #27063 ) ;
#6709=CARTESIAN_POINT ( 'NONE',  ( 158.0000000000007674, 133.2243747372535267, -45.00000000000000000 ) ) ;
#6713=EDGE_CURVE ( 'NONE', #16287, #26306, #18454, .T. ) ;
#6714=EDGE_CURVE ( 'NONE', #9424, #21781, #5796, .T. ) ;
#6715=CARTESIAN_POINT ( 'NONE',  ( 158.0000000000014211, 68.52749954957745615, 45.00000000000000000 ) ) ;
#6718=EDGE_LOOP ( 'NONE', ( #9735, #17642, #4204, #10334 ) ) ;
#6721=EDGE_LOOP ( 'NONE', ( #1698, #7942, #1319, #3066 ) ) ;
#6726=DIRECTION ( 'NONE',  ( -0.000000000000000000, -0.000000000000000000, -1.000000000000000000 ) ) ;
#6727=ADVANCED_FACE ( 'NONE', ( #25606 ), #1066, .F. ) ;
#6729=DIRECTION ( 'NONE',  ( 0.000000000000000000, 0.000000000000000000, 1.000000000000000000 ) ) ;
#6730=DIRECTION ( 'NONE',  ( -0.8916010070296733758, -0.4528218681376511845, 0.000000000000000000 ) ) ;
#6732=DIRECTION ( 'NONE',  ( -0.8916010070300285362, -0.4528218681369517995, 0.000000000000000000 ) ) ;
#6734=DIRECTION ( 'NONE',  ( -0.8916010070293783896, 0.4528218681382319422, 0.000000000000000000 ) ) ;
#6743=EDGE_CURVE ( 'NONE', #20893, #5272, #7815, .T. ) ;
#6745=AXIS2_PLACEMENT_3D ( 'NONE', #25804, #6130, #14905 ) ;
#6746=CARTESIAN_POINT ( 'NONE',  ( 158.0000000000001421, 193.4133749174225443, 45.00000000000000000 ) ) ;
#6753=CARTESIAN_POINT ( 'NONE',  ( 157.4999999999998579, 118.4310621959647563, 45.00000000000000000 ) ) ;
#6755=ORIENTED_EDGE ( 'NONE', *, *, #4388, .T. ) ;
#6761=VECTOR ( 'NONE', #17221, 1000.000000000000000 ) ;
#6762=LINE ( 'NONE', #4748, #21720 ) ;
#6766=ORIENTED_EDGE ( 'NONE', *, *, #6654, .F. ) ;
#6769=CARTESIAN_POINT ( 'NONE',  ( 158.0000000000000853, 198.9369999399436892, 45.00000000000000000 ) ) ;
#6770=CARTESIAN_POINT ( 'NONE',  ( 157.9999999999997158, 263.6338751276190351, 45.00000000000000000 ) ) ;
#6771=EDGE_LOOP ( 'NONE', ( #12390, #23397, #20599, #11105 ) ) ;
#6772=LINE ( 'NONE', #26028, #2733 ) ;
#6778=ORIENTED_EDGE ( 'NONE', *, *, #10204, .F. ) ;
#6779=( NAMED_UNIT ( * ) SI_UNIT ( $, .STERADIAN. ) SOLID_ANGLE_UNIT ( ) );
#6781=EDGE_CURVE ( 'NONE', #1313, #18620, #22902, .T. ) ;
#6783=DIRECTION ( 'NONE',  ( 0.4528218681382713551, 0.8916010070293584056, -0.000000000000000000 ) ) ;
#6793=LINE ( 'NONE', #2334, #14842 ) ;
#6795=VECTOR ( 'NONE', #17128, 1000.000000000000114 ) ;
#6797=LINE ( 'NONE', #2920, #15361 ) ;
#6798=PLANE ( 'NONE',  #11744 ) ;
#6802=ORIENTED_EDGE ( 'NONE', *, *, #23855, .T. ) ;
#6804=LINE ( 'NONE', #4228, #20268 ) ;
#6805=CARTESIAN_POINT ( 'NONE',  ( 187.4999999999996305, 288.9665627064425166, 45.00000000000000000 ) ) ;
#6809=EDGE_LOOP ( 'NONE', ( #8133, #13894, #856, #5510 ) ) ;
#6812=DIRECTION ( 'NONE',  ( -0.8916010070293584056, 0.4528218681382713551, 0.000000000000000000 ) ) ;
#6821=EDGE_LOOP ( 'NONE', ( #23477, #17707, #8604, #27408 ) ) ;
#6825=ORIENTED_EDGE ( 'NONE', *, *, #21387, .F. ) ;
#6826=ORIENTED_EDGE ( 'NONE', *, *, #23299, .T. ) ;
#6827=DIRECTION ( 'NONE',  ( 0.8916010070294800860, -0.4528218681380314359, 0.000000000000000000 ) ) ;
#6830=ORIENTED_EDGE ( 'NONE', *, *, #20422, .T. ) ;
#6831=ORIENTED_EDGE ( 'NONE', *, *, #11017, .F. ) ;
#6832=LINE ( 'NONE', #12893, #13680 ) ;
#6839=VECTOR ( 'NONE', #18939, 1000.000000000000114 ) ;
#6843=CARTESIAN_POINT ( 'NONE',  ( 158.0000000000000000, 208.4606249624626457, 45.00000000000000000 ) ) ;
#6845=LINE ( 'NONE', #26660, #20560 ) ;
#6851=CARTESIAN_POINT ( 'NONE',  ( 157.4999999999998579, 153.5413123010633853, 45.00000000000000000 ) ) ;
#6857=VERTEX_POINT ( 'NONE', #12424 ) ;
#6859=CARTESIAN_POINT ( 'NONE',  ( 158.0000000000009948, 108.6534996696901345, -45.00000000000000000 ) ) ;
#6862=ORIENTED_EDGE ( 'NONE', *, *, #17460, .T. ) ;
#6866=ORIENTED_EDGE ( 'NONE', *, *, #22705, .T. ) ;
#6868=ORIENTED_EDGE ( 'NONE', *, *, #18826, .F. ) ;
#6871=AXIS2_PLACEMENT_3D ( 'NONE', #2552, #17500, #11339 ) ;
#6872=DIRECTION ( 'NONE',  ( -0.000000000000000000, 0.000000000000000000, -1.000000000000000000 ) ) ;
#6874=ADVANCED_FACE ( 'NONE', ( #21586 ), #25746, .F. ) ;
#6879=PLANE ( 'NONE',  #14500 ) ;
#6881=DIRECTION ( 'NONE',  ( 0.4528218681376312005, 0.8916010070296835899, -0.000000000000000000 ) ) ;
#6885=LINE ( 'NONE', #8622, #899 ) ;
#6886=LINE ( 'NONE', #4724, #6018 ) ;
#6891=CARTESIAN_POINT ( 'NONE',  ( 157.4999999999994884, 211.2224374737238577, -45.00000000000000000 ) ) ;
#6901=ORIENTED_EDGE ( 'NONE', *, *, #276, .F. ) ;
#6902=ORIENTED_EDGE ( 'NONE', *, *, #2440, .F. ) ;
#6904=DIRECTION ( 'NONE',  ( -0.000000000000000000, -0.000000000000000000, -1.000000000000000000 ) ) ;
#6909=EDGE_CURVE ( 'NONE', #11282, #7826, #19147, .T. ) ;
#6910=LINE ( 'NONE', #4750, #16728 ) ;
#6914=AXIS2_PLACEMENT_3D ( 'NONE', #3617, #16846, #14693 ) ;
#6916=EDGE_CURVE ( 'NONE', #5026, #26072, #21441, .T. ) ;
#6918=DIRECTION ( 'NONE',  ( -0.000000000000000000, -0.000000000000000000, -1.000000000000000000 ) ) ;
#6924=LINE ( 'NONE', #24308, #13090 ) ;
#6926=ORIENTED_EDGE ( 'NONE', *, *, #4183, .T. ) ;
#6929=ORIENTED_EDGE ( 'NONE', *, *, #8957, .F. ) ;
#6933=CARTESIAN_POINT ( 'NONE',  ( 157.4999999999998579, 188.6515624061619576, 45.00000000000000000 ) ) ;
#6934=ORIENTED_EDGE ( 'NONE', *, *, #13626, .F. ) ;
#6939=DIRECTION ( 'NONE',  ( 0.4528218681378916588, 0.8916010070295512513, -0.000000000000000000 ) ) ;
#6945=ORIENTED_EDGE ( 'NONE', *, *, #956, .F. ) ;
#6947=DIRECTION ( 'NONE',  ( 0.8916010070293383105, -0.4528218681383106015, 0.000000000000000000 ) ) ;
#6951=CARTESIAN_POINT ( 'NONE',  ( 158.0000000000007105, 136.2401247522676044, -45.00000000000000000 ) ) ;
#6953=VECTOR ( 'NONE', #26311, 1000.000000000000000 ) ;
#6955=LINE ( 'NONE', #26787, #9664 ) ;
#6960=VECTOR ( 'NONE', #6083, 1000.000000000000114 ) ;
#6967=EDGE_LOOP ( 'NONE', ( #10705, #9354, #17530, #10365 ) ) ;
#6968=DIRECTION ( 'NONE',  ( -0.000000000000000000, 0.000000000000000000, -1.000000000000000000 ) ) ;
#6975=DIRECTION ( 'NONE',  ( -0.000000000000000000, -0.000000000000000000, -1.000000000000000000 ) ) ;
#6978=AXIS2_PLACEMENT_3D ( 'NONE', #26508, #4536, #22507 ) ;
#6980=ADVANCED_FACE ( 'NONE', ( #20686 ), #25556, .F. ) ;
#6989=FACE_OUTER_BOUND ( 'NONE', #26027, .T. ) ;
#6990=LINE ( 'NONE', #24948, #13236 ) ;
#6993=CARTESIAN_POINT ( 'NONE',  ( 158.0000000000016200, 50.97237449702815582, -45.00000000000000000 ) ) ;
#6995=CARTESIAN_POINT ( 'NONE',  ( 157.9999999999997726, 244.0787500750700474, 45.00000000000000000 ) ) ;
#6998=VECTOR ( 'NONE', #1456, 1000.000000000000000 ) ;
#7001=ORIENTED_EDGE ( 'NONE', *, *, #10419, .T. ) ;
#7004=VECTOR ( 'NONE', #8900, 1000.000000000000114 ) ;
#7008=ORIENTED_EDGE ( 'NONE', *, *, #23480, .F. ) ;
#7009=VERTEX_POINT ( 'NONE', #10061 ) ;
#7010=VERTEX_POINT ( 'NONE', #25701 ) ;
#7011=ORIENTED_EDGE ( 'NONE', *, *, #9233, .F. ) ;
#7013=CARTESIAN_POINT ( 'NONE',  ( 158.0000000000009663, 115.6692496847042264, 45.00000000000000000 ) ) ;
#7018=VECTOR ( 'NONE', #15439, 1000.000000000000114 ) ;
#7020=CARTESIAN_POINT ( 'NONE',  ( 158.0000000000003979, 170.8424998498591663, 45.00000000000000000 ) ) ;
#7024=LINE ( 'NONE', #17942, #15425 ) ;
#7025=LINE ( 'NONE', #13219, #2975 ) ;
#7027=DIRECTION ( 'NONE',  ( -1.000000000000000000, 0.000000000000000000, 0.000000000000000000 ) ) ;
#7028=FACE_OUTER_BOUND ( 'NONE', #1628, .T. ) ;
#7031=EDGE_CURVE ( 'NONE', #1602, #21761, #5457, .T. ) ;
#7034=CARTESIAN_POINT ( 'NONE',  ( 158.0000000000004832, 161.3188748273380213, -45.00000000000000000 ) ) ;
#7041=ORIENTED_EDGE ( 'NONE', *, *, #7857, .F. ) ;
#7048=EDGE_LOOP ( 'NONE', ( #10122, #5474, #10610, #10549 ) ) ;
#7054=EDGE_LOOP ( 'NONE', ( #22037, #8879, #3959, #23191 ) ) ;
#7058=DIRECTION ( 'NONE',  ( -0.000000000000000000, -0.000000000000000000, -1.000000000000000000 ) ) ;
#7060=VECTOR ( 'NONE', #17293, 1000.000000000000000 ) ;
#7062=EDGE_CURVE ( 'NONE', #17988, #21244, #23274, .T. ) ;
#7064=DIRECTION ( 'NONE',  ( 0.4528218681378310406, 0.8916010070295820045, -0.000000000000000000 ) ) ;
#7068=ORIENTED_EDGE ( 'NONE', *, *, #19112, .F. ) ;
#7070=DIRECTION ( 'NONE',  ( 0.8916010070300383061, -0.4528218681369324261, 0.000000000000000000 ) ) ;
#7075=EDGE_CURVE ( 'NONE', #16487, #5204, #17438, .T. ) ;
#7080=ORIENTED_EDGE ( 'NONE', *, *, #169, .T. ) ;
#7082=VERTEX_POINT ( 'NONE', #10908 ) ;
#7086=DIRECTION ( 'NONE',  ( 1.000000000000000000, 0.000000000000000000, -0.000000000000000000 ) ) ;
#7091=CARTESIAN_POINT ( 'NONE',  ( 158.0000000000001705, 188.9054999099155054, 45.00000000000000000 ) ) ;
#7093=FACE_OUTER_BOUND ( 'NONE', #26477, .T. ) ;
#7094=EDGE_CURVE ( 'NONE', #26492, #18389, #26406, .T. ) ;
#7095=LINE ( 'NONE', #20453, #11958 ) ;
#7098=EDGE_CURVE ( 'NONE', #7888, #6230, #129, .T. ) ;
#7101=CARTESIAN_POINT ( 'NONE',  ( 158.0000000000009663, 113.6692496847042264, -45.00000000000000000 ) ) ;
#7102=LINE ( 'NONE', #11281, #21728 ) ;
#7105=DIRECTION ( 'NONE',  ( -0.8916010070298968637, -0.4528218681372109811, 0.000000000000000000 ) ) ;
#7107=CARTESIAN_POINT ( 'NONE',  ( 157.4999999999996874, 268.9035626463865469, 45.00000000000000000 ) ) ;
#7110=EDGE_LOOP ( 'NONE', ( #19014, #2314, #10295, #2441 ) ) ;
#7116=ORIENTED_EDGE ( 'NONE', *, *, #20387, .T. ) ;
#7117=CARTESIAN_POINT ( 'NONE',  ( 158.0000000000004263, 166.3346248423521274, 45.00000000000000000 ) ) ;
#7122=FACE_OUTER_BOUND ( 'NONE', #3966, .T. ) ;
#7124=VECTOR ( 'NONE', #9285, 1000.000000000000114 ) ;
#7129=CARTESIAN_POINT ( 'NONE',  ( 158.0000000000015916, 55.48024950453520177, -45.00000000000000000 ) ) ;
#7130=PLANE ( 'NONE',  #16089 ) ;
#7132=DIRECTION ( 'NONE',  ( 0.000000000000000000, -1.000000000000000000, 0.000000000000000000 ) ) ;
#7133=DIRECTION ( 'NONE',  ( 0.000000000000000000, 1.000000000000000000, -0.000000000000000000 ) ) ;
#7135=CARTESIAN_POINT ( 'NONE',  ( 158.0000000000006821, 138.7479997597746433, -45.00000000000000000 ) ) ;
#7136=CARTESIAN_POINT ( 'NONE',  ( 158.0000000000011937, 91.09837461714084839, 45.00000000000000000 ) ) ;
#7137=CARTESIAN_POINT ( 'NONE',  ( 158.0000000000012221, 90.59049960963380954, 45.00000000000000000 ) ) ;
#7142=FACE_OUTER_BOUND ( 'NONE', #13631, .T. ) ;
#7144=VECTOR ( 'NONE', #8813, 1000.000000000000227 ) ;
#7151=DIRECTION ( 'NONE',  ( -0.8916010070297041290, -0.4528218681375906218, 0.000000000000000000 ) ) ;
#7152=ADVANCED_FACE ( 'NONE', ( #8471 ), #19530, .F. ) ;
#7153=VECTOR ( 'NONE', #28000, 1000.000000000000000 ) ;
#7158=ORIENTED_EDGE ( 'NONE', *, *, #22289, .T. ) ;
#7159=VERTEX_POINT ( 'NONE', #17503 ) ;
#7162=CARTESIAN_POINT ( 'NONE',  ( 158.0000000000007105, 138.2401247522676044, -45.00000000000000000 ) ) ;
#7163=PLANE ( 'NONE',  #22936 ) ;
#7164=VECTOR ( 'NONE', #13793, 1000.000000000000114 ) ;
#7166=VECTOR ( 'NONE', #19904, 1000.000000000000000 ) ;
#7175=CARTESIAN_POINT ( 'NONE',  ( 158.0000000000000568, 201.4448749474510407, -45.00000000000000000 ) ) ;
#7176=DIRECTION ( 'NONE',  ( -0.8916010070296834789, 0.4528218681376311450, 0.000000000000000000 ) ) ;
#7178=CARTESIAN_POINT ( 'NONE',  ( 157.9999999999996874, 271.1575001501400379, 45.00000000000000000 ) ) ;
#7179=LINE ( 'NONE', #7608, #27482 ) ;
#7181=DIRECTION ( 'NONE',  ( 0.000000000000000000, -1.000000000000000000, 0.000000000000000000 ) ) ;
#7184=CARTESIAN_POINT ( 'NONE',  ( 158.0000000000015064, 61.00387452705632541, 45.00000000000000000 ) ) ;
#7186=CARTESIAN_POINT ( 'NONE',  ( 157.4999999999998579, 68.27356204582390831, -45.00000000000000000 ) ) ;
#7195=EDGE_CURVE ( 'NONE', #3903, #20000, #26125, .T. ) ;
#7198=EDGE_LOOP ( 'NONE', ( #1593, #1837, #13854, #6684 ) ) ;
#7201=CARTESIAN_POINT ( 'NONE',  ( 157.9999999999996305, 284.2047501951820436, 45.00000000000000000 ) ) ;
#7204=LINE ( 'NONE', #11528, #8421 ) ;
#7207=AXIS2_PLACEMENT_3D ( 'NONE', #7894, #18537, #1144 ) ;
#7211=EDGE_CURVE ( 'NONE', #17167, #21241, #17225, .T. ) ;
#7213=LINE ( 'NONE', #27162, #11124 ) ;
#7214=CARTESIAN_POINT ( 'NONE',  ( 158.0000000000014779, 65.51174953456337846, -45.00000000000000000 ) ) ;
#7217=EDGE_CURVE ( 'NONE', #543, #12064, #11052, .T. ) ;
#7219=CARTESIAN_POINT ( 'NONE',  ( 157.4999999999995737, 203.6988124512014338, -45.00000000000000000 ) ) ;
#7220=ORIENTED_EDGE ( 'NONE', *, *, #22633, .T. ) ;
#7225=EDGE_CURVE ( 'NONE', #12854, #12943, #21828, .T. ) ;
#7228=VERTEX_POINT ( 'NONE', #17481 ) ;
#7240=PLANE ( 'NONE',  #16457 ) ;
#7241=EDGE_CURVE ( 'NONE', #23120, #5724, #4408, .T. ) ;
#7242=DIRECTION ( 'NONE',  ( 0.4528218681382319422, 0.8916010070293783896, -0.000000000000000000 ) ) ;
#7243=DIRECTION ( 'NONE',  ( -0.000000000000000000, 0.000000000000000000, -1.000000000000000000 ) ) ;
#7246=CARTESIAN_POINT ( 'NONE',  ( 157.4999999999998295, 228.7775625262745223, 45.00000000000000000 ) ) ;
#7247=PLANE ( 'NONE',  #22882 ) ;
#7252=ORIENTED_EDGE ( 'NONE', *, *, #13358, .F. ) ;
#7253=ADVANCED_FACE ( 'NONE', ( #6428 ), #26663, .F. ) ;
#7259=CARTESIAN_POINT ( 'NONE',  ( 157.4999999999994600, 213.7303124812313513, 45.00000000000000000 ) ) ;
#7261=CARTESIAN_POINT ( 'NONE',  ( 157.9999999999997442, 251.0945000900840398, 45.00000000000000000 ) ) ;
#7262=ORIENTED_EDGE ( 'NONE', *, *, #9265, .F. ) ;
#7265=ORIENTED_EDGE ( 'NONE', *, *, #10390, .F. ) ;
#7267=DIRECTION ( 'NONE',  ( -0.000000000000000000, 0.000000000000000000, -1.000000000000000000 ) ) ;
#7271=ORIENTED_EDGE ( 'NONE', *, *, #4602, .F. ) ;
#7273=FACE_OUTER_BOUND ( 'NONE', #7858, .T. ) ;
#7274=CARTESIAN_POINT ( 'NONE',  ( 158.0000000000005400, 158.3031248123239436, 45.00000000000000000 ) ) ;
#7275=LINE ( 'NONE', #20199, #5952 ) ;
#7280=( GEOMETRIC_REPRESENTATION_CONTEXT ( 3 ) GLOBAL_UNCERTAINTY_ASSIGNED_CONTEXT ( ( #11776 ) ) GLOBAL_UNIT_ASSIGNED_CONTEXT ( ( #25645, #23643, #10571 ) ) REPRESENTATION_CONTEXT ( 'NONE', 'WORKASPACE' ) );
#7282=DIRECTION ( 'NONE',  ( 0.4528218681369324261, 0.8916010070300384172, -0.000000000000000000 ) ) ;
#7285=DIRECTION ( 'NONE',  ( -0.000000000000000000, -0.000000000000000000, -1.000000000000000000 ) ) ;
#7291=CARTESIAN_POINT ( 'NONE',  ( 158.0000000000014495, 66.01962454207041731, 45.00000000000000000 ) ) ;
#7296=DIRECTION ( 'NONE',  ( 0.8916010070293783896, -0.4528218681382319422, 0.000000000000000000 ) ) ;
#7298=LINE ( 'NONE', #3107, #17806 ) ;
#7299=ORIENTED_EDGE ( 'NONE', *, *, #24814, .F. ) ;
#7302=ORIENTED_EDGE ( 'NONE', *, *, #15183, .T. ) ;
#7305=CARTESIAN_POINT ( 'NONE',  ( 157.4999999999995453, 206.2066874587088989, -45.00000000000000000 ) ) ;
#7307=AXIS2_PLACEMENT_3D ( 'NONE', #26781, #2781, #4500 ) ;
#7309=CARTESIAN_POINT ( 'NONE',  ( 158.0000000000010800, 103.1298746471690038, 45.00000000000000000 ) ) ;
#7312=DIRECTION ( 'NONE',  ( -0.000000000000000000, -0.000000000000000000, -1.000000000000000000 ) ) ;
#7314=CARTESIAN_POINT ( 'NONE',  ( 157.4999999999997726, 246.3326875788235384, 45.00000000000000000 ) ) ;
#7321=VECTOR ( 'NONE', #28031, 1000.000000000000227 ) ;
#7329=CARTESIAN_POINT ( 'NONE',  ( 157.4999999999998579, 45.70268697826052318, 45.00000000000000000 ) ) ;
#7332=VERTEX_POINT ( 'NONE', #6993 ) ;
#7338=ADVANCED_FACE ( 'NONE', ( #26099 ), #105, .F. ) ;
#7340=ORIENTED_EDGE ( 'NONE', *, *, #18925, .T. ) ;
#7341=DIRECTION ( 'NONE',  ( 0.4528218681374511223, -0.8916010070297750723, 0.000000000000000000 ) ) ;
#7342=DIRECTION ( 'NONE',  ( -0.8916010070294396739, 0.4528218681381114274, 0.000000000000000000 ) ) ;
#7344=EDGE_CURVE ( 'NONE', #5313, #22382, #17340, .T. ) ;
#7350=DIRECTION ( 'NONE',  ( -0.000000000000000000, -0.000000000000000000, -1.000000000000000000 ) ) ;
#7351=ADVANCED_FACE ( 'NONE', ( #2387 ), #9012, .F. ) ;
#7354=ADVANCED_FACE ( 'NONE', ( #10888 ), #19643, .F. ) ;
#7356=EDGE_CURVE ( 'NONE', #17304, #23194, #7945, .T. ) ;
#7357=LINE ( 'NONE', #174, #16569 ) ;
#7359=PLANE ( 'NONE',  #28148 ) ;
#7360=ORIENTED_EDGE ( 'NONE', *, *, #12545, .T. ) ;
#7362=VECTOR ( 'NONE', #17053, 1000.000000000000000 ) ;
#7364=ORIENTED_EDGE ( 'NONE', *, *, #27187, .F. ) ;
#7371=FACE_OUTER_BOUND ( 'NONE', #24890, .T. ) ;
#7375=DIRECTION ( 'NONE',  ( -0.000000000000000000, 0.000000000000000000, -1.000000000000000000 ) ) ;
#7376=ORIENTED_EDGE ( 'NONE', *, *, #9594, .F. ) ;
#7383=DIRECTION ( 'NONE',  ( -0.8916010070299070778, -0.4528218681371909971, 0.000000000000000000 ) ) ;
#7386=DIRECTION ( 'NONE',  ( -0.8916010070293783896, -0.4528218681382319422, 0.000000000000000000 ) ) ;
#7388=LINE ( 'NONE', #24624, #12693 ) ;
#7391=EDGE_CURVE ( 'NONE', #4479, #2548, #16851, .T. ) ;
#7396=CARTESIAN_POINT ( 'NONE',  ( 157.9999999999997726, 241.5708750675630370, -45.00000000000000000 ) ) ;
#7397=EDGE_LOOP ( 'NONE', ( #11594, #16984, #12319, #19270 ) ) ;
#7400=CARTESIAN_POINT ( 'NONE',  ( 158.0000000000013358, 78.55899957960562574, 45.00000000000000000 ) ) ;
#7406=DIRECTION ( 'NONE',  ( 0.000000000000000000, -1.000000000000000000, 0.000000000000000000 ) ) ;
#7407=FACE_OUTER_BOUND ( 'NONE', #6721, .T. ) ;
#7413=ORIENTED_EDGE ( 'NONE', *, *, #28331, .T. ) ;
#7417=CARTESIAN_POINT ( 'NONE',  ( 158.0000000000000284, 203.9527499549551806, 45.00000000000000000 ) ) ;
#7418=DIRECTION ( 'NONE',  ( -0.000000000000000000, -0.000000000000000000, -1.000000000000000000 ) ) ;
#7419=LINE ( 'NONE', #27226, #16107 ) ;
#7423=CARTESIAN_POINT ( 'NONE',  ( 158.0000000000009663, 115.6692496847042264, -45.00000000000000000 ) ) ;
#7431=EDGE_CURVE ( 'NONE', #23450, #9316, #10108, .T. ) ;
#7436=ORIENTED_EDGE ( 'NONE', *, *, #28125, .F. ) ;
#7437=CARTESIAN_POINT ( 'NONE',  ( 157.4999999999998579, 88.33656210588026170, 45.00000000000000000 ) ) ;
#7441=ORIENTED_EDGE ( 'NONE', *, *, #7356, .T. ) ;
#7448=CARTESIAN_POINT ( 'NONE',  ( 157.4999999999998579, 55.73418700828869277, -45.00000000000000000 ) ) ;
#7453=EDGE_CURVE ( 'NONE', #19895, #11442, #18720, .T. ) ;
#7455=DIRECTION ( 'NONE',  ( -0.8916010070293283185, -0.4528218681383305855, 0.000000000000000000 ) ) ;
#7460=CARTESIAN_POINT ( 'NONE',  ( 158.0000000000011369, 98.11412463215494029, 45.00000000000000000 ) ) ;
#7462=PLANE ( 'NONE',  #18274 ) ;
#7464=VECTOR ( 'NONE', #26596, 1000.000000000000114 ) ;
#7471=VECTOR ( 'NONE', #2959, 1000.000000000000000 ) ;
#7473=ORIENTED_EDGE ( 'NONE', *, *, #12545, .F. ) ;
#7477=VERTEX_POINT ( 'NONE', #8088 ) ;
#7481=VERTEX_POINT ( 'NONE', #23452 ) ;
#7482=CARTESIAN_POINT ( 'NONE',  ( 158.0000000000003411, 173.8582498648732440, 45.00000000000000000 ) ) ;
#7483=EDGE_CURVE ( 'NONE', #26789, #26868, #18065, .T. ) ;
#7487=VECTOR ( 'NONE', #21620, 1000.000000000000000 ) ;
#7489=ADVANCED_FACE ( 'NONE', ( #2820 ), #20354, .F. ) ;
#7491=DIRECTION ( 'NONE',  ( 0.8916010070298961976, -0.4528218681372121468, 0.000000000000000000 ) ) ;
#7492=VECTOR ( 'NONE', #13885, 1000.000000000000000 ) ;
#7493=FACE_OUTER_BOUND ( 'NONE', #4354, .T. ) ;
#7494=CARTESIAN_POINT ( 'NONE',  ( 158.0000000000011369, 98.11412463215494029, 45.00000000000000000 ) ) ;
#7497=DIRECTION ( 'NONE',  ( -0.8916010070297846202, 0.4528218681374320820, 0.000000000000000000 ) ) ;
#7503=VECTOR ( 'NONE', #17841, 1000.000000000000000 ) ;
#7508=VECTOR ( 'NONE', #15488, 1000.000000000000000 ) ;
#7511=CARTESIAN_POINT ( 'NONE',  ( 158.0000000000004263, 168.3346248423521274, -45.00000000000000000 ) ) ;
#7512=ORIENTED_EDGE ( 'NONE', *, *, #546, .F. ) ;
#7515=EDGE_CURVE ( 'NONE', #5835, #4162, #28027, .T. ) ;
#7517=EDGE_CURVE ( 'NONE', #14722, #7676, #3907, .T. ) ;
#7518=CARTESIAN_POINT ( 'NONE',  ( 157.9999999999996874, 271.1575001501400379, 45.00000000000000000 ) ) ;
#7519=EDGE_CURVE ( 'NONE', #16964, #4623, #21578, .T. ) ;
#7521=VERTEX_POINT ( 'NONE', #21433 ) ;
#7524=VECTOR ( 'NONE', #24439, 1000.000000000000000 ) ;
#7525=DIRECTION ( 'NONE',  ( -0.000000000000000000, -0.000000000000000000, -1.000000000000000000 ) ) ;
#7526=VECTOR ( 'NONE', #2619, 1000.000000000000000 ) ;
#7527=DIRECTION ( 'NONE',  ( -0.000000000000000000, -0.000000000000000000, -1.000000000000000000 ) ) ;
#7538=ORIENTED_EDGE ( 'NONE', *, *, #15430, .F. ) ;
#7540=ORIENTED_EDGE ( 'NONE', *, *, #13135, .F. ) ;
#7541=LINE ( 'NONE', #9968, #13473 ) ;
#7544=ORIENTED_EDGE ( 'NONE', *, *, #13363, .T. ) ;
#7546=CARTESIAN_POINT ( 'NONE',  ( 157.4999999999998579, 120.9389372034718093, 45.00000000000000000 ) ) ;
#7550=ADVANCED_FACE ( 'NONE', ( #2036 ), #8369, .F. ) ;
#7555=ORIENTED_EDGE ( 'NONE', *, *, #22019, .F. ) ;
#7556=EDGE_CURVE ( 'NONE', #15387, #21202, #1890, .T. ) ;
#7560=VERTEX_POINT ( 'NONE', #1749 ) ;
#7565=CARTESIAN_POINT ( 'NONE',  ( 158.0000000000001990, 188.3976249024084666, -45.00000000000000000 ) ) ;
#7566=AXIS2_PLACEMENT_3D ( 'NONE', #26302, #24021, #13388 ) ;
#7568=DIRECTION ( 'NONE',  ( -0.000000000000000000, -0.000000000000000000, -1.000000000000000000 ) ) ;
#7569=PLANE ( 'NONE',  #21234 ) ;
#7572=CARTESIAN_POINT ( 'NONE',  ( 158.0000000000015348, 60.49599951954928656, -45.00000000000000000 ) ) ;
#7590=VERTEX_POINT ( 'NONE', #4189 ) ;
#7595=CARTESIAN_POINT ( 'NONE',  ( 157.4999999999998579, 53.22631200078164682, 45.00000000000000000 ) ) ;
#7598=CARTESIAN_POINT ( 'NONE',  ( 157.4999999999998579, 78.30506207585207790, 45.00000000000000000 ) ) ;
#7600=CARTESIAN_POINT ( 'NONE',  ( 158.0000000000012506, 88.08262460212675649, 45.00000000000000000 ) ) ;
#7601=CARTESIAN_POINT ( 'NONE',  ( 157.4999999999998579, 73.28931206083800021, 45.00000000000000000 ) ) ;
#7606=ORIENTED_EDGE ( 'NONE', *, *, #17289, .T. ) ;
#7607=ADVANCED_FACE ( 'NONE', ( #14850 ), #15413, .F. ) ;
#7608=CARTESIAN_POINT ( 'NONE',  ( 158.0000000000012221, 88.59049960963380954, 45.00000000000000000 ) ) ;
#7611=VECTOR ( 'NONE', #9200, 1000.000000000000114 ) ;
#7617=EDGE_LOOP ( 'NONE', ( #923, #16798, #3735, #7752 ) ) ;
#7618=VERTEX_POINT ( 'NONE', #17409 ) ;
#7620=VERTEX_POINT ( 'NONE', #26168 ) ;
#7621=CARTESIAN_POINT ( 'NONE',  ( 157.4999999999997158, 261.3799376238655441, 45.00000000000000000 ) ) ;
#7622=AXIS2_PLACEMENT_3D ( 'NONE', #5096, #20472, #20038 ) ;
#7626=LINE ( 'NONE', #9643, #4098 ) ;
#7627=PLANE ( 'NONE',  #10264 ) ;
#7630=DIRECTION ( 'NONE',  ( 0.4528218681374520105, 0.8916010070297746282, -0.000000000000000000 ) ) ;
#7638=AXIS2_PLACEMENT_3D ( 'NONE', #4665, #17895, #6968 ) ;
#7640=DIRECTION ( 'NONE',  ( -0.000000000000000000, 0.000000000000000000, -1.000000000000000000 ) ) ;
#7643=LINE ( 'NONE', #12104, #24582 ) ;
#7644=ORIENTED_EDGE ( 'NONE', *, *, #436, .F. ) ;
#7650=DIRECTION ( 'NONE',  ( -0.8916010070297751833, -0.4528218681374507892, 0.000000000000000000 ) ) ;
#7653=CARTESIAN_POINT ( 'NONE',  ( 157.9999999999996589, 274.1732501651540588, 45.00000000000000000 ) ) ;
#7655=CARTESIAN_POINT ( 'NONE',  ( 157.4999999999998579, 146.0176872785422404, 45.00000000000000000 ) ) ;
#7663=CARTESIAN_POINT ( 'NONE',  ( 157.4999999999998579, 161.0649373235845019, 45.00000000000000000 ) ) ;
#7664=DIRECTION ( 'NONE',  ( 0.000000000000000000, -1.000000000000000000, 0.000000000000000000 ) ) ;
#7665=CARTESIAN_POINT ( 'NONE',  ( 157.4999999999998579, 153.5413123010633853, 45.00000000000000000 ) ) ;
#7666=LINE ( 'NONE', #16432, #12435 ) ;
#7671=CARTESIAN_POINT ( 'NONE',  ( 158.0000000000010800, 101.1298746471690038, 45.00000000000000000 ) ) ;
#7672=ORIENTED_EDGE ( 'NONE', *, *, #1960, .T. ) ;
#7673=EDGE_CURVE ( 'NONE', #7009, #25157, #15985, .T. ) ;
#7675=EDGE_CURVE ( 'NONE', #4902, #8063, #7357, .T. ) ;
#7676=VERTEX_POINT ( 'NONE', #8935 ) ;
#7683=ORIENTED_EDGE ( 'NONE', *, *, #11045, .F. ) ;
#7684=AXIS2_PLACEMENT_3D ( 'NONE', #11669, #20405, #18258 ) ;
#7687=LINE ( 'NONE', #23052, #22297 ) ;
#7690=CARTESIAN_POINT ( 'NONE',  ( 157.9999999999996874, 266.6496251426330559, 45.00000000000000000 ) ) ;
#7692=EDGE_CURVE ( 'NONE', #24469, #17639, #20130, .T. ) ;
#7694=ORIENTED_EDGE ( 'NONE', *, *, #8179, .T. ) ;
#7699=DIRECTION ( 'NONE',  ( -0.000000000000000000, -0.000000000000000000, -1.000000000000000000 ) ) ;
#7701=LINE ( 'NONE', #27359, #3223 ) ;
#7702=CARTESIAN_POINT ( 'NONE',  ( 157.9999999999999147, 213.9842499849850697, 45.00000000000000000 ) ) ;
#7703=DIRECTION ( 'NONE',  ( -0.8916010070294301260, -0.4528218681381301347, 0.000000000000000000 ) ) ;
#7705=EDGE_CURVE ( 'NONE', #26626, #20330, #27022, .T. ) ;
#7706=CARTESIAN_POINT ( 'NONE',  ( 158.0000000000005400, 155.7952498048169048, -45.00000000000000000 ) ) ;
#7713=DIRECTION ( 'NONE',  ( 0.4528218681378110011, -0.8916010070295922185, 0.000000000000000000 ) ) ;
#7716=ORIENTED_EDGE ( 'NONE', *, *, #701, .F. ) ;
#7723=ORIENTED_EDGE ( 'NONE', *, *, #448, .F. ) ;
#7724=ORIENTED_EDGE ( 'NONE', *, *, #1867, .F. ) ;
#7726=PLANE ( 'NONE',  #20515 ) ;
#7737=LINE ( 'NONE', #25113, #16743 ) ;
#7741=ORIENTED_EDGE ( 'NONE', *, *, #3838, .F. ) ;
#7742=EDGE_CURVE ( 'NONE', #8983, #23817, #20555, .T. ) ;
#7744=DIRECTION ( 'NONE',  ( 0.000000000000000000, -1.000000000000000000, 0.000000000000000000 ) ) ;
#7745=LINE ( 'NONE', #14359, #15758 ) ;
#7752=ORIENTED_EDGE ( 'NONE', *, *, #12448, .T. ) ;
#7753=ORIENTED_EDGE ( 'NONE', *, *, #27498, .F. ) ;
#7755=VECTOR ( 'NONE', #14979, 1000.000000000000000 ) ;
#7756=ORIENTED_EDGE ( 'NONE', *, *, #23297, .F. ) ;
#7762=DIRECTION ( 'NONE',  ( 0.8916010070298455714, -0.4528218681373120669, 0.000000000000000000 ) ) ;
#7767=CARTESIAN_POINT ( 'NONE',  ( 158.0000000000017053, 43.44874947450702507, 45.00000000000000000 ) ) ;
#7777=ADVANCED_FACE ( 'NONE', ( #880 ), #18409, .F. ) ;
#7780=ORIENTED_EDGE ( 'NONE', *, *, #13847, .F. ) ;
#7781=ORIENTED_EDGE ( 'NONE', *, *, #15351, .T. ) ;
#7782=LINE ( 'NONE', #23430, #1926 ) ;
#7785=ORIENTED_EDGE ( 'NONE', *, *, #10298, .F. ) ;
#7797=PLANE ( 'NONE',  #20919 ) ;
#7800=CARTESIAN_POINT ( 'NONE',  ( 157.9999999999997726, 246.5866250825770294, 45.00000000000000000 ) ) ;
#7801=PLANE ( 'NONE',  #20068 ) ;
#7805=AXIS2_PLACEMENT_3D ( 'NONE', #22071, #9002, #19768 ) ;
#7808=CARTESIAN_POINT ( 'NONE',  ( 157.9999999999998579, 223.5078750075070104, 45.00000000000000000 ) ) ;
#7810=ORIENTED_EDGE ( 'NONE', *, *, #10060, .F. ) ;
#7813=ORIENTED_EDGE ( 'NONE', *, *, #20861, .F. ) ;
#7814=CARTESIAN_POINT ( 'NONE',  ( 157.4999999999997158, 258.8720626163585621, 45.00000000000000000 ) ) ;
#7815=LINE ( 'NONE', #11857, #8285 ) ;
#7816=DIRECTION ( 'NONE',  ( 0.8916010070295207202, -0.4528218681379515553, 0.000000000000000000 ) ) ;
#7817=EDGE_LOOP ( 'NONE', ( #24741, #22368, #6778, #19856 ) ) ;
#7818=CARTESIAN_POINT ( 'NONE',  ( 157.4999999999998579, 58.24206201579573872, 45.00000000000000000 ) ) ;
#7821=CARTESIAN_POINT ( 'NONE',  ( 158.0000000000016200, 50.97237449702815582, 45.00000000000000000 ) ) ;
#7822=CARTESIAN_POINT ( 'NONE',  ( 158.0000000000011084, 100.6219996396619791, 45.00000000000000000 ) ) ;
#7823=ORIENTED_EDGE ( 'NONE', *, *, #26911, .F. ) ;
#7826=VERTEX_POINT ( 'NONE', #1158 ) ;
#7829=EDGE_LOOP ( 'NONE', ( #725, #6868, #1133, #9342 ) ) ;
#7831=ADVANCED_FACE ( 'NONE', ( #9928 ), #8049, .F. ) ;
#7839=CARTESIAN_POINT ( 'NONE',  ( 187.4999999999996305, 258.6181251126050711, -5.999999999999991118 ) ) ;
#7841=ORIENTED_EDGE ( 'NONE', *, *, #18050, .F. ) ;
#7848=ORIENTED_EDGE ( 'NONE', *, *, #8026, .F. ) ;
#7850=DIRECTION ( 'NONE',  ( 0.8916010070299166257, -0.4528218681371722343, 0.000000000000000000 ) ) ;
#7851=VERTEX_POINT ( 'NONE', #22724 ) ;
#7853=CARTESIAN_POINT ( 'NONE',  ( 158.0000000000015064, 63.00387452705633251, 45.00000000000000000 ) ) ;
#7855=EDGE_LOOP ( 'NONE', ( #26394, #805, #6314, #2503 ) ) ;
#7856=ORIENTED_EDGE ( 'NONE', *, *, #3174, .T. ) ;
#7857=EDGE_CURVE ( 'NONE', #26178, #18505, #16402, .T. ) ;
#7858=EDGE_LOOP ( 'NONE', ( #10513, #3648, #19934, #14293 ) ) ;
#7862=EDGE_CURVE ( 'NONE', #21781, #18321, #14385, .T. ) ;
#7863=EDGE_CURVE ( 'NONE', #4812, #13811, #27569, .T. ) ;
#7867=VECTOR ( 'NONE', #3356, 1000.000000000000000 ) ;
#7868=VECTOR ( 'NONE', #18383, 1000.000000000000000 ) ;
#7875=CARTESIAN_POINT ( 'NONE',  ( 157.4999999999998579, 120.9389372034718093, -45.00000000000000000 ) ) ;
#7877=EDGE_LOOP ( 'NONE', ( #15489, #19868, #5804, #26646 ) ) ;
#7880=VERTEX_POINT ( 'NONE', #12939 ) ;
#7881=ORIENTED_EDGE ( 'NONE', *, *, #4508, .F. ) ;
#7882=VECTOR ( 'NONE', #497, 1000.000000000000000 ) ;
#7886=VECTOR ( 'NONE', #17280, 1000.000000000000000 ) ;
#7888=VERTEX_POINT ( 'NONE', #14953 ) ;
#7889=VECTOR ( 'NONE', #16170, 1000.000000000000000 ) ;
#7890=EDGE_CURVE ( 'NONE', #14086, #25161, #23850, .T. ) ;
#7891=EDGE_LOOP ( 'NONE', ( #15139, #21139, #3458, #20246 ) ) ;
#7892=ORIENTED_EDGE ( 'NONE', *, *, #5237, .F. ) ;
#7894=CARTESIAN_POINT ( 'NONE',  ( 158.0000000000009095, 120.6849996997183183, 45.00000000000000000 ) ) ;
#7895=EDGE_CURVE ( 'NONE', #21239, #14664, #4304, .T. ) ;
#7896=LINE ( 'NONE', #3434, #23377 ) ;
#7901=AXIS2_PLACEMENT_3D ( 'NONE', #3008, #11800, #20539 ) ;
#7910=VERTEX_POINT ( 'NONE', #28139 ) ;
#7912=DIRECTION ( 'NONE',  ( 0.4528218681378716193, 0.8916010070295614653, -0.000000000000000000 ) ) ;
#7913=ORIENTED_EDGE ( 'NONE', *, *, #11624, .F. ) ;
#7916=AXIS2_PLACEMENT_3D ( 'NONE', #23515, #14762, #1953 ) ;
#7920=DIRECTION ( 'NONE',  ( 0.8916010070295719014, -0.4528218681378510246, 0.000000000000000000 ) ) ;
#7922=VERTEX_POINT ( 'NONE', #23563 ) ;
#7923=VECTOR ( 'NONE', #949, 1000.000000000000000 ) ;
#7925=CARTESIAN_POINT ( 'NONE',  ( 158.0000000000008811, 123.1928747072253572, 45.00000000000000000 ) ) ;
#7927=CARTESIAN_POINT ( 'NONE',  ( 158.0000000000013642, 76.05112457209858690, 45.00000000000000000 ) ) ;
#7928=LINE ( 'NONE', #20576, #8679 ) ;
#7929=ORIENTED_EDGE ( 'NONE', *, *, #25411, .T. ) ;
#7932=LINE ( 'NONE', #3609, #18954 ) ;
#7934=EDGE_CURVE ( 'NONE', #14606, #25368, #28278, .T. ) ;
#7942=ORIENTED_EDGE ( 'NONE', *, *, #25986, .F. ) ;
#7945=LINE ( 'NONE', #24811, #12440 ) ;
#7946=CARTESIAN_POINT ( 'NONE',  ( 158.0000000000002558, 181.3818748873943889, 45.00000000000000000 ) ) ;
#7949=ORIENTED_EDGE ( 'NONE', *, *, #9815, .T. ) ;
#7953=EDGE_CURVE ( 'NONE', #21404, #23339, #14662, .T. ) ;
#7954=CARTESIAN_POINT ( 'NONE',  ( 157.4999999999997158, 263.8878126313725829, 45.00000000000000000 ) ) ;
#7956=CARTESIAN_POINT ( 'NONE',  ( 158.0000000000009379, 116.1771246922112653, -45.00000000000000000 ) ) ;
#7957=ORIENTED_EDGE ( 'NONE', *, *, #24681, .F. ) ;
#7961=PLANE ( 'NONE',  #4205 ) ;
#7963=EDGE_LOOP ( 'NONE', ( #20925, #2692, #24248, #13344 ) ) ;
#7966=CARTESIAN_POINT ( 'NONE',  ( 158.0000000000008811, 121.1928747072253572, 45.00000000000000000 ) ) ;
#7970=ORIENTED_EDGE ( 'NONE', *, *, #18816, .F. ) ;
#7972=DIRECTION ( 'NONE',  ( -0.8916010070293995948, -0.4528218681381900867, 0.000000000000000000 ) ) ;
#7975=CARTESIAN_POINT ( 'NONE',  ( 158.0000000000009095, 118.6849996997183041, 45.00000000000000000 ) ) ;
#7976=CARTESIAN_POINT ( 'NONE',  ( 158.0000000000009663, 113.1613746771971876, 45.00000000000000000 ) ) ;
#7977=DIRECTION ( 'NONE',  ( -0.8916010070293584056, -0.4528218681382712996, 0.000000000000000000 ) ) ;
#7981=FACE_OUTER_BOUND ( 'NONE', #5078, .T. ) ;
#7982=CARTESIAN_POINT ( 'NONE',  ( 158.0000000000015348, 58.49599951954928656, -45.00000000000000000 ) ) ;
#7984=ORIENTED_EDGE ( 'NONE', *, *, #23138, .F. ) ;
#7991=LINE ( 'NONE', #27795, #26685 ) ;
#7995=EDGE_CURVE ( 'NONE', #9638, #17008, #6312, .T. ) ;
#7997=ORIENTED_EDGE ( 'NONE', *, *, #8866, .F. ) ;
#7998=DIRECTION ( 'NONE',  ( 0.8916010070293383105, -0.4528218681383106015, 0.000000000000000000 ) ) ;
#7999=ORIENTED_EDGE ( 'NONE', *, *, #16495, .T. ) ;
#8001=ORIENTED_EDGE ( 'NONE', *, *, #9034, .F. ) ;
#8007=VECTOR ( 'NONE', #9818, 1000.000000000000000 ) ;
#8008=CARTESIAN_POINT ( 'NONE',  ( 157.4999999999998579, 53.22631200078164682, -45.00000000000000000 ) ) ;
#8010=FACE_OUTER_BOUND ( 'NONE', #21443, .T. ) ;
#8017=CARTESIAN_POINT ( 'NONE',  ( 157.9999999999996589, 274.1732501651540588, 45.00000000000000000 ) ) ;
#8023=ORIENTED_EDGE ( 'NONE', *, *, #8866, .T. ) ;
#8024=ORIENTED_EDGE ( 'NONE', *, *, #14271, .T. ) ;
#8026=EDGE_CURVE ( 'NONE', #8626, #7922, #10633, .T. ) ;
#8027=DIRECTION ( 'NONE',  ( -0.000000000000000000, 0.000000000000000000, -1.000000000000000000 ) ) ;
#8033=ORIENTED_EDGE ( 'NONE', *, *, #15633, .T. ) ;
#8035=VERTEX_POINT ( 'NONE', #574 ) ;
#8038=VECTOR ( 'NONE', #20622, 1000.000000000000000 ) ;
#8039=AXIS2_PLACEMENT_3D ( 'NONE', #22361, #2668, #17472 ) ;
#8048=FACE_OUTER_BOUND ( 'NONE', #8316, .T. ) ;
#8049=PLANE ( 'NONE',  #11072 ) ;
#8053=EDGE_CURVE ( 'NONE', #23149, #23826, #5012, .T. ) ;
#8055=FACE_OUTER_BOUND ( 'NONE', #7397, .T. ) ;
#8060=ORIENTED_EDGE ( 'NONE', *, *, #41, .T. ) ;
#8062=VECTOR ( 'NONE', #5202, 1000.000000000000000 ) ;
#8063=VERTEX_POINT ( 'NONE', #7034 ) ;
#8064=CARTESIAN_POINT ( 'NONE',  ( 157.9999999999996589, 278.6811251726610976, -45.00000000000000000 ) ) ;
#8069=CARTESIAN_POINT ( 'NONE',  ( 158.0000000000000568, 201.4448749474510407, 45.00000000000000000 ) ) ;
#8070=CARTESIAN_POINT ( 'NONE',  ( 158.0000000000002274, 185.8897498949014278, 45.00000000000000000 ) ) ;
#8072=ORIENTED_EDGE ( 'NONE', *, *, #27412, .T. ) ;
#8080=AXIS2_PLACEMENT_3D ( 'NONE', #12954, #6618, #19552 ) ;
#8083=EDGE_CURVE ( 'NONE', #2726, #23391, #15665, .T. ) ;
#8085=DIRECTION ( 'NONE',  ( -0.8916010070299064116, 0.4528218681371922183, 0.000000000000000000 ) ) ;
#8088=CARTESIAN_POINT ( 'NONE',  ( 158.0000000000015632, 55.98812451204224061, 45.00000000000000000 ) ) ;
#8089=CARTESIAN_POINT ( 'NONE',  ( 157.9999999999998010, 241.0630000600560550, 45.00000000000000000 ) ) ;
#8091=ORIENTED_EDGE ( 'NONE', *, *, #22289, .F. ) ;
#8094=ADVANCED_FACE ( 'NONE', ( #13226 ), #18100, .F. ) ;
#8098=ORIENTED_EDGE ( 'NONE', *, *, #14481, .T. ) ;
#8100=CARTESIAN_POINT ( 'NONE',  ( 157.9999999999996589, 276.1732501651540588, 45.00000000000000000 ) ) ;
#8102=EDGE_CURVE ( 'NONE', #20337, #11428, #6886, .T. ) ;
#8103=CARTESIAN_POINT ( 'NONE',  ( 158.0000000000005400, 153.7952498048169048, 45.00000000000000000 ) ) ;
#8108=DIRECTION ( 'NONE',  ( -0.000000000000000000, -0.000000000000000000, -1.000000000000000000 ) ) ;
#8110=AXIS2_PLACEMENT_3D ( 'NONE', #18164, #26918, #7243 ) ;
#8112=ORIENTED_EDGE ( 'NONE', *, *, #3562, .F. ) ;
#8113=EDGE_CURVE ( 'NONE', #14425, #26178, #13803, .T. ) ;
#8114=LINE ( 'NONE', #23759, #3336 ) ;
#8124=CARTESIAN_POINT ( 'NONE',  ( 157.4999999999998010, 238.8090625563025071, -45.00000000000000000 ) ) ;
#8125=VECTOR ( 'NONE', #20711, 1000.000000000000000 ) ;
#8128=VECTOR ( 'NONE', #11911, 1000.000000000000000 ) ;
#8131=LINE ( 'NONE', #16480, #19243 ) ;
#8133=ORIENTED_EDGE ( 'NONE', *, *, #12522, .T. ) ;
#8135=CARTESIAN_POINT ( 'NONE',  ( 157.4999999999998579, 135.9861872485140850, 45.00000000000000000 ) ) ;
#8136=ORIENTED_EDGE ( 'NONE', *, *, #3391, .T. ) ;
#8137=PLANE ( 'NONE',  #19976 ) ;
#8138=VERTEX_POINT ( 'NONE', #22549 ) ;
#8139=ORIENTED_EDGE ( 'NONE', *, *, #14492, .T. ) ;
#8149=EDGE_CURVE ( 'NONE', #15078, #10864, #8907, .T. ) ;
#8150=LINE ( 'NONE', #8294, #7362 ) ;
#8156=EDGE_CURVE ( 'NONE', #14497, #9601, #4580, .T. ) ;
#8158=DIRECTION ( 'NONE',  ( -0.8916010070293383105, -0.4528218681383106015, 0.000000000000000000 ) ) ;
#8159=LINE ( 'NONE', #3695, #12070 ) ;
#8162=CARTESIAN_POINT ( 'NONE',  ( 157.9999999999996589, 271.6653751576470768, 45.00000000000000000 ) ) ;
#8164=PLANE ( 'NONE',  #22562 ) ;
#8166=VERTEX_POINT ( 'NONE', #432 ) ;
#8171=AXIS2_PLACEMENT_3D ( 'NONE', #22672, #15930, #18496 ) ;
#8172=ORIENTED_EDGE ( 'NONE', *, *, #17061, .T. ) ;
#8173=VERTEX_POINT ( 'NONE', #9194 ) ;
#8179=EDGE_CURVE ( 'NONE', #6129, #4617, #8761, .T. ) ;
#8184=CARTESIAN_POINT ( 'NONE',  ( 158.0000000000006537, 143.7637497747887210, 45.00000000000000000 ) ) ;
#8190=CARTESIAN_POINT ( 'NONE',  ( 158.0000000000002558, 183.3818748873943889, 45.00000000000000000 ) ) ;
#8198=ORIENTED_EDGE ( 'NONE', *, *, #11660, .F. ) ;
#8200=ORIENTED_EDGE ( 'NONE', *, *, #13975, .F. ) ;
#8205=CARTESIAN_POINT ( 'NONE',  ( 158.0000000000011369, 96.11412463215494029, 45.00000000000000000 ) ) ;
#8208=CARTESIAN_POINT ( 'NONE',  ( 158.0000000000001137, 195.9212499249295831, 45.00000000000000000 ) ) ;
#8213=EDGE_CURVE ( 'NONE', #14958, #1247, #9622, .T. ) ;
#8215=ORIENTED_EDGE ( 'NONE', *, *, #22893, .T. ) ;
#8217=EDGE_CURVE ( 'NONE', #19122, #18428, #12349, .T. ) ;
#8222=AXIS2_PLACEMENT_3D ( 'NONE', #19599, #28339, #2341 ) ;
#8224=DIRECTION ( 'NONE',  ( 0.8916010070293584056, -0.4528218681382712996, 0.000000000000000000 ) ) ;
#8225=CARTESIAN_POINT ( 'NONE',  ( 158.0000000000000000, 206.4606249624626457, 45.00000000000000000 ) ) ;
#8229=DIRECTION ( 'NONE',  ( 0.4528218681375913990, 0.8916010070297037959, -0.000000000000000000 ) ) ;
#8233=AXIS2_PLACEMENT_3D ( 'NONE', #18135, #5192, #11685 ) ;
#8234=DIRECTION ( 'NONE',  ( -0.8916010070299774659, 0.4528218681370523302, 0.000000000000000000 ) ) ;
#8237=EDGE_LOOP ( 'NONE', ( #12851, #26995, #14752, #17668 ) ) ;
#8239=DIRECTION ( 'NONE',  ( -0.000000000000000000, -0.000000000000000000, -1.000000000000000000 ) ) ;
#8241=VECTOR ( 'NONE', #10714, 1000.000000000000000 ) ;
#8243=CARTESIAN_POINT ( 'NONE',  ( 158.0000000000001421, 191.4133749174225443, -45.00000000000000000 ) ) ;
#8245=VERTEX_POINT ( 'NONE', #9486 ) ;
#8246=VECTOR ( 'NONE', #20796, 1000.000000000000000 ) ;
#8254=DIRECTION ( 'NONE',  ( 0.8916010070293483025, 0.4528218681382912836, 0.000000000000000000 ) ) ;
#8257=DIRECTION ( 'NONE',  ( -0.8916010070293995948, -0.4528218681381900867, 0.000000000000000000 ) ) ;
#8258=FACE_BOUND ( 'NONE', #1888, .T. ) ;
#8262=AXIS2_PLACEMENT_3D ( 'NONE', #5933, #14707, #19012 ) ;
#8267=CARTESIAN_POINT ( 'NONE',  ( 157.9999999999998863, 216.4921249924925348, -45.00000000000000000 ) ) ;
#8268=DIRECTION ( 'NONE',  ( 0.8916010070300282031, -0.4528218681369524101, 0.000000000000000000 ) ) ;
#8269=CARTESIAN_POINT ( 'NONE',  ( 158.0000000000015632, 55.98812451204224061, -45.00000000000000000 ) ) ;
#8277=EDGE_LOOP ( 'NONE', ( #13489, #25903, #7984, #19157 ) ) ;
#8278=VECTOR ( 'NONE', #244, 1000.000000000000000 ) ;
#8283=ORIENTED_EDGE ( 'NONE', *, *, #5170, .F. ) ;
#8285=VECTOR ( 'NONE', #12143, 1000.000000000000000 ) ;
#8287=EDGE_CURVE ( 'NONE', #10360, #1132, #10606, .T. ) ;
#8288=EDGE_LOOP ( 'NONE', ( #20502, #9131, #27835, #4165 ) ) ;
#8293=DIRECTION ( 'NONE',  ( 0.4528218681375319465, 0.8916010070297339940, -0.000000000000000000 ) ) ;
#8294=CARTESIAN_POINT ( 'NONE',  ( 157.4999999999998579, 95.86018712840139244, 45.00000000000000000 ) ) ;
#8302=CARTESIAN_POINT ( 'NONE',  ( 157.9999999999997726, 248.5866250825770294, 45.00000000000000000 ) ) ;
#8303=CARTESIAN_POINT ( 'NONE',  ( 157.9999999999998295, 228.5236250225210313, 45.00000000000000000 ) ) ;
#8306=EDGE_LOOP ( 'NONE', ( #22262, #26864, #5596, #1757 ) ) ;
#8310=CARTESIAN_POINT ( 'NONE',  ( 157.4999999999998579, 88.33656210588026170, 45.00000000000000000 ) ) ;
#8312=ORIENTED_EDGE ( 'NONE', *, *, #8607, .F. ) ;
#8313=ADVANCED_FACE ( 'NONE', ( #6285 ), #8164, .F. ) ;
#8314=EDGE_CURVE ( 'NONE', #15041, #3632, #25541, .T. ) ;
#8316=EDGE_LOOP ( 'NONE', ( #6830, #10093, #5450, #1703 ) ) ;
#8321=VERTEX_POINT ( 'NONE', #17064 ) ;
#8322=ORIENTED_EDGE ( 'NONE', *, *, #12419, .T. ) ;
#8323=CARTESIAN_POINT ( 'NONE',  ( 158.0000000000000000, 206.4606249624626457, -45.00000000000000000 ) ) ;
#8324=VECTOR ( 'NONE', #2892, 1000.000000000000000 ) ;
#8326=CARTESIAN_POINT ( 'NONE',  ( 157.4999999999998579, 146.0176872785422404, 45.00000000000000000 ) ) ;
#8329=CARTESIAN_POINT ( 'NONE',  ( 157.4999999999998579, 103.3838121509225090, 45.00000000000000000 ) ) ;
#8330=DIRECTION ( 'NONE',  ( 0.4528218681373120669, 0.8916010070298455714, -0.000000000000000000 ) ) ;
#8331=PLANE ( 'NONE',  #10226 ) ;
#8332=VECTOR ( 'NONE', #6947, 1000.000000000000114 ) ;
#8333=DIRECTION ( 'NONE',  ( -0.000000000000000000, -0.000000000000000000, -1.000000000000000000 ) ) ;
#8338=ORIENTED_EDGE ( 'NONE', *, *, #5359, .T. ) ;
#8339=AXIS2_PLACEMENT_3D ( 'NONE', #20888, #21305, #3497 ) ;
#8343=ORIENTED_EDGE ( 'NONE', *, *, #7217, .F. ) ;
#8350=PLANE ( 'NONE',  #6256 ) ;
#8352=EDGE_CURVE ( 'NONE', #26072, #4314, #10182, .T. ) ;
#8355=VECTOR ( 'NONE', #28172, 1000.000000000000000 ) ;
#8359=LINE ( 'NONE', #3471, #3180 ) ;
#8362=CARTESIAN_POINT ( 'NONE',  ( 158.0000000000009095, 120.6849996997183183, -45.00000000000000000 ) ) ;
#8364=CARTESIAN_POINT ( 'NONE',  ( 158.0000000000004547, 163.8267498348450886, -45.00000000000000000 ) ) ;
#8365=CARTESIAN_POINT ( 'NONE',  ( 158.0000000000006821, 138.7479997597746433, 45.00000000000000000 ) ) ;
#8366=DIRECTION ( 'NONE',  ( -0.8916010070293783896, 0.4528218681382319422, 0.000000000000000000 ) ) ;
#8369=PLANE ( 'NONE',  #13820 ) ;
#8370=DIRECTION ( 'NONE',  ( -0.000000000000000000, 0.000000000000000000, -1.000000000000000000 ) ) ;
#8374=FACE_OUTER_BOUND ( 'NONE', #25440, .T. ) ;
#8375=AXIS2_PLACEMENT_3D ( 'NONE', #19392, #19539, #4156 ) ;
#8377=DIRECTION ( 'NONE',  ( 1.000000000000000000, 0.000000000000000000, -0.000000000000000000 ) ) ;
#8381=PLANE ( 'NONE',  #20763 ) ;
#8383=VECTOR ( 'NONE', #21086, 1000.000000000000000 ) ;
#8392=ORIENTED_EDGE ( 'NONE', *, *, #13947, .T. ) ;
#8394=ORIENTED_EDGE ( 'NONE', *, *, #17771, .T. ) ;
#8398=CARTESIAN_POINT ( 'NONE',  ( 158.0000000000013074, 83.06687458711267880, 45.00000000000000000 ) ) ;
#8401=PLANE ( 'NONE',  #4753 ) ;
#8402=VECTOR ( 'NONE', #16069, 1000.000000000000000 ) ;
#8403=CARTESIAN_POINT ( 'NONE',  ( 158.0000000000010800, 103.1298746471690038, 45.00000000000000000 ) ) ;
#8410=DIRECTION ( 'NONE',  ( -0.8916010070293283185, -0.4528218681383305855, 0.000000000000000000 ) ) ;
#8418=DIRECTION ( 'NONE',  ( 0.000000000000000000, -1.000000000000000000, 0.000000000000000000 ) ) ;
#8420=ORIENTED_EDGE ( 'NONE', *, *, #25002, .T. ) ;
#8421=VECTOR ( 'NONE', #4890, 999.9999999999998863 ) ;
#8425=ORIENTED_EDGE ( 'NONE', *, *, #18796, .T. ) ;
#8428=ORIENTED_EDGE ( 'NONE', *, *, #19113, .F. ) ;
#8430=EDGE_LOOP ( 'NONE', ( #20900, #5407, #20480, #21730 ) ) ;
#8431=DIRECTION ( 'NONE',  ( -0.000000000000000000, -0.000000000000000000, -1.000000000000000000 ) ) ;
#8432=PRODUCT_DEFINITION ( 'UNKNOWN', '', #22578, #20085 ) ;
#8447=CARTESIAN_POINT ( 'NONE',  ( 158.0000000000015348, 60.49599951954928656, 45.00000000000000000 ) ) ;
#8449=CARTESIAN_POINT ( 'NONE',  ( 158.0000000000003411, 173.8582498648732440, 45.00000000000000000 ) ) ;
#8453=CARTESIAN_POINT ( 'NONE',  ( 158.0000000000010516, 105.6377496546760568, -45.00000000000000000 ) ) ;
#8455=ORIENTED_EDGE ( 'NONE', *, *, #9227, .T. ) ;
#8459=ADVANCED_FACE ( 'NONE', ( #22227 ), #2535, .F. ) ;
#8460=ORIENTED_EDGE ( 'NONE', *, *, #12806, .T. ) ;
#8461=ORIENTED_EDGE ( 'NONE', *, *, #25620, .T. ) ;
#8462=ADVANCED_FACE ( 'NONE', ( #15493 ), #542, .F. ) ;
#8465=ORIENTED_EDGE ( 'NONE', *, *, #12847, .F. ) ;
#8471=FACE_OUTER_BOUND ( 'NONE', #26463, .T. ) ;
#8472=CARTESIAN_POINT ( 'NONE',  ( 158.0000000000011653, 95.60624962464788723, 45.00000000000000000 ) ) ;
#8478=CARTESIAN_POINT ( 'NONE',  ( 157.4999999999998010, 233.7933125412885147, -45.00000000000000000 ) ) ;
#8480=PLANE ( 'NONE',  #24434 ) ;
#8486=VERTEX_POINT ( 'NONE', #12178 ) ;
#8487=ORIENTED_EDGE ( 'NONE', *, *, #17597, .T. ) ;
#8488=EDGE_CURVE ( 'NONE', #19893, #7880, #20499, .T. ) ;
#8494=VECTOR ( 'NONE', #25955, 1000.000000000000000 ) ;
#8496=ORIENTED_EDGE ( 'NONE', *, *, #24657, .F. ) ;
#8499=DIRECTION ( 'NONE',  ( 0.8916010070295820045, 0.4528218681378310406, 0.000000000000000000 ) ) ;
#8505=EDGE_CURVE ( 'NONE', #12774, #7618, #3244, .T. ) ;
#8508=ADVANCED_FACE ( 'NONE', ( #22519 ), #22804, .F. ) ;
#8517=DIRECTION ( 'NONE',  ( 0.000000000000000000, -1.000000000000000000, 0.000000000000000000 ) ) ;
#8521=LINE ( 'NONE', #10816, #22470 ) ;
#8524=DIRECTION ( 'NONE',  ( -0.000000000000000000, 0.000000000000000000, -1.000000000000000000 ) ) ;
#8526=DIRECTION ( 'NONE',  ( 0.8916010070299369428, -0.4528218681371322663, 0.000000000000000000 ) ) ;
#8529=CARTESIAN_POINT ( 'NONE',  ( 158.0000000000012790, 83.57474959461971764, 45.00000000000000000 ) ) ;
#8535=ORIENTED_EDGE ( 'NONE', *, *, #25176, .T. ) ;
#8537=VERTEX_POINT ( 'NONE', #26962 ) ;
#8539=VECTOR ( 'NONE', #5941, 1000.000000000000000 ) ;
#8540=CARTESIAN_POINT ( 'NONE',  ( 158.0000000000015632, 57.98812451204224061, -45.00000000000000000 ) ) ;
#8542=CARTESIAN_POINT ( 'NONE',  ( 157.9999999999996874, 271.1575001501400379, -45.00000000000000000 ) ) ;
#8548=CARTESIAN_POINT ( 'NONE',  ( 157.9999999999997442, 251.0945000900840398, -45.00000000000000000 ) ) ;
#8551=APPLICATION_CONTEXT ( 'automotive_design' ) ;
#8553=FACE_OUTER_BOUND ( 'NONE', #26639, .T. ) ;
#8556=VERTEX_POINT ( 'NONE', #5406 ) ;
#8560=DIRECTION ( 'NONE',  ( 0.4528218681374507892, -0.8916010070297751833, 0.000000000000000000 ) ) ;
#8561=DIRECTION ( 'NONE',  ( -0.8916010070298360235, -0.4528218681373308852, 0.000000000000000000 ) ) ;
#8563=VECTOR ( 'NONE', #21352, 1000.000000000000000 ) ;
#8565=VERTEX_POINT ( 'NONE', #14186 ) ;
#8569=ORIENTED_EDGE ( 'NONE', *, *, #23557, .T. ) ;
#8574=CARTESIAN_POINT ( 'NONE',  ( 158.0000000000004263, 168.3346248423521274, 45.00000000000000000 ) ) ;
#8576=PLANE ( 'NONE',  #5177 ) ;
#8581=ADVANCED_FACE ( 'NONE', ( #18767 ), #24817, .F. ) ;
#8588=DIRECTION ( 'NONE',  ( -0.000000000000000000, 0.000000000000000000, -1.000000000000000000 ) ) ;
#8589=CARTESIAN_POINT ( 'NONE',  ( 157.9999999999996589, 276.6811251726610976, -45.00000000000000000 ) ) ;
#8590=DIRECTION ( 'NONE',  ( 0.8916010070297338830, -0.4528218681375318910, 0.000000000000000000 ) ) ;
#8594=CARTESIAN_POINT ( 'NONE',  ( 157.4999999999998579, 148.5255622860493077, -45.00000000000000000 ) ) ;
#8595=DIRECTION ( 'NONE',  ( 0.8916010070294706491, 0.4528218681380502542, 0.000000000000000000 ) ) ;
#8596=ORIENTED_EDGE ( 'NONE', *, *, #24179, .F. ) ;
#8598=ORIENTED_EDGE ( 'NONE', *, *, #15070, .F. ) ;
#8602=ORIENTED_EDGE ( 'NONE', *, *, #24281, .F. ) ;
#8604=ORIENTED_EDGE ( 'NONE', *, *, #26964, .F. ) ;
#8605=ORIENTED_EDGE ( 'NONE', *, *, #13093, .T. ) ;
#8607=EDGE_CURVE ( 'NONE', #20671, #16796, #19184, .T. ) ;
#8610=DIRECTION ( 'NONE',  ( 0.000000000000000000, -1.000000000000000000, 0.000000000000000000 ) ) ;
#8614=EDGE_CURVE ( 'NONE', #27410, #729, #21624, .T. ) ;
#8615=CARTESIAN_POINT ( 'NONE',  ( 158.0000000000011369, 98.11412463215494029, -45.00000000000000000 ) ) ;
#8616=LINE ( 'NONE', #11055, #12163 ) ;
#8617=LINE ( 'NONE', #17368, #375 ) ;
#8618=AXIS2_PLACEMENT_3D ( 'NONE', #10024, #9605, #3257 ) ;
#8622=CARTESIAN_POINT ( 'NONE',  ( 158.0000000000001421, 191.4133749174225443, 45.00000000000000000 ) ) ;
#8624=CARTESIAN_POINT ( 'NONE',  ( 157.9999999999996589, 278.6811251726610976, -45.00000000000000000 ) ) ;
#8626=VERTEX_POINT ( 'NONE', #19328 ) ;
#8629=VERTEX_POINT ( 'NONE', #12879 ) ;
#8633=VECTOR ( 'NONE', #8158, 1000.000000000000114 ) ;
#8637=VECTOR ( 'NONE', #18306, 1000.000000000000114 ) ;
#8640=EDGE_CURVE ( 'NONE', #21329, #24666, #18905, .T. ) ;
#8645=LINE ( 'NONE', #26580, #5211 ) ;
#8653=DIRECTION ( 'NONE',  ( 0.4528218681382713551, -0.8916010070293584056, 0.000000000000000000 ) ) ;
#8657=CARTESIAN_POINT ( 'NONE',  ( 157.4999999999998579, 178.6200623761337738, 45.00000000000000000 ) ) ;
#8673=CARTESIAN_POINT ( 'NONE',  ( 158.0000000000013642, 78.05112457209858690, 45.00000000000000000 ) ) ;
#8674=AXIS2_PLACEMENT_3D ( 'NONE', #3868, #8330, #1155 ) ;
#8679=VECTOR ( 'NONE', #25037, 1000.000000000000000 ) ;
#8683=FACE_OUTER_BOUND ( 'NONE', #24848, .T. ) ;
#8686=AXIS2_PLACEMENT_3D ( 'NONE', #8693, #20026, #24202 ) ;
#8687=CARTESIAN_POINT ( 'NONE',  ( 158.0000000000003979, 170.8424998498591663, 45.00000000000000000 ) ) ;
#8689=CARTESIAN_POINT ( 'NONE',  ( 158.0000000000002274, 185.8897498949014278, -45.00000000000000000 ) ) ;
#8690=CARTESIAN_POINT ( 'NONE',  ( 158.0000000000001137, 195.9212499249295831, -45.00000000000000000 ) ) ;
#8691=DIRECTION ( 'NONE',  ( -0.8916010070293383105, -0.4528218681383106015, 0.000000000000000000 ) ) ;
#8693=CARTESIAN_POINT ( 'NONE',  ( 158.0000000000013358, 78.55899957960562574, 45.00000000000000000 ) ) ;
#8695=LINE ( 'NONE', #22191, #21703 ) ;
#8697=DIRECTION ( 'NONE',  ( 0.8916010070296834789, 0.4528218681376311450, 0.000000000000000000 ) ) ;
#8700=ORIENTED_EDGE ( 'NONE', *, *, #11905, .T. ) ;
#8703=PLANE ( 'NONE',  #2088 ) ;
#8705=VERTEX_POINT ( 'NONE', #10572 ) ;
#8706=EDGE_CURVE ( 'NONE', #11442, #15969, #28219, .T. ) ;
#8707=LINE ( 'NONE', #13175, #3481 ) ;
#8710=ORIENTED_EDGE ( 'NONE', *, *, #4178, .F. ) ;
#8712=FACE_OUTER_BOUND ( 'NONE', #20959, .T. ) ;
#8713=CARTESIAN_POINT ( 'NONE',  ( 158.0000000000011369, 96.11412463215494029, 45.00000000000000000 ) ) ;
#8719=PLANE ( 'NONE',  #8039 ) ;
#8722=CARTESIAN_POINT ( 'NONE',  ( 157.4999999999998579, 130.9704372334999789, 45.00000000000000000 ) ) ;
#8723=FACE_OUTER_BOUND ( 'NONE', #18667, .T. ) ;
#8725=LINE ( 'NONE', #6426, #17131 ) ;
#8728=AXIS2_PLACEMENT_3D ( 'NONE', #14309, #17331, #12759 ) ;
#8729=EDGE_CURVE ( 'NONE', #26896, #11940, #6254, .T. ) ;
#8731=CARTESIAN_POINT ( 'NONE',  ( 157.4999999999998579, 55.73418700828869277, 45.00000000000000000 ) ) ;
#8732=CARTESIAN_POINT ( 'NONE',  ( 157.4999999999998579, 73.28931206083800021, 45.00000000000000000 ) ) ;
#8738=ORIENTED_EDGE ( 'NONE', *, *, #21569, .T. ) ;
#8739=EDGE_CURVE ( 'NONE', #7910, #5416, #1384, .T. ) ;
#8741=EDGE_CURVE ( 'NONE', #5416, #152, #7991, .T. ) ;
#8744=ORIENTED_EDGE ( 'NONE', *, *, #4227, .T. ) ;
#8745=ORIENTED_EDGE ( 'NONE', *, *, #16955, .T. ) ;
#8747=PLANE ( 'NONE',  #2164 ) ;
#8750=CARTESIAN_POINT ( 'NONE',  ( 157.9999999999997158, 261.1260001201120531, -45.00000000000000000 ) ) ;
#8756=DIRECTION ( 'NONE',  ( -0.000000000000000000, -0.000000000000000000, -1.000000000000000000 ) ) ;
#8761=LINE ( 'NONE', #13656, #17962 ) ;
#8762=DIRECTION ( 'NONE',  ( -0.8916010070290389944, 0.4528218681389001299, 0.000000000000000000 ) ) ;
#8766=EDGE_CURVE ( 'NONE', #2485, #1653, #15601, .T. ) ;
#8767=VECTOR ( 'NONE', #13649, 1000.000000000000000 ) ;
#8771=VERTEX_POINT ( 'NONE', #13165 ) ;
#8772=VECTOR ( 'NONE', #24559, 1000.000000000000114 ) ;
#8775=EDGE_CURVE ( 'NONE', #10126, #18558, #2499, .T. ) ;
#8778=LINE ( 'NONE', #26298, #25204 ) ;
#8786=VECTOR ( 'NONE', #20099, 999.9999999999998863 ) ;
#8787=ORIENTED_EDGE ( 'NONE', *, *, #13546, .F. ) ;
#8788=LINE ( 'NONE', #17265, #6326 ) ;
#8789=DIRECTION ( 'NONE',  ( 0.8916010070293383105, -0.4528218681383106015, 0.000000000000000000 ) ) ;
#8790=PLANE ( 'NONE',  #3772 ) ;
#8791=LINE ( 'NONE', #13691, #4312 ) ;
#8792=EDGE_LOOP ( 'NONE', ( #21299, #20133, #23187, #12749 ) ) ;
#8796=LINE ( 'NONE', #11393, #19517 ) ;
#8797=VERTEX_POINT ( 'NONE', #15320 ) ;
#8798=VERTEX_POINT ( 'NONE', #17594 ) ;
#8801=LINE ( 'NONE', #13553, #12941 ) ;
#8804=VECTOR ( 'NONE', #22595, 1000.000000000000000 ) ;
#8808=DIRECTION ( 'NONE',  ( 0.4528218681380715149, 0.8916010070294598799, -0.000000000000000000 ) ) ;
#8813=DIRECTION ( 'NONE',  ( -0.8916010070299577039, -0.4528218681370910215, 0.000000000000000000 ) ) ;
#8814=PLANE ( 'NONE',  #3854 ) ;
#8815=CARTESIAN_POINT ( 'NONE',  ( 157.4999999999998579, 118.4310621959647563, -45.00000000000000000 ) ) ;
#8816=CARTESIAN_POINT ( 'NONE',  ( 157.9999999999998295, 229.0315000300280417, -45.00000000000000000 ) ) ;
#8817=EDGE_CURVE ( 'NONE', #16274, #23832, #11435, .T. ) ;
#8818=VECTOR ( 'NONE', #14542, 1000.000000000000000 ) ;
#8821=ORIENTED_EDGE ( 'NONE', *, *, #17771, .F. ) ;
#8824=CARTESIAN_POINT ( 'NONE',  ( 157.4999999999998579, 141.0019372635281627, -45.00000000000000000 ) ) ;
#8826=AXIS2_PLACEMENT_3D ( 'NONE', #16467, #22653, #5258 ) ;
#8830=CARTESIAN_POINT ( 'NONE',  ( 158.0000000000015064, 63.00387452705633251, 45.00000000000000000 ) ) ;
#8832=ORIENTED_EDGE ( 'NONE', *, *, #27000, .F. ) ;
#8838=ORIENTED_EDGE ( 'NONE', *, *, #3141, .T. ) ;
#8841=DIRECTION ( 'NONE',  ( 0.000000000000000000, -1.000000000000000000, 0.000000000000000000 ) ) ;
#8842=ORIENTED_EDGE ( 'NONE', *, *, #15827, .T. ) ;
#8846=CARTESIAN_POINT ( 'NONE',  ( 158.0000000000001990, 186.3976249024084666, 45.00000000000000000 ) ) ;
#8853=VECTOR ( 'NONE', #7850, 1000.000000000000227 ) ;
#8857=ADVANCED_FACE ( 'NONE', ( #27070 ), #15460, .F. ) ;
#8858=LINE ( 'NONE', #4260, #8278 ) ;
#8861=DIRECTION ( 'NONE',  ( 1.000000000000000000, 0.000000000000000000, -0.000000000000000000 ) ) ;
#8863=CARTESIAN_POINT ( 'NONE',  ( 157.4999999999997158, 261.3799376238655441, 45.00000000000000000 ) ) ;
#8864=CARTESIAN_POINT ( 'NONE',  ( 157.9999999999997158, 256.6181251126050711, 45.00000000000000000 ) ) ;
#8865=DIRECTION ( 'NONE',  ( 0.8916010070297643031, -0.4528218681374719945, 0.000000000000000000 ) ) ;
#8866=EDGE_CURVE ( 'NONE', #21473, #14934, #16310, .T. ) ;
#8867=ORIENTED_EDGE ( 'NONE', *, *, #23113, .T. ) ;
#8869=DIRECTION ( 'NONE',  ( 0.8916010070299876800, -0.4528218681370323462, 0.000000000000000000 ) ) ;
#8871=VECTOR ( 'NONE', #9555, 1000.000000000000000 ) ;
#8873=DIRECTION ( 'NONE',  ( 0.4528218681370711485, -0.8916010070299680290, 0.000000000000000000 ) ) ;
#8876=VECTOR ( 'NONE', #13910, 1000.000000000000000 ) ;
#8877=ORIENTED_EDGE ( 'NONE', *, *, #24863, .T. ) ;
#8879=ORIENTED_EDGE ( 'NONE', *, *, #19514, .F. ) ;
#8883=VERTEX_POINT ( 'NONE', #18592 ) ;
#8886=CARTESIAN_POINT ( 'NONE',  ( 157.4999999999998579, 168.5885623461056184, -45.00000000000000000 ) ) ;
#8889=VECTOR ( 'NONE', #17711, 1000.000000000000000 ) ;
#8890=CARTESIAN_POINT ( 'NONE',  ( 157.4999999999998579, 105.8916871584295478, -45.00000000000000000 ) ) ;
#8891=VECTOR ( 'NONE', #2072, 1000.000000000000000 ) ;
#8897=LINE ( 'NONE', #26693, #22762 ) ;
#8899=CARTESIAN_POINT ( 'NONE',  ( 157.4999999999998579, 128.4625622259929401, -45.00000000000000000 ) ) ;
#8900=DIRECTION ( 'NONE',  ( 0.8916010070293383105, -0.4528218681383106015, 0.000000000000000000 ) ) ;
#8907=LINE ( 'NONE', #2423, #8786 ) ;
#8911=VECTOR ( 'NONE', #15725, 1000.000000000000000 ) ;
#8914=ORIENTED_EDGE ( 'NONE', *, *, #19674, .F. ) ;
#8915=VECTOR ( 'NONE', #23599, 1000.000000000000000 ) ;
#8920=ORIENTED_EDGE ( 'NONE', *, *, #19214, .F. ) ;
#8924=VERTEX_POINT ( 'NONE', #7546 ) ;
#8927=DIRECTION ( 'NONE',  ( 1.000000000000000000, 0.000000000000000000, -0.000000000000000000 ) ) ;
#8932=ORIENTED_EDGE ( 'NONE', *, *, #23776, .F. ) ;
#8935=CARTESIAN_POINT ( 'NONE',  ( 157.4999999999997442, 251.3484375938375024, -45.00000000000000000 ) ) ;
#8936=DIRECTION ( 'NONE',  ( 0.8916010070293995948, 0.4528218681381900312, 0.000000000000000000 ) ) ;
#8938=ORIENTED_EDGE ( 'NONE', *, *, #27083, .T. ) ;
#8943=( LENGTH_UNIT ( ) NAMED_UNIT ( * ) SI_UNIT ( .MILLI., .METRE. ) );
#8947=DIRECTION ( 'NONE',  ( 0.8916010070294598799, -0.4528218681380714594, 0.000000000000000000 ) ) ;
#8951=EDGE_LOOP ( 'NONE', ( #21174, #4801, #23229, #27831 ) ) ;
#8952=CARTESIAN_POINT ( 'NONE',  ( 157.9999999999997158, 259.1260001201120531, -45.00000000000000000 ) ) ;
#8955=ORIENTED_EDGE ( 'NONE', *, *, #16972, .T. ) ;
#8957=EDGE_CURVE ( 'NONE', #4617, #17073, #27620, .T. ) ;
#8960=LINE ( 'NONE', #17719, #20837 ) ;
#8962=CARTESIAN_POINT ( 'NONE',  ( 157.4999999999998579, 108.3995621659365867, 45.00000000000000000 ) ) ;
#8967=FACE_OUTER_BOUND ( 'NONE', #5097, .T. ) ;
#8968=ADVANCED_FACE ( 'NONE', ( #1759 ), #1626, .F. ) ;
#8969=AXIS2_PLACEMENT_3D ( 'NONE', #10785, #23571, #1860 ) ;
#8970=DIRECTION ( 'NONE',  ( 0.8916010070299064116, -0.4528218681371922183, 0.000000000000000000 ) ) ;
#8972=CARTESIAN_POINT ( 'NONE',  ( 157.9999999999998010, 239.0630000600560550, 45.00000000000000000 ) ) ;
#8975=ORIENTED_EDGE ( 'NONE', *, *, #16527, .F. ) ;
#8981=CARTESIAN_POINT ( 'NONE',  ( 158.0000000000003979, 168.8424998498591663, 45.00000000000000000 ) ) ;
#8983=VERTEX_POINT ( 'NONE', #16585 ) ;
#8986=DIRECTION ( 'NONE',  ( 1.000000000000000000, 0.000000000000000000, -0.000000000000000000 ) ) ;
#8988=AXIS2_PLACEMENT_3D ( 'NONE', #20868, #5639, #1465 ) ;
#8989=AXIS2_PLACEMENT_3D ( 'NONE', #7702, #18201, #11606 ) ;
#8992=EDGE_LOOP ( 'NONE', ( #18499, #4453, #3741, #5104 ) ) ;
#9002=DIRECTION ( 'NONE',  ( 1.000000000000000000, 0.000000000000000000, -0.000000000000000000 ) ) ;
#9008=LINE ( 'NONE', #20492, #22414 ) ;
#9012=PLANE ( 'NONE',  #18834 ) ;
#9022=VERTEX_POINT ( 'NONE', #23325 ) ;
#9024=ORIENTED_EDGE ( 'NONE', *, *, #20567, .F. ) ;
#9026=ORIENTED_EDGE ( 'NONE', *, *, #12017, .T. ) ;
#9027=ORIENTED_EDGE ( 'NONE', *, *, #19877, .F. ) ;
#9030=LINE ( 'NONE', #8886, #2618 ) ;
#9034=EDGE_CURVE ( 'NONE', #4647, #20791, #17141, .T. ) ;
#9036=ADVANCED_FACE ( 'NONE', ( #28036 ), #27896, .F. ) ;
#9037=CARTESIAN_POINT ( 'NONE',  ( 158.0000000000004263, 168.3346248423521274, -45.00000000000000000 ) ) ;
#9041=LINE ( 'NONE', #6597, #10366 ) ;
#9042=DIRECTION ( 'NONE',  ( 0.8916010070298353574, -0.4528218681373320509, 0.000000000000000000 ) ) ;
#9043=LINE ( 'NONE', #10627, #20088 ) ;
#9044=DIRECTION ( 'NONE',  ( 0.000000000000000000, -1.000000000000000000, 0.000000000000000000 ) ) ;
#9050=VERTEX_POINT ( 'NONE', #10397 ) ;
#9053=CARTESIAN_POINT ( 'NONE',  ( 0.000000000000000000, 0.000000000000000000, -45.00000000000000000 ) ) ;
#9057=ORIENTED_EDGE ( 'NONE', *, *, #17061, .F. ) ;
#9060=ORIENTED_EDGE ( 'NONE', *, *, #10081, .T. ) ;
#9061=EDGE_CURVE ( 'NONE', #1176, #12421, #27480, .T. ) ;
#9063=PLANE ( 'NONE',  #4912 ) ;
#9065=CARTESIAN_POINT ( 'NONE',  ( 157.4999999999998010, 233.7933125412885147, -45.00000000000000000 ) ) ;
#9066=VERTEX_POINT ( 'NONE', #14434 ) ;
#9069=DIRECTION ( 'NONE',  ( -0.000000000000000000, -0.000000000000000000, -1.000000000000000000 ) ) ;
#9070=AXIS2_PLACEMENT_3D ( 'NONE', #17466, #21638, #16141 ) ;
#9074=ORIENTED_EDGE ( 'NONE', *, *, #17460, .F. ) ;
#9078=DIRECTION ( 'NONE',  ( -0.8916010070297345491, -0.4528218681375307253, 0.000000000000000000 ) ) ;
#9082=ADVANCED_FACE ( 'NONE', ( #10537 ), #8381, .F. ) ;
#9083=CARTESIAN_POINT ( 'NONE',  ( 157.4999999999998579, 50.71843699327460797, 45.00000000000000000 ) ) ;
#9084=AXIS2_PLACEMENT_3D ( 'NONE', #5079, #22619, #27197 ) ;
#9088=LINE ( 'NONE', #19581, #23492 ) ;
#9090=ORIENTED_EDGE ( 'NONE', *, *, #26653, .T. ) ;
#9092=ORIENTED_EDGE ( 'NONE', *, *, #9758, .T. ) ;
#9094=CARTESIAN_POINT ( 'NONE',  ( 157.9999999999998579, 221.0000000000000284, 45.00000000000000000 ) ) ;
#9095=EDGE_CURVE ( 'NONE', #12922, #16796, #4199, .T. ) ;
#9096=LINE ( 'NONE', #8673, #7526 ) ;
#9098=ADVANCED_FACE ( 'NONE', ( #13808 ), #22556, .F. ) ;
#9099=ORIENTED_EDGE ( 'NONE', *, *, #17499, .T. ) ;
#9103=CARTESIAN_POINT ( 'NONE',  ( 157.4999999999998579, 181.1279373836408411, 45.00000000000000000 ) ) ;
#9104=LINE ( 'NONE', #26614, #21743 ) ;
#9106=LINE ( 'NONE', #17864, #12787 ) ;
#9110=FACE_OUTER_BOUND ( 'NONE', #18733, .T. ) ;
#9111=CARTESIAN_POINT ( 'NONE',  ( 157.9999999999998579, 223.5078750075070104, -45.00000000000000000 ) ) ;
#9112=DIRECTION ( 'NONE',  ( -0.000000000000000000, -0.000000000000000000, -1.000000000000000000 ) ) ;
#9113=CARTESIAN_POINT ( 'NONE',  ( 157.4999999999995737, 203.6988124512014338, 45.00000000000000000 ) ) ;
#9114=VERTEX_POINT ( 'NONE', #6891 ) ;
#9115=DIRECTION ( 'NONE',  ( -0.000000000000000000, 0.000000000000000000, -1.000000000000000000 ) ) ;
#9116=VERTEX_POINT ( 'NONE', #28181 ) ;
#9122=FACE_OUTER_BOUND ( 'NONE', #4666, .T. ) ;
#9125=EDGE_CURVE ( 'NONE', #14251, #11388, #22267, .T. ) ;
#9129=ADVANCED_FACE ( 'NONE', ( #20250 ), #2430, .F. ) ;
#9130=AXIS2_PLACEMENT_3D ( 'NONE', #16566, #23170, #5780 ) ;
#9131=ORIENTED_EDGE ( 'NONE', *, *, #11305, .F. ) ;
#9132=ORIENTED_EDGE ( 'NONE', *, *, #2105, .T. ) ;
#9134=LINE ( 'NONE', #8846, #17714 ) ;
#9140=EDGE_CURVE ( 'NONE', #9424, #21412, #23893, .T. ) ;
#9144=LINE ( 'NONE', #4530, #2749 ) ;
#9146=VECTOR ( 'NONE', #2859, 1000.000000000000000 ) ;
#9149=DIRECTION ( 'NONE',  ( 0.000000000000000000, -1.000000000000000000, 0.000000000000000000 ) ) ;
#9156=CARTESIAN_POINT ( 'NONE',  ( 158.0000000000007105, 138.2401247522676044, 45.00000000000000000 ) ) ;
#9158=CARTESIAN_POINT ( 'NONE',  ( 157.9999999999998010, 236.0472500450420341, -45.00000000000000000 ) ) ;
#9159=CARTESIAN_POINT ( 'NONE',  ( 158.0000000000004547, 163.8267498348450886, 45.00000000000000000 ) ) ;
#9162=ADVANCED_FACE ( 'NONE', ( #5018 ), #24710, .T. ) ;
#9163=VECTOR ( 'NONE', #27855, 1000.000000000000000 ) ;
#9165=ORIENTED_EDGE ( 'NONE', *, *, #18979, .T. ) ;
#9171=ORIENTED_EDGE ( 'NONE', *, *, #2105, .F. ) ;
#9173=PLANE ( 'NONE',  #14122 ) ;
#9179=LINE ( 'NONE', #22535, #190 ) ;
#9184=DIRECTION ( 'NONE',  ( -0.8916010070299273949, -0.4528218681371510845, 0.000000000000000000 ) ) ;
#9186=LINE ( 'NONE', #14981, #12903 ) ;
#9187=DIRECTION ( 'NONE',  ( -0.8916010070297643031, 0.4528218681374719390, 0.000000000000000000 ) ) ;
#9194=CARTESIAN_POINT ( 'NONE',  ( 157.9999999999998010, 233.5393750375350237, 45.00000000000000000 ) ) ;
#9197=ORIENTED_EDGE ( 'NONE', *, *, #1365, .F. ) ;
#9200=DIRECTION ( 'NONE',  ( -0.8916010070293383105, -0.4528218681383106015, 0.000000000000000000 ) ) ;
#9209=DIRECTION ( 'NONE',  ( -0.000000000000000000, -0.000000000000000000, -1.000000000000000000 ) ) ;
#9212=CARTESIAN_POINT ( 'NONE',  ( 158.0000000000016769, 45.95662448201407102, -45.00000000000000000 ) ) ;
#9213=ORIENTED_EDGE ( 'NONE', *, *, #24150, .F. ) ;
#9215=LINE ( 'NONE', #15687, #7524 ) ;
#9216=CARTESIAN_POINT ( 'NONE',  ( 157.4999999999998579, 73.28931206083800021, -45.00000000000000000 ) ) ;
#9217=CARTESIAN_POINT ( 'NONE',  ( 158.0000000000016485, 50.46449948952111697, 45.00000000000000000 ) ) ;
#9220=DIRECTION ( 'NONE',  ( 0.000000000000000000, -1.000000000000000000, 0.000000000000000000 ) ) ;
#9223=PLANE ( 'NONE',  #11218 ) ;
#9224=VERTEX_POINT ( 'NONE', #24566 ) ;
#9225=EDGE_CURVE ( 'NONE', #8629, #25161, #13662, .T. ) ;
#9227=EDGE_CURVE ( 'NONE', #4314, #17184, #2722, .T. ) ;
#9233=EDGE_CURVE ( 'NONE', #17812, #17412, #26035, .T. ) ;
#9234=ORIENTED_EDGE ( 'NONE', *, *, #12584, .F. ) ;
#9236=LINE ( 'NONE', #13991, #25964 ) ;
#9237=ORIENTED_EDGE ( 'NONE', *, *, #23333, .F. ) ;
#9241=CARTESIAN_POINT ( 'NONE',  ( 158.0000000000003695, 171.3503748573662051, -45.00000000000000000 ) ) ;
#9242=ORIENTED_EDGE ( 'NONE', *, *, #12748, .F. ) ;
#9247=VECTOR ( 'NONE', #13366, 1000.000000000000000 ) ;
#9248=DIRECTION ( 'NONE',  ( 0.000000000000000000, -1.000000000000000000, 0.000000000000000000 ) ) ;
#9251=DIRECTION ( 'NONE',  ( 0.4528218681382713551, 0.8916010070293584056, -0.000000000000000000 ) ) ;
#9253=CARTESIAN_POINT ( 'NONE',  ( 158.0000000000008242, 128.2086247222394206, -45.00000000000000000 ) ) ;
#9254=ORIENTED_EDGE ( 'NONE', *, *, #27843, .T. ) ;
#9258=PLANE ( 'NONE',  #13252 ) ;
#9265=EDGE_CURVE ( 'NONE', #18558, #17461, #27275, .T. ) ;
#9267=DIRECTION ( 'NONE',  ( 0.4528218681382713551, 0.8916010070293584056, -0.000000000000000000 ) ) ;
#9272=EDGE_LOOP ( 'NONE', ( #23937, #4663, #1864, #24821 ) ) ;
#9278=ORIENTED_EDGE ( 'NONE', *, *, #8607, .T. ) ;
#9279=DIRECTION ( 'NONE',  ( -0.8916010070300078860, 0.4528218681369924337, 0.000000000000000000 ) ) ;
#9280=ORIENTED_EDGE ( 'NONE', *, *, #1095, .T. ) ;
#9281=ORIENTED_EDGE ( 'NONE', *, *, #10879, .F. ) ;
#9285=DIRECTION ( 'NONE',  ( -0.8916010070293409751, -0.4528218681383056610, 0.000000000000000000 ) ) ;
#9286=CARTESIAN_POINT ( 'NONE',  ( 158.0000000000000568, 201.4448749474510407, 45.00000000000000000 ) ) ;
#9288=VECTOR ( 'NONE', #8239, 1000.000000000000000 ) ;
#9289=CARTESIAN_POINT ( 'NONE',  ( 158.0000000000002558, 181.3818748873943889, 45.00000000000000000 ) ) ;
#9290=EDGE_CURVE ( 'NONE', #16854, #24374, #11933, .T. ) ;
#9291=DIRECTION ( 'NONE',  ( 0.000000000000000000, -1.000000000000000000, 0.000000000000000000 ) ) ;
#9294=LINE ( 'NONE', #7136, #17677 ) ;
#9298=ORIENTED_EDGE ( 'NONE', *, *, #2759, .F. ) ;
#9302=CARTESIAN_POINT ( 'NONE',  ( 157.4999999999998579, 158.5570623160774630, 45.00000000000000000 ) ) ;
#9306=ORIENTED_EDGE ( 'NONE', *, *, #18754, .F. ) ;
#9313=VERTEX_POINT ( 'NONE', #12074 ) ;
#9316=VERTEX_POINT ( 'NONE', #20674 ) ;
#9319=CARTESIAN_POINT ( 'NONE',  ( 158.0000000000005116, 160.8109998198309825, -45.00000000000000000 ) ) ;
#9323=DIRECTION ( 'NONE',  ( -0.8916010070294706491, -0.4528218681380501986, 0.000000000000000000 ) ) ;
#9324=AXIS2_PLACEMENT_3D ( 'NONE', #3051, #20443, #5353 ) ;
#9327=EDGE_CURVE ( 'NONE', #25161, #18388, #16380, .T. ) ;
#9328=CARTESIAN_POINT ( 'NONE',  ( 158.0000000000000853, 198.4291249324366504, 45.00000000000000000 ) ) ;
#9333=CARTESIAN_POINT ( 'NONE',  ( 157.9999999999998010, 241.0630000600560550, 45.00000000000000000 ) ) ;
#9334=CARTESIAN_POINT ( 'NONE',  ( 158.0000000000009663, 111.1613746771971876, 45.00000000000000000 ) ) ;
#9342=ORIENTED_EDGE ( 'NONE', *, *, #22508, .T. ) ;
#9343=FACE_OUTER_BOUND ( 'NONE', #22702, .T. ) ;
#9344=ADVANCED_FACE ( 'NONE', ( #14365 ), #14226, .F. ) ;
#9354=ORIENTED_EDGE ( 'NONE', *, *, #11508, .F. ) ;
#9357=CARTESIAN_POINT ( 'NONE',  ( 158.0000000000016769, 47.95662448201407102, 45.00000000000000000 ) ) ;
#9358=EDGE_CURVE ( 'NONE', #14502, #25694, #14088, .T. ) ;
#9361=ORIENTED_EDGE ( 'NONE', *, *, #7519, .T. ) ;
#9365=ADVANCED_FACE ( 'NONE', ( #18387 ), #5307, .F. ) ;
#9366=DIRECTION ( 'NONE',  ( -0.000000000000000000, -0.000000000000000000, -1.000000000000000000 ) ) ;
#9374=AXIS2_PLACEMENT_3D ( 'NONE', #20842, #22999, #23535 ) ;
#9375=LINE ( 'NONE', #7214, #25879 ) ;
#9376=ORIENTED_EDGE ( 'NONE', *, *, #13189, .T. ) ;
#9381=DIRECTION ( 'NONE',  ( 0.000000000000000000, -1.000000000000000000, 0.000000000000000000 ) ) ;
#9383=VERTEX_POINT ( 'NONE', #3564 ) ;
#9385=LINE ( 'NONE', #26901, #13126 ) ;
#9386=VERTEX_POINT ( 'NONE', #21095 ) ;
#9391=LINE ( 'NONE', #3184, #25396 ) ;
#9392=ORIENTED_EDGE ( 'NONE', *, *, #10352, .F. ) ;
#9394=ORIENTED_EDGE ( 'NONE', *, *, #10266, .T. ) ;
#9395=VECTOR ( 'NONE', #5270, 1000.000000000000227 ) ;
#9398=CARTESIAN_POINT ( 'NONE',  ( 157.4999999999998579, 75.79718706834503905, -45.00000000000000000 ) ) ;
#9400=DIRECTION ( 'NONE',  ( -0.000000000000000000, -0.000000000000000000, -1.000000000000000000 ) ) ;
#9406=DIRECTION ( 'NONE',  ( -0.000000000000000000, -0.000000000000000000, -1.000000000000000000 ) ) ;
#9409=CARTESIAN_POINT ( 'NONE',  ( 157.9999999999997726, 246.0787500750700474, -45.00000000000000000 ) ) ;
#9411=AXIS2_PLACEMENT_3D ( 'NONE', #26694, #12933, #17655 ) ;
#9417=ORIENTED_EDGE ( 'NONE', *, *, #2225, .F. ) ;
#9420=EDGE_CURVE ( 'NONE', #7851, #16902, #13340, .T. ) ;
#9422=VERTEX_POINT ( 'NONE', #24381 ) ;
#9424=VERTEX_POINT ( 'NONE', #19785 ) ;
#9427=VERTEX_POINT ( 'NONE', #26827 ) ;
#9428=PLANE ( 'NONE',  #25088 ) ;
#9429=ORIENTED_EDGE ( 'NONE', *, *, #8505, .F. ) ;
#9433=VECTOR ( 'NONE', #15053, 1000.000000000000000 ) ;
#9434=ADVANCED_FACE ( 'NONE', ( #22231 ), #20217, .F. ) ;
#9441=PLANE ( 'NONE',  #8989 ) ;
#9444=PLANE ( 'NONE',  #3912 ) ;
#9449=DIRECTION ( 'NONE',  ( 0.000000000000000000, -1.000000000000000000, 0.000000000000000000 ) ) ;
#9450=ADVANCED_FACE ( 'NONE', ( #19931 ), #17772, .F. ) ;
#9454=DIRECTION ( 'NONE',  ( 0.000000000000000000, -1.000000000000000000, 0.000000000000000000 ) ) ;
#9458=VERTEX_POINT ( 'NONE', #13773 ) ;
#9461=VECTOR ( 'NONE', #14489, 1000.000000000000000 ) ;
#9466=ORIENTED_EDGE ( 'NONE', *, *, #21572, .F. ) ;
#9467=LINE ( 'NONE', #22384, #3543 ) ;
#9468=LINE ( 'NONE', #22242, #9527 ) ;
#9469=DIRECTION ( 'NONE',  ( -0.000000000000000000, -0.000000000000000000, -1.000000000000000000 ) ) ;
#9471=EDGE_CURVE ( 'NONE', #19742, #7009, #26671, .T. ) ;
#9482=CARTESIAN_POINT ( 'NONE',  ( 157.9999999999996305, 286.2047501951820436, -45.00000000000000000 ) ) ;
#9486=CARTESIAN_POINT ( 'NONE',  ( 157.4999999999998579, 110.9074371734436255, 45.00000000000000000 ) ) ;
#9490=DIRECTION ( 'NONE',  ( 0.8916010070300282031, -0.4528218681369524101, 0.000000000000000000 ) ) ;
#9493=VECTOR ( 'NONE', #22492, 1000.000000000000000 ) ;
#9494=VERTEX_POINT ( 'NONE', #6715 ) ;
#9497=CARTESIAN_POINT ( 'NONE',  ( 157.9999999999997158, 256.6181251126050711, 45.00000000000000000 ) ) ;
#9501=DIRECTION ( 'NONE',  ( 0.8916010070293584056, -0.4528218681382712996, 0.000000000000000000 ) ) ;
#9504=DIRECTION ( 'NONE',  ( -0.8916010070293383105, -0.4528218681383106015, 0.000000000000000000 ) ) ;
#9507=ADVANCED_FACE ( 'NONE', ( #1103 ), #3104, .F. ) ;
#9509=DIRECTION ( 'NONE',  ( -0.8916010070297746282, 0.4528218681374520105, 0.000000000000000000 ) ) ;
#9515=DIRECTION ( 'NONE',  ( 0.000000000000000000, -1.000000000000000000, 0.000000000000000000 ) ) ;
#9516=DIRECTION ( 'NONE',  ( 0.8916010070293384215, 0.4528218681383106015, 0.000000000000000000 ) ) ;
#9517=VERTEX_POINT ( 'NONE', #14059 ) ;
#9518=LINE ( 'NONE', #27298, #14218 ) ;
#9523=EDGE_CURVE ( 'NONE', #17073, #8883, #22942, .T. ) ;
#9527=VECTOR ( 'NONE', #24393, 1000.000000000000000 ) ;
#9528=ORIENTED_EDGE ( 'NONE', *, *, #9732, .T. ) ;
#9530=CARTESIAN_POINT ( 'NONE',  ( 158.0000000000005684, 151.2873747973098659, 45.00000000000000000 ) ) ;
#9531=CARTESIAN_POINT ( 'NONE',  ( 157.4999999999998579, 135.9861872485140850, -45.00000000000000000 ) ) ;
#9535=DIRECTION ( 'NONE',  ( 0.8916010070297037959, -0.4528218681375912325, 0.000000000000000000 ) ) ;
#9536=ADVANCED_FACE ( 'NONE', ( #16483 ), #16210, .F. ) ;
#9537=EDGE_CURVE ( 'NONE', #21780, #4389, #11763, .T. ) ;
#9541=DIRECTION ( 'NONE',  ( 0.8916010070297041290, 0.4528218681375906218, 0.000000000000000000 ) ) ;
#9542=PLANE ( 'NONE',  #25272 ) ;
#9547=CARTESIAN_POINT ( 'NONE',  ( 157.4999999999998579, 221.2539375037535194, 45.00000000000000000 ) ) ;
#9548=DIRECTION ( 'NONE',  ( 0.4528218681378310406, 0.8916010070295820045, -0.000000000000000000 ) ) ;
#9549=DIRECTION ( 'NONE',  ( 0.8916010070299470458, -0.4528218681371123377, 0.000000000000000000 ) ) ;
#9550=ORIENTED_EDGE ( 'NONE', *, *, #24633, .F. ) ;
#9552=CARTESIAN_POINT ( 'NONE',  ( 157.4999999999998579, 123.4468122109788482, 45.00000000000000000 ) ) ;
#9553=ORIENTED_EDGE ( 'NONE', *, *, #26309, .F. ) ;
#9554=EDGE_CURVE ( 'NONE', #6691, #25965, #18770, .T. ) ;
#9555=DIRECTION ( 'NONE',  ( -0.000000000000000000, -0.000000000000000000, -1.000000000000000000 ) ) ;
#9559=DIRECTION ( 'NONE',  ( 0.8916010070298961976, -0.4528218681372121468, 0.000000000000000000 ) ) ;
#9560=DIRECTION ( 'NONE',  ( -0.8916010070293510781, 0.4528218681382856214, 0.000000000000000000 ) ) ;
#9561=ORIENTED_EDGE ( 'NONE', *, *, #24879, .F. ) ;
#9570=VECTOR ( 'NONE', #9406, 1000.000000000000000 ) ;
#9580=CARTESIAN_POINT ( 'NONE',  ( 157.4999999999998579, 201.1909374436971802, 45.00000000000000000 ) ) ;
#9581=DIRECTION ( 'NONE',  ( -0.8916010070295820045, -0.4528218681378310406, 0.000000000000000000 ) ) ;
#9583=CARTESIAN_POINT ( 'NONE',  ( 157.9999999999997442, 254.1102501050980322, 45.00000000000000000 ) ) ;
#9584=DIRECTION ( 'NONE',  ( 0.4528218681381102617, -0.8916010070294402290, 0.000000000000000000 ) ) ;
#9585=ORIENTED_EDGE ( 'NONE', *, *, #20503, .T. ) ;
#9586=VECTOR ( 'NONE', #20633, 1000.000000000000000 ) ;
#9587=VECTOR ( 'NONE', #7312, 1000.000000000000000 ) ;
#9593=VECTOR ( 'NONE', #2444, 1000.000000000000114 ) ;
#9594=EDGE_CURVE ( 'NONE', #8173, #21166, #27516, .T. ) ;
#9598=EDGE_CURVE ( 'NONE', #4619, #14425, #23087, .T. ) ;
#9600=VECTOR ( 'NONE', #1340, 1000.000000000000000 ) ;
#9601=VERTEX_POINT ( 'NONE', #27242 ) ;
#9605=DIRECTION ( 'NONE',  ( 0.4528218681376712240, 0.8916010070296632728, -0.000000000000000000 ) ) ;
#9608=DIRECTION ( 'NONE',  ( -0.000000000000000000, -0.000000000000000000, -1.000000000000000000 ) ) ;
#9613=CARTESIAN_POINT ( 'NONE',  ( 157.9999999999996589, 276.6811251726610976, -45.00000000000000000 ) ) ;
#9614=EDGE_CURVE ( 'NONE', #18134, #1534, #826, .T. ) ;
#9622=LINE ( 'NONE', #23255, #7868 ) ;
#9625=ORIENTED_EDGE ( 'NONE', *, *, #7031, .F. ) ;
#9627=PLANE ( 'NONE',  #5931 ) ;
#9634=VECTOR ( 'NONE', #27285, 1000.000000000000000 ) ;
#9637=CARTESIAN_POINT ( 'NONE',  ( 157.4999999999998579, 201.1909374436971802, 45.00000000000000000 ) ) ;
#9638=VERTEX_POINT ( 'NONE', #16895 ) ;
#9641=CARTESIAN_POINT ( 'NONE',  ( 157.4999999999998579, 83.32081209086616980, -45.00000000000000000 ) ) ;
#9643=CARTESIAN_POINT ( 'NONE',  ( 158.0000000000002842, 178.8739998798873216, -45.00000000000000000 ) ) ;
#9651=CARTESIAN_POINT ( 'NONE',  ( 157.4999999999997442, 256.3641876088515232, 45.00000000000000000 ) ) ;
#9653=CARTESIAN_POINT ( 'NONE',  ( 158.0000000000006253, 146.2716247822957598, 45.00000000000000000 ) ) ;
#9655=ORIENTED_EDGE ( 'NONE', *, *, #3785, .F. ) ;
#9656=CARTESIAN_POINT ( 'NONE',  ( 157.4999999999998295, 226.2696875187675118, 45.00000000000000000 ) ) ;
#9658=VECTOR ( 'NONE', #5956, 1000.000000000000114 ) ;
#9659=EDGE_CURVE ( 'NONE', #26528, #1795, #27656, .T. ) ;
#9662=ORIENTED_EDGE ( 'NONE', *, *, #17251, .T. ) ;
#9664=VECTOR ( 'NONE', #18176, 1000.000000000000000 ) ;
#9667=VERTEX_POINT ( 'NONE', #15032 ) ;
#9671=DIRECTION ( 'NONE',  ( 1.000000000000000000, -0.000000000000000000, -0.000000000000000000 ) ) ;
#9673=CARTESIAN_POINT ( 'NONE',  ( 158.0000000000000000, 206.4606249624626457, 45.00000000000000000 ) ) ;
#9674=VERTEX_POINT ( 'NONE', #17035 ) ;
#9676=VECTOR ( 'NONE', #13754, 1000.000000000000000 ) ;
#9678=CARTESIAN_POINT ( 'NONE',  ( 158.0000000000014211, 70.52749954957745615, 45.00000000000000000 ) ) ;
#9685=CARTESIAN_POINT ( 'NONE',  ( 187.4999999999996305, 288.9665627064425166, 45.00000000000000000 ) ) ;
#9686=PLANE ( 'NONE',  #91 ) ;
#9688=ORIENTED_EDGE ( 'NONE', *, *, #16523, .F. ) ;
#9695=LINE ( 'NONE', #22195, #13857 ) ;
#9697=VERTEX_POINT ( 'NONE', #8135 ) ;
#9702=ORIENTED_EDGE ( 'NONE', *, *, #13189, .F. ) ;
#9703=ORIENTED_EDGE ( 'NONE', *, *, #23058, .F. ) ;
#9709=EDGE_CURVE ( 'NONE', #8771, #23789, #4241, .T. ) ;
#9712=LINE ( 'NONE', #20484, #25005 ) ;
#9713=CARTESIAN_POINT ( 'NONE',  ( 158.0000000000001705, 190.9054999099155054, 45.00000000000000000 ) ) ;
#9714=LINE ( 'NONE', #18054, #21575 ) ;
#9717=CARTESIAN_POINT ( 'NONE',  ( 158.0000000000000568, 203.4448749474510407, 45.00000000000000000 ) ) ;
#9718=VECTOR ( 'NONE', #12449, 1000.000000000000000 ) ;
#9722=VECTOR ( 'NONE', #7920, 1000.000000000000114 ) ;
#9724=FACE_OUTER_BOUND ( 'NONE', #8237, .T. ) ;
#9728=DIRECTION ( 'NONE',  ( -0.8916010070295922185, 0.4528218681378110011, 0.000000000000000000 ) ) ;
#9732=EDGE_CURVE ( 'NONE', #14031, #10648, #1798, .T. ) ;
#9735=ORIENTED_EDGE ( 'NONE', *, *, #20496, .T. ) ;
#9737=ORIENTED_EDGE ( 'NONE', *, *, #25783, .F. ) ;
#9742=VECTOR ( 'NONE', #11516, 1000.000000000000114 ) ;
#9745=CARTESIAN_POINT ( 'NONE',  ( 158.0000000000011369, 96.11412463215494029, 45.00000000000000000 ) ) ;
#9751=PLANE ( 'NONE',  #24496 ) ;
#9756=CARTESIAN_POINT ( 'NONE',  ( 157.9999999999998010, 241.0630000600560550, 45.00000000000000000 ) ) ;
#9757=LINE ( 'NONE', #7600, #25470 ) ;
#9758=EDGE_CURVE ( 'NONE', #3282, #6570, #22054, .T. ) ;
#9759=CARTESIAN_POINT ( 'NONE',  ( 158.0000000000002274, 185.8897498949014278, 45.00000000000000000 ) ) ;
#9762=AXIS2_PLACEMENT_3D ( 'NONE', #14448, #23062, #3371 ) ;
#9767=VECTOR ( 'NONE', #19404, 1000.000000000000000 ) ;
#9769=ORIENTED_EDGE ( 'NONE', *, *, #5841, .F. ) ;
#9770=VECTOR ( 'NONE', #20396, 1000.000000000000000 ) ;
#9773=ORIENTED_EDGE ( 'NONE', *, *, #19865, .T. ) ;
#9774=VERTEX_POINT ( 'NONE', #367 ) ;
#9779=CARTESIAN_POINT ( 'NONE',  ( 157.9999999999996305, 286.2047501951820436, 45.00000000000000000 ) ) ;
#9780=VECTOR ( 'NONE', #25121, 1000.000000000000000 ) ;
#9786=EDGE_CURVE ( 'NONE', #18620, #6585, #17740, .T. ) ;
#9793=DIRECTION ( 'NONE',  ( -0.000000000000000000, -0.000000000000000000, -1.000000000000000000 ) ) ;
#9795=VECTOR ( 'NONE', #7491, 1000.000000000000114 ) ;
#9800=ORIENTED_EDGE ( 'NONE', *, *, #14950, .F. ) ;
#9804=CARTESIAN_POINT ( 'NONE',  ( 157.9999999999999716, 208.9684999699701393, 45.00000000000000000 ) ) ;
#9807=LINE ( 'NONE', #8208, #22815 ) ;
#9809=CARTESIAN_POINT ( 'NONE',  ( 158.0000000000016200, 50.97237449702815582, -45.00000000000000000 ) ) ;
#9815=EDGE_CURVE ( 'NONE', #8138, #22744, #2361, .T. ) ;
#9816=EDGE_CURVE ( 'NONE', #21445, #4287, #26794, .T. ) ;
#9818=DIRECTION ( 'NONE',  ( 0.000000000000000000, -1.000000000000000000, 0.000000000000000000 ) ) ;
#9820=VECTOR ( 'NONE', #21615, 1000.000000000000000 ) ;
#9827=CARTESIAN_POINT ( 'NONE',  ( 158.0000000000000000, 208.4606249624626457, 45.00000000000000000 ) ) ;
#9828=ORIENTED_EDGE ( 'NONE', *, *, #12097, .T. ) ;
#9829=CARTESIAN_POINT ( 'NONE',  ( 158.0000000000002558, 181.3818748873943889, -45.00000000000000000 ) ) ;
#9834=ORIENTED_EDGE ( 'NONE', *, *, #3310, .F. ) ;
#9835=CARTESIAN_POINT ( 'NONE',  ( 157.9999999999997442, 256.1102501050980322, 45.00000000000000000 ) ) ;
#9840=CARTESIAN_POINT ( 'NONE',  ( 158.0000000000003979, 170.8424998498591663, -45.00000000000000000 ) ) ;
#9841=ORIENTED_EDGE ( 'NONE', *, *, #12034, .F. ) ;
#9843=ORIENTED_EDGE ( 'NONE', *, *, #13947, .F. ) ;
#9844=PLANE ( 'NONE',  #20035 ) ;
#9859=AXIS2_PLACEMENT_3D ( 'NONE', #23926, #14893, #23781 ) ;
#9860=DIRECTION ( 'NONE',  ( 0.000000000000000000, -1.000000000000000000, 0.000000000000000000 ) ) ;
#9861=DIRECTION ( 'NONE',  ( 0.8916010070299883461, 0.4528218681370311249, 0.000000000000000000 ) ) ;
#9868=VERTEX_POINT ( 'NONE', #28353 ) ;
#9869=ADVANCED_FACE ( 'NONE', ( #17456 ), #20891, .F. ) ;
#9870=DIRECTION ( 'NONE',  ( -0.000000000000000000, 0.000000000000000000, -1.000000000000000000 ) ) ;
#9871=ORIENTED_EDGE ( 'NONE', *, *, #1149, .F. ) ;
#9876=ORIENTED_EDGE ( 'NONE', *, *, #24404, .T. ) ;
#9882=CARTESIAN_POINT ( 'NONE',  ( 157.9999999999996305, 283.6968751876750616, 45.00000000000000000 ) ) ;
#9884=DIRECTION ( 'NONE',  ( -0.8916010070293584056, 0.4528218681382713551, 0.000000000000000000 ) ) ;
#9887=FACE_OUTER_BOUND ( 'NONE', #14819, .T. ) ;
#9888=CARTESIAN_POINT ( 'NONE',  ( 157.4999999999998579, 50.71843699327460797, 45.00000000000000000 ) ) ;
#9893=DIRECTION ( 'NONE',  ( 0.8916010070293584056, -0.4528218681382712996, 0.000000000000000000 ) ) ;
#9902=FACE_OUTER_BOUND ( 'NONE', #21917, .T. ) ;
#9908=EDGE_CURVE ( 'NONE', #11767, #12751, #18734, .T. ) ;
#9909=EDGE_CURVE ( 'NONE', #5308, #10360, #22486, .T. ) ;
#9914=ORIENTED_EDGE ( 'NONE', *, *, #7705, .F. ) ;
#9921=CARTESIAN_POINT ( 'NONE',  ( 158.0000000000015064, 61.00387452705632541, -45.00000000000000000 ) ) ;
#9925=DIRECTION ( 'NONE',  ( 0.8916010070299672519, -0.4528218681370723142, 0.000000000000000000 ) ) ;
#9927=LINE ( 'NONE', #18820, #11885 ) ;
#9928=FACE_OUTER_BOUND ( 'NONE', #15753, .T. ) ;
#9929=DIRECTION ( 'NONE',  ( -0.8916010070293283185, -0.4528218681383305855, 0.000000000000000000 ) ) ;
#9930=CARTESIAN_POINT ( 'NONE',  ( 158.0000000000016485, 48.46449948952110987, 45.00000000000000000 ) ) ;
#9938=ORIENTED_EDGE ( 'NONE', *, *, #19617, .F. ) ;
#9941=CARTESIAN_POINT ( 'NONE',  ( 157.4999999999998579, 88.33656210588026170, 45.00000000000000000 ) ) ;
#9943=ORIENTED_EDGE ( 'NONE', *, *, #111, .F. ) ;
#9948=ORIENTED_EDGE ( 'NONE', *, *, #16340, .T. ) ;
#9957=CARTESIAN_POINT ( 'NONE',  ( 157.4999999999998579, 221.2539375037535194, -45.00000000000000000 ) ) ;
#9959=ORIENTED_EDGE ( 'NONE', *, *, #2759, .T. ) ;
#9961=DIRECTION ( 'NONE',  ( 0.000000000000000000, 0.000000000000000000, -1.000000000000000000 ) ) ;
#9963=DIRECTION ( 'NONE',  ( 0.8916010070295614653, -0.4528218681378716193, 0.000000000000000000 ) ) ;
#9964=PLANE ( 'NONE',  #17604 ) ;
#9968=CARTESIAN_POINT ( 'NONE',  ( 158.0000000000014211, 71.03537455708449500, 45.00000000000000000 ) ) ;
#9969=CARTESIAN_POINT ( 'NONE',  ( 157.9999999999997726, 246.5866250825770294, 45.00000000000000000 ) ) ;
#9971=VERTEX_POINT ( 'NONE', #7821 ) ;
#9974=EDGE_CURVE ( 'NONE', #11698, #2950, #11729, .T. ) ;
#9975=EDGE_LOOP ( 'NONE', ( #15035, #14572, #18669, #1161 ) ) ;
#9977=EDGE_CURVE ( 'NONE', #11698, #3367, #16450, .T. ) ;
#9981=ADVANCED_FACE ( 'NONE', ( #26040 ), #7961, .F. ) ;
#9984=ORIENTED_EDGE ( 'NONE', *, *, #19704, .F. ) ;
#9986=EDGE_LOOP ( 'NONE', ( #9361, #16922, #18318, #18180 ) ) ;
#9987=ORIENTED_EDGE ( 'NONE', *, *, #25002, .F. ) ;
#9988=ORIENTED_EDGE ( 'NONE', *, *, #19694, .F. ) ;
#9989=PLANE ( 'NONE',  #18469 ) ;
#10002=ORIENTED_EDGE ( 'NONE', *, *, #1996, .F. ) ;
#10004=EDGE_CURVE ( 'NONE', #3340, #14776, #4058, .T. ) ;
#10005=EDGE_CURVE ( 'NONE', #17429, #26528, #10540, .T. ) ;
#10007=DIRECTION ( 'NONE',  ( 0.8916010070295922185, 0.4528218681378110011, 0.000000000000000000 ) ) ;
#10012=DIRECTION ( 'NONE',  ( 0.8916010070297338830, -0.4528218681375318910, 0.000000000000000000 ) ) ;
#10019=EDGE_CURVE ( 'NONE', #12783, #27491, #12710, .T. ) ;
#10021=ORIENTED_EDGE ( 'NONE', *, *, #585, .T. ) ;
#10022=ORIENTED_EDGE ( 'NONE', *, *, #3698, .T. ) ;
#10024=CARTESIAN_POINT ( 'NONE',  ( 157.4999999999998579, 135.9861872485140850, 45.00000000000000000 ) ) ;
#10030=CARTESIAN_POINT ( 'NONE',  ( 158.0000000000004832, 163.3188748273380213, 45.00000000000000000 ) ) ;
#10032=CARTESIAN_POINT ( 'NONE',  ( 158.0000000000007390, 135.7322497447605656, 45.00000000000000000 ) ) ;
#10033=VECTOR ( 'NONE', #18160, 1000.000000000000227 ) ;
#10037=LINE ( 'NONE', #14495, #8383 ) ;
#10044=VECTOR ( 'NONE', #27925, 1000.000000000000000 ) ;
#10048=ORIENTED_EDGE ( 'NONE', *, *, #13485, .T. ) ;
#10056=PLANE ( 'NONE',  #7207 ) ;
#10059=PLANE ( 'NONE',  #11658 ) ;
#10060=EDGE_CURVE ( 'NONE', #23339, #25239, #14716, .T. ) ;
#10061=CARTESIAN_POINT ( 'NONE',  ( 157.4999999999998579, 186.1436873986549188, -45.00000000000000000 ) ) ;
#10062=EDGE_CURVE ( 'NONE', #27410, #21564, #5802, .T. ) ;
#10066=CARTESIAN_POINT ( 'NONE',  ( 158.0000000000000853, 198.9369999399436892, 45.00000000000000000 ) ) ;
#10067=LINE ( 'NONE', #19104, #10680 ) ;
#10068=VECTOR ( 'NONE', #11353, 1000.000000000000114 ) ;
#10075=LINE ( 'NONE', #11960, #5304 ) ;
#10078=ORIENTED_EDGE ( 'NONE', *, *, #16975, .T. ) ;
#10081=EDGE_CURVE ( 'NONE', #23544, #22677, #14438, .T. ) ;
#10087=CARTESIAN_POINT ( 'NONE',  ( 158.0000000000004263, 166.3346248423521274, 45.00000000000000000 ) ) ;
#10090=CARTESIAN_POINT ( 'NONE',  ( 157.9999999999998295, 229.0315000300280417, 45.00000000000000000 ) ) ;
#10093=ORIENTED_EDGE ( 'NONE', *, *, #8488, .F. ) ;
#10096=PLANE ( 'NONE',  #10303 ) ;
#10097=CARTESIAN_POINT ( 'NONE',  ( 158.0000000000002274, 183.8897498949014278, 45.00000000000000000 ) ) ;
#10098=CARTESIAN_POINT ( 'NONE',  ( 157.4999999999998579, 176.1121873686267350, -45.00000000000000000 ) ) ;
#10100=EDGE_CURVE ( 'NONE', #7159, #2485, #16729, .T. ) ;
#10106=EDGE_CURVE ( 'NONE', #24140, #22209, #18873, .T. ) ;
#10108=LINE ( 'NONE', #15921, #3227 ) ;
#10109=DIRECTION ( 'NONE',  ( 0.4528218681380702382, -0.8916010070294605461, 0.000000000000000000 ) ) ;
#10111=ORIENTED_EDGE ( 'NONE', *, *, #15112, .F. ) ;
#10115=AXIS2_PLACEMENT_3D ( 'NONE', #25000, #7341, #11804 ) ;
#10120=CARTESIAN_POINT ( 'NONE',  ( 157.4999999999998010, 241.3169375638095460, 45.00000000000000000 ) ) ;
#10122=ORIENTED_EDGE ( 'NONE', *, *, #15075, .T. ) ;
#10123=DIRECTION ( 'NONE',  ( -0.000000000000000000, -0.000000000000000000, -1.000000000000000000 ) ) ;
#10125=ORIENTED_EDGE ( 'NONE', *, *, #19407, .T. ) ;
#10126=VERTEX_POINT ( 'NONE', #12429 ) ;
#10133=AXIS2_PLACEMENT_3D ( 'NONE', #6572, #18859, #14283 ) ;
#10135=EDGE_CURVE ( 'NONE', #18450, #12823, #21168, .T. ) ;
#10136=CARTESIAN_POINT ( 'NONE',  ( 158.0000000000004547, 165.8267498348450886, 45.00000000000000000 ) ) ;
#10138=CARTESIAN_POINT ( 'NONE',  ( 157.4999999999998579, 196.1751874286831026, -45.00000000000000000 ) ) ;
#10140=DIRECTION ( 'NONE',  ( -0.8916010070299780210, -0.4528218681370510534, 0.000000000000000000 ) ) ;
#10142=LINE ( 'NONE', #13428, #16369 ) ;
#10143=CARTESIAN_POINT ( 'NONE',  ( 158.0000000000005684, 153.2873747973098659, -45.00000000000000000 ) ) ;
#10144=DIRECTION ( 'NONE',  ( 0.8916010070299267287, -0.4528218681371523058, 0.000000000000000000 ) ) ;
#10147=LINE ( 'NONE', #17170, #13730 ) ;
#10149=CARTESIAN_POINT ( 'NONE',  ( 157.4999999999996589, 276.4271876689075498, 45.00000000000000000 ) ) ;
#10152=CARTESIAN_POINT ( 'NONE',  ( 158.0000000000005684, 151.2873747973098659, -45.00000000000000000 ) ) ;
#10153=ORIENTED_EDGE ( 'NONE', *, *, #7890, .T. ) ;
#10154=VECTOR ( 'NONE', #18822, 1000.000000000000000 ) ;
#10158=ORIENTED_EDGE ( 'NONE', *, *, #2169, .F. ) ;
#10161=ORIENTED_EDGE ( 'NONE', *, *, #3175, .F. ) ;
#10163=DIRECTION ( 'NONE',  ( -0.000000000000000000, -0.000000000000000000, -1.000000000000000000 ) ) ;
#10165=CARTESIAN_POINT ( 'NONE',  ( 157.4999999999998579, 65.76568703831686946, 45.00000000000000000 ) ) ;
#10169=VECTOR ( 'NONE', #23188, 1000.000000000000000 ) ;
#10172=DIRECTION ( 'NONE',  ( 0.8916010070294699830, -0.4528218681380514199, 0.000000000000000000 ) ) ;
#10177=CARTESIAN_POINT ( 'NONE',  ( 157.4999999999998579, 60.74993702330277756, -45.00000000000000000 ) ) ;
#10182=LINE ( 'NONE', #1830, #25294 ) ;
#10184=ORIENTED_EDGE ( 'NONE', *, *, #10666, .F. ) ;
#10185=VECTOR ( 'NONE', #15167, 1000.000000000000114 ) ;
#10188=ORIENTED_EDGE ( 'NONE', *, *, #17648, .T. ) ;
#10191=ORIENTED_EDGE ( 'NONE', *, *, #5812, .T. ) ;
#10196=VERTEX_POINT ( 'NONE', #20001 ) ;
#10199=DIRECTION ( 'NONE',  ( 0.000000000000000000, -1.000000000000000000, 0.000000000000000000 ) ) ;
#10204=EDGE_CURVE ( 'NONE', #24279, #14031, #12993, .T. ) ;
#10206=FACE_OUTER_BOUND ( 'NONE', #16452, .T. ) ;
#10209=EDGE_CURVE ( 'NONE', #13594, #26578, #9088, .T. ) ;
#10213=CARTESIAN_POINT ( 'NONE',  ( 157.9999999999997158, 256.6181251126050711, -45.00000000000000000 ) ) ;
#10215=DIRECTION ( 'NONE',  ( -0.8916010070293483025, -0.4528218681382912281, 0.000000000000000000 ) ) ;
#10221=ORIENTED_EDGE ( 'NONE', *, *, #7225, .T. ) ;
#10222=VECTOR ( 'NONE', #21907, 1000.000000000000000 ) ;
#10224=LINE ( 'NONE', #3319, #26892 ) ;
#10225=ORIENTED_EDGE ( 'NONE', *, *, #25881, .T. ) ;
#10226=AXIS2_PLACEMENT_3D ( 'NONE', #26277, #1999, #17509 ) ;
#10228=CARTESIAN_POINT ( 'NONE',  ( 157.9999999999996305, 284.2047501951820436, -45.00000000000000000 ) ) ;
#10237=LINE ( 'NONE', #16842, #23670 ) ;
#10244=DIRECTION ( 'NONE',  ( -0.8916010070293409751, -0.4528218681383056610, 0.000000000000000000 ) ) ;
#10245=ORIENTED_EDGE ( 'NONE', *, *, #6781, .F. ) ;
#10246=EDGE_CURVE ( 'NONE', #12285, #18364, #4620, .T. ) ;
#10250=CARTESIAN_POINT ( 'NONE',  ( 158.0000000000015632, 55.98812451204224061, -45.00000000000000000 ) ) ;
#10251=ORIENTED_EDGE ( 'NONE', *, *, #24504, .T. ) ;
#10253=ORIENTED_EDGE ( 'NONE', *, *, #27367, .T. ) ;
#10260=ADVANCED_FACE ( 'NONE', ( #24040 ), #4202, .F. ) ;
#10264=AXIS2_PLACEMENT_3D ( 'NONE', #22425, #15977, #13970 ) ;
#10266=EDGE_CURVE ( 'NONE', #9316, #9424, #22160, .T. ) ;
#10267=FACE_OUTER_BOUND ( 'NONE', #1738, .T. ) ;
#10270=EDGE_CURVE ( 'NONE', #372, #1220, #8801, .T. ) ;
#10271=ORIENTED_EDGE ( 'NONE', *, *, #1640, .T. ) ;
#10277=SHAPE_REPRESENTATION ( 'Gear Rack', ( #10637 ), #15244 ) ;
#10282=CARTESIAN_POINT ( 'NONE',  ( 158.0000000000002842, 180.8739998798873501, -45.00000000000000000 ) ) ;
#10284=DIRECTION ( 'NONE',  ( -0.8916010070297953893, -0.4528218681374107657, 0.000000000000000000 ) ) ;
#10286=AXIS2_PLACEMENT_3D ( 'NONE', #13568, #6939, #17575 ) ;
#10287=LINE ( 'NONE', #19178, #10044 ) ;
#10290=DIRECTION ( 'NONE',  ( -0.000000000000000000, -0.000000000000000000, -1.000000000000000000 ) ) ;
#10295=ORIENTED_EDGE ( 'NONE', *, *, #20447, .F. ) ;
#10298=EDGE_CURVE ( 'NONE', #27610, #25616, #2466, .T. ) ;
#10301=ORIENTED_EDGE ( 'NONE', *, *, #8113, .F. ) ;
#10303=AXIS2_PLACEMENT_3D ( 'NONE', #18851, #24764, #5071 ) ;
#10305=CARTESIAN_POINT ( 'NONE',  ( 157.4999999999998295, 231.2854375337815327, -45.00000000000000000 ) ) ;
#10307=VECTOR ( 'NONE', #12457, 999.9999999999998863 ) ;
#10318=ORIENTED_EDGE ( 'NONE', *, *, #24047, .F. ) ;
#10320=LINE ( 'NONE', #5581, #4091 ) ;
#10322=ORIENTED_EDGE ( 'NONE', *, *, #10651, .T. ) ;
#10324=VECTOR ( 'NONE', #19532, 1000.000000000000000 ) ;
#10326=ORIENTED_EDGE ( 'NONE', *, *, #17650, .F. ) ;
#10327=ORIENTED_EDGE ( 'NONE', *, *, #3892, .F. ) ;
#10329=VECTOR ( 'NONE', #7816, 1000.000000000000227 ) ;
#10330=VERTEX_POINT ( 'NONE', #2756 ) ;
#10331=EDGE_CURVE ( 'NONE', #13726, #8797, #759, .T. ) ;
#10334=ORIENTED_EDGE ( 'NONE', *, *, #10353, .T. ) ;
#10337=LINE ( 'NONE', #23552, #17859 ) ;
#10338=AXIS2_PLACEMENT_3D ( 'NONE', #3675, #5836, #14330 ) ;
#10339=CARTESIAN_POINT ( 'NONE',  ( 157.9999999999997158, 259.1260001201120531, 45.00000000000000000 ) ) ;
#10342=VECTOR ( 'NONE', #4359, 1000.000000000000000 ) ;
#10343=CARTESIAN_POINT ( 'NONE',  ( 158.0000000000014211, 68.52749954957745615, 45.00000000000000000 ) ) ;
#10345=CARTESIAN_POINT ( 'NONE',  ( 157.4999999999998579, 156.0491873085704242, 45.00000000000000000 ) ) ;
#10346=CARTESIAN_POINT ( 'NONE',  ( 158.0000000000011084, 100.6219996396619791, -45.00000000000000000 ) ) ;
#10347=DIRECTION ( 'NONE',  ( 0.000000000000000000, -1.000000000000000000, 0.000000000000000000 ) ) ;
#10348=CARTESIAN_POINT ( 'NONE',  ( 158.0000000000014779, 63.51174953456337136, 45.00000000000000000 ) ) ;
#10349=ORIENTED_EDGE ( 'NONE', *, *, #18672, .F. ) ;
#10351=EDGE_CURVE ( 'NONE', #23194, #1111, #25030, .T. ) ;
#10352=EDGE_CURVE ( 'NONE', #4162, #23149, #22735, .T. ) ;
#10353=EDGE_CURVE ( 'NONE', #15277, #23733, #12110, .T. ) ;
#10356=AXIS2_PLACEMENT_3D ( 'NONE', #15515, #26546, #4857 ) ;
#10360=VERTEX_POINT ( 'NONE', #9941 ) ;
#10361=DIRECTION ( 'NONE',  ( -0.000000000000000000, -0.000000000000000000, -1.000000000000000000 ) ) ;
#10364=EDGE_CURVE ( 'NONE', #9494, #9427, #26900, .T. ) ;
#10365=ORIENTED_EDGE ( 'NONE', *, *, #24597, .T. ) ;
#10366=VECTOR ( 'NONE', #4573, 1000.000000000000000 ) ;
#10368=PLANE ( 'NONE',  #21879 ) ;
#10372=DIRECTION ( 'NONE',  ( 0.000000000000000000, -1.000000000000000000, 0.000000000000000000 ) ) ;
#10373=ORIENTED_EDGE ( 'NONE', *, *, #27223, .F. ) ;
#10374=CARTESIAN_POINT ( 'NONE',  ( 157.4999999999997442, 256.3641876088515232, -45.00000000000000000 ) ) ;
#10376=LINE ( 'NONE', #8615, #5321 ) ;
#10377=FACE_OUTER_BOUND ( 'NONE', #7963, .T. ) ;
#10378=AXIS2_PLACEMENT_3D ( 'NONE', #11009, #19759, #13036 ) ;
#10385=DIRECTION ( 'NONE',  ( -0.8916010070297036849, 0.4528218681375913435, 0.000000000000000000 ) ) ;
#10390=EDGE_CURVE ( 'NONE', #27901, #14163, #18835, .T. ) ;
#10396=DIRECTION ( 'NONE',  ( 1.000000000000000000, 0.000000000000000000, -0.000000000000000000 ) ) ;
#10397=CARTESIAN_POINT ( 'NONE',  ( 157.9999999999998579, 219.0000000000000284, -45.00000000000000000 ) ) ;
#10398=VERTEX_POINT ( 'NONE', #21130 ) ;
#10399=DIRECTION ( 'NONE',  ( 0.000000000000000000, -1.000000000000000000, 0.000000000000000000 ) ) ;
#10400=FACE_OUTER_BOUND ( 'NONE', #784, .T. ) ;
#10404=PLANE ( 'NONE',  #4893 ) ;
#10406=EDGE_CURVE ( 'NONE', #20034, #20000, #18980, .T. ) ;
#10407=EDGE_CURVE ( 'NONE', #20071, #4844, #27723, .T. ) ;
#10409=ORIENTED_EDGE ( 'NONE', *, *, #19561, .T. ) ;
#10410=LINE ( 'NONE', #1639, #12081 ) ;
#10414=ADVANCED_FACE ( 'NONE', ( #14399 ), #25573, .F. ) ;
#10419=EDGE_CURVE ( 'NONE', #5065, #1356, #7782, .T. ) ;
#10421=CARTESIAN_POINT ( 'NONE',  ( 158.0000000000014495, 66.01962454207041731, 45.00000000000000000 ) ) ;
#10422=LINE ( 'NONE', #12593, #27904 ) ;
#10424=AXIS2_PLACEMENT_3D ( 'NONE', #24754, #13559, #479 ) ;
#10429=FACE_OUTER_BOUND ( 'NONE', #24002, .T. ) ;
#10430=DIRECTION ( 'NONE',  ( -0.000000000000000000, -0.000000000000000000, -1.000000000000000000 ) ) ;
#10433=VERTEX_POINT ( 'NONE', #27862 ) ;
#10437=ORIENTED_EDGE ( 'NONE', *, *, #19337, .F. ) ;
#10439=PLANE ( 'NONE',  #24615 ) ;
#10440=ADVANCED_FACE ( 'NONE', ( #16550 ), #25720, .F. ) ;
#10442=ORIENTED_EDGE ( 'NONE', *, *, #2546, .T. ) ;
#10444=VECTOR ( 'NONE', #1706, 1000.000000000000227 ) ;
#10445=CARTESIAN_POINT ( 'NONE',  ( 157.4999999999997442, 251.3484375938375024, 45.00000000000000000 ) ) ;
#10446=PLANE ( 'NONE',  #7916 ) ;
#10453=CARTESIAN_POINT ( 'NONE',  ( 157.9999999999996874, 271.1575001501400379, -45.00000000000000000 ) ) ;
#10457=ADVANCED_FACE ( 'NONE', ( #10504 ), #26570, .F. ) ;
#10460=VECTOR ( 'NONE', #4434, 1000.000000000000000 ) ;
#10461=VECTOR ( 'NONE', #24332, 1000.000000000000114 ) ;
#10464=ADVANCED_FACE ( 'NONE', ( #24151 ), #11074, .F. ) ;
#10471=ORIENTED_EDGE ( 'NONE', *, *, #22819, .T. ) ;
#10476=DIRECTION ( 'NONE',  ( -0.8916010070299477119, -0.4528218681371110610, 0.000000000000000000 ) ) ;
#10478=VECTOR ( 'NONE', #3409, 1000.000000000000000 ) ;
#10479=DIRECTION ( 'NONE',  ( 0.4528218681383056610, -0.8916010070293409751, 0.000000000000000000 ) ) ;
#10480=FACE_OUTER_BOUND ( 'NONE', #23821, .T. ) ;
#10483=EDGE_CURVE ( 'NONE', #22709, #25403, #17672, .T. ) ;
#10484=DIRECTION ( 'NONE',  ( 0.4528218681372309096, -0.8916010070298868717, 0.000000000000000000 ) ) ;
#10502=VECTOR ( 'NONE', #19125, 1000.000000000000227 ) ;
#10503=ORIENTED_EDGE ( 'NONE', *, *, #20964, .F. ) ;
#10504=FACE_OUTER_BOUND ( 'NONE', #27249, .T. ) ;
#10505=CARTESIAN_POINT ( 'NONE',  ( 157.9999999999997442, 249.0945000900840398, -45.00000000000000000 ) ) ;
#10507=ORIENTED_EDGE ( 'NONE', *, *, #19550, .T. ) ;
#10510=VECTOR ( 'NONE', #11132, 1000.000000000000227 ) ;
#10513=ORIENTED_EDGE ( 'NONE', *, *, #1003, .T. ) ;
#10517=EDGE_CURVE ( 'NONE', #27414, #3041, #302, .T. ) ;
#10523=CARTESIAN_POINT ( 'NONE',  ( 158.0000000000002558, 183.3818748873943889, -45.00000000000000000 ) ) ;
#10528=FACE_OUTER_BOUND ( 'NONE', #14996, .T. ) ;
#10533=DIRECTION ( 'NONE',  ( -0.000000000000000000, -0.000000000000000000, -1.000000000000000000 ) ) ;
#10535=EDGE_LOOP ( 'NONE', ( #20367, #22627, #3425, #21551 ) ) ;
#10537=FACE_OUTER_BOUND ( 'NONE', #27722, .T. ) ;
#10539=AXIS2_PLACEMENT_3D ( 'NONE', #5087, #9267, #6812 ) ;
#10540=LINE ( 'NONE', #16866, #22095 ) ;
#10545=CARTESIAN_POINT ( 'NONE',  ( 157.4999999999998579, 153.5413123010633853, -45.00000000000000000 ) ) ;
#10546=VERTEX_POINT ( 'NONE', #22273 ) ;
#10547=ORIENTED_EDGE ( 'NONE', *, *, #18354, .T. ) ;
#10548=EDGE_CURVE ( 'NONE', #20032, #21598, #10645, .T. ) ;
#10549=ORIENTED_EDGE ( 'NONE', *, *, #28250, .T. ) ;
#10555=DIRECTION ( 'NONE',  ( 0.4528218681378510801, 0.8916010070295719014, -0.000000000000000000 ) ) ;
#10560=ORIENTED_EDGE ( 'NONE', *, *, #24363, .T. ) ;
#10563=DIRECTION ( 'NONE',  ( 0.000000000000000000, -1.000000000000000000, 0.000000000000000000 ) ) ;
#10568=LINE ( 'NONE', #3420, #7487 ) ;
#10571=( NAMED_UNIT ( * ) SI_UNIT ( $, .STERADIAN. ) SOLID_ANGLE_UNIT ( ) );
#10572=CARTESIAN_POINT ( 'NONE',  ( 158.0000000000003979, 170.8424998498591663, 45.00000000000000000 ) ) ;
#10573=ORIENTED_EDGE ( 'NONE', *, *, #22869, .T. ) ;
#10574=AXIS2_PLACEMENT_3D ( 'NONE', #6379, #20017, #19456 ) ;
#10576=VERTEX_POINT ( 'NONE', #15535 ) ;
#10581=CARTESIAN_POINT ( 'NONE',  ( 157.4999999999998579, 120.9389372034718093, 45.00000000000000000 ) ) ;
#10582=ORIENTED_EDGE ( 'NONE', *, *, #27601, .T. ) ;
#10583=VECTOR ( 'NONE', #22224, 1000.000000000000000 ) ;
#10584=ORIENTED_EDGE ( 'NONE', *, *, #7344, .F. ) ;
#10594=VECTOR ( 'NONE', #20947, 1000.000000000000114 ) ;
#10597=LINE ( 'NONE', #8303, #15218 ) ;
#10600=ORIENTED_EDGE ( 'NONE', *, *, #1797, .F. ) ;
#10604=CARTESIAN_POINT ( 'NONE',  ( 157.9999999999998295, 231.0315000300280417, -45.00000000000000000 ) ) ;
#10606=LINE ( 'NONE', #8310, #26214 ) ;
#10610=ORIENTED_EDGE ( 'NONE', *, *, #17205, .F. ) ;
#10614=VECTOR ( 'NONE', #26817, 1000.000000000000000 ) ;
#10615=ORIENTED_EDGE ( 'NONE', *, *, #16188, .F. ) ;
#10616=ORIENTED_EDGE ( 'NONE', *, *, #15714, .T. ) ;
#10617=ORIENTED_EDGE ( 'NONE', *, *, #21572, .T. ) ;
#10618=EDGE_CURVE ( 'NONE', #24084, #26943, #11938, .T. ) ;
#10620=EDGE_CURVE ( 'NONE', #23775, #20816, #15828, .T. ) ;
#10623=EDGE_CURVE ( 'NONE', #14862, #13449, #26866, .T. ) ;
#10624=DIRECTION ( 'NONE',  ( -0.8916010070296226386, 0.4528218681377511601, 0.000000000000000000 ) ) ;
#10625=CARTESIAN_POINT ( 'NONE',  ( 187.4999999999996305, 258.6181251126050711, 1.387778780781445676E-14 ) ) ;
#10627=CARTESIAN_POINT ( 'NONE',  ( 158.0000000000015632, 57.98812451204224061, 45.00000000000000000 ) ) ;
#10628=CARTESIAN_POINT ( 'NONE',  ( 157.4999999999996305, 286.4586876989355915, 45.00000000000000000 ) ) ;
#10633=LINE ( 'NONE', #15239, #6473 ) ;
#10634=PLANE ( 'NONE',  #8375 ) ;
#10635=VECTOR ( 'NONE', #26451, 1000.000000000000000 ) ;
#10637=AXIS2_PLACEMENT_3D ( 'NONE', #25065, #2320, #14860 ) ;
#10639=VECTOR ( 'NONE', #8561, 1000.000000000000227 ) ;
#10645=LINE ( 'NONE', #23862, #23971 ) ;
#10648=VERTEX_POINT ( 'NONE', #26716 ) ;
#10651=EDGE_CURVE ( 'NONE', #3632, #12751, #2727, .T. ) ;
#10652=VECTOR ( 'NONE', #14663, 1000.000000000000114 ) ;
#10658=DIRECTION ( 'NONE',  ( 0.4528218681382319422, -0.8916010070293783896, 0.000000000000000000 ) ) ;
#10661=CARTESIAN_POINT ( 'NONE',  ( 158.0000000000004263, 168.3346248423521274, 45.00000000000000000 ) ) ;
#10666=EDGE_CURVE ( 'NONE', #4885, #7590, #13960, .T. ) ;
#10668=CARTESIAN_POINT ( 'NONE',  ( 158.0000000000006537, 143.7637497747887210, 45.00000000000000000 ) ) ;
#10669=LINE ( 'NONE', #19429, #17625 ) ;
#10670=ORIENTED_EDGE ( 'NONE', *, *, #14579, .F. ) ;
#10671=VECTOR ( 'NONE', #837, 1000.000000000000114 ) ;
#10672=LINE ( 'NONE', #17698, #21519 ) ;
#10674=ADVANCED_FACE ( 'NONE', ( #727 ), #22706, .F. ) ;
#10677=LINE ( 'NONE', #21303, #14932 ) ;
#10680=VECTOR ( 'NONE', #12375, 1000.000000000000000 ) ;
#10681=ORIENTED_EDGE ( 'NONE', *, *, #13823, .F. ) ;
#10690=ORIENTED_EDGE ( 'NONE', *, *, #21641, .T. ) ;
#10691=ADVANCED_FACE ( 'NONE', ( #19770 ), #2238, .F. ) ;
#10692=ORIENTED_EDGE ( 'NONE', *, *, #18331, .T. ) ;
#10693=EDGE_LOOP ( 'NONE', ( #27937, #15789, #24498, #6402 ) ) ;
#10695=DIRECTION ( 'NONE',  ( 0.8916010070293510781, -0.4528218681382856770, 0.000000000000000000 ) ) ;
#10696=VECTOR ( 'NONE', #1755, 1000.000000000000227 ) ;
#10698=CARTESIAN_POINT ( 'NONE',  ( 158.0000000000017053, 45.44874947450702507, -45.00000000000000000 ) ) ;
#10699=CARTESIAN_POINT ( 'NONE',  ( 157.4999999999997726, 246.3326875788235384, 45.00000000000000000 ) ) ;
#10705=ORIENTED_EDGE ( 'NONE', *, *, #7863, .T. ) ;
#10708=DIRECTION ( 'NONE',  ( -0.000000000000000000, -0.000000000000000000, -1.000000000000000000 ) ) ;
#10710=CARTESIAN_POINT ( 'NONE',  ( 158.0000000000011653, 93.60624962464788723, -45.00000000000000000 ) ) ;
#10713=DIRECTION ( 'NONE',  ( 0.8916010070299470458, -0.4528218681371123377, 0.000000000000000000 ) ) ;
#10714=DIRECTION ( 'NONE',  ( -0.000000000000000000, -0.000000000000000000, -1.000000000000000000 ) ) ;
#10723=ORIENTED_EDGE ( 'NONE', *, *, #12618, .T. ) ;
#10724=CARTESIAN_POINT ( 'NONE',  ( 158.0000000000013358, 80.55899957960563995, 45.00000000000000000 ) ) ;
#10734=DIRECTION ( 'NONE',  ( 0.000000000000000000, -1.000000000000000000, 0.000000000000000000 ) ) ;
#10736=ADVANCED_FACE ( 'NONE', ( #20202 ), #13186, .F. ) ;
#10737=CARTESIAN_POINT ( 'NONE',  ( 157.9999999999999147, 213.9842499849850697, 45.00000000000000000 ) ) ;
#10750=CARTESIAN_POINT ( 'NONE',  ( 157.4999999999997442, 256.3641876088515232, -45.00000000000000000 ) ) ;
#10751=DIRECTION ( 'NONE',  ( -0.8916010070298157064, -0.4528218681373708532, 0.000000000000000000 ) ) ;
#10753=ORIENTED_EDGE ( 'NONE', *, *, #11531, .T. ) ;
#10754=EDGE_CURVE ( 'NONE', #2647, #17690, #11022, .T. ) ;
#10764=CARTESIAN_POINT ( 'NONE',  ( 158.0000000000006537, 141.2558747672816821, 45.00000000000000000 ) ) ;
#10767=PLANE ( 'NONE',  #3646 ) ;
#10768=DIRECTION ( 'NONE',  ( 0.8916010070293783896, -0.4528218681382319422, 0.000000000000000000 ) ) ;
#10770=LINE ( 'NONE', #16426, #25044 ) ;
#10779=DIRECTION ( 'NONE',  ( -0.000000000000000000, -0.000000000000000000, -1.000000000000000000 ) ) ;
#10780=DIRECTION ( 'NONE',  ( 0.4528218681389001854, 0.8916010070290391054, -0.000000000000000000 ) ) ;
#10785=CARTESIAN_POINT ( 'NONE',  ( 157.4999999999996305, 283.9508126914284958, 45.00000000000000000 ) ) ;
#10790=ORIENTED_EDGE ( 'NONE', *, *, #13135, .T. ) ;
#10792=PLANE ( 'NONE',  #28265 ) ;
#10794=VECTOR ( 'NONE', #8257, 1000.000000000000227 ) ;
#10798=CARTESIAN_POINT ( 'NONE',  ( 158.0000000000001990, 188.3976249024084666, 45.00000000000000000 ) ) ;
#10802=ORIENTED_EDGE ( 'NONE', *, *, #15962, .T. ) ;
#10806=DIRECTION ( 'NONE',  ( 0.4528218681373320509, 0.8916010070298354684, -0.000000000000000000 ) ) ;
#10807=DIRECTION ( 'NONE',  ( -0.000000000000000000, -0.000000000000000000, -1.000000000000000000 ) ) ;
#10813=CARTESIAN_POINT ( 'NONE',  ( 158.0000000000010516, 103.6377496546760568, -45.00000000000000000 ) ) ;
#10814=VECTOR ( 'NONE', #1370, 1000.000000000000000 ) ;
#10816=CARTESIAN_POINT ( 'NONE',  ( 157.4999999999998579, 118.4310621959647563, 45.00000000000000000 ) ) ;
#10819=CARTESIAN_POINT ( 'NONE',  ( 158.0000000000013642, 76.05112457209858690, 45.00000000000000000 ) ) ;
#10822=VECTOR ( 'NONE', #19874, 1000.000000000000000 ) ;
#10823=ORIENTED_EDGE ( 'NONE', *, *, #14517, .F. ) ;
#10824=CARTESIAN_POINT ( 'NONE',  ( 157.9999999999998010, 241.0630000600560550, 45.00000000000000000 ) ) ;
#10826=ORIENTED_EDGE ( 'NONE', *, *, #19830, .F. ) ;
#10827=EDGE_LOOP ( 'NONE', ( #16384, #24176, #992, #9099 ) ) ;
#10828=DIRECTION ( 'NONE',  ( -0.8916010070293384215, 0.4528218681383106015, 0.000000000000000000 ) ) ;
#10829=CARTESIAN_POINT ( 'NONE',  ( 158.0000000000007390, 135.7322497447605656, -45.00000000000000000 ) ) ;
#10832=ORIENTED_EDGE ( 'NONE', *, *, #23458, .T. ) ;
#10833=VECTOR ( 'NONE', #13451, 999.9999999999998863 ) ;
#10836=DIRECTION ( 'NONE',  ( -0.000000000000000000, -0.000000000000000000, -1.000000000000000000 ) ) ;
#10838=LINE ( 'NONE', #200, #10342 ) ;
#10841=CARTESIAN_POINT ( 'NONE',  ( 158.0000000000011369, 96.11412463215494029, -45.00000000000000000 ) ) ;
#10843=ORIENTED_EDGE ( 'NONE', *, *, #19407, .F. ) ;
#10845=EDGE_CURVE ( 'NONE', #11955, #8565, #14044, .T. ) ;
#10849=ORIENTED_EDGE ( 'NONE', *, *, #2655, .T. ) ;
#10851=FACE_OUTER_BOUND ( 'NONE', #19900, .T. ) ;
#10853=ADVANCED_FACE ( 'NONE', ( #813 ), #18751, .F. ) ;
#10854=LINE ( 'NONE', #1933, #23985 ) ;
#10856=CARTESIAN_POINT ( 'NONE',  ( 158.0000000000011084, 98.62199963966197913, 45.00000000000000000 ) ) ;
#10864=VERTEX_POINT ( 'NONE', #20629 ) ;
#10867=LINE ( 'NONE', #21782, #300 ) ;
#10874=FACE_OUTER_BOUND ( 'NONE', #21859, .T. ) ;
#10876=EDGE_CURVE ( 'NONE', #5381, #6186, #23210, .T. ) ;
#10879=EDGE_CURVE ( 'NONE', #16770, #5280, #27228, .T. ) ;
#10888=FACE_OUTER_BOUND ( 'NONE', #26318, .T. ) ;
#10896=ORIENTED_EDGE ( 'NONE', *, *, #18498, .T. ) ;
#10898=ORIENTED_EDGE ( 'NONE', *, *, #27498, .T. ) ;
#10899=AXIS2_PLACEMENT_3D ( 'NONE', #9745, #16220, #14067 ) ;
#10900=ORIENTED_EDGE ( 'NONE', *, *, #7515, .F. ) ;
#10904=DIRECTION ( 'NONE',  ( 0.4528218681382713551, 0.8916010070293584056, -0.000000000000000000 ) ) ;
#10908=CARTESIAN_POINT ( 'NONE',  ( 157.4999999999998295, 226.2696875187675118, 45.00000000000000000 ) ) ;
#10913=LINE ( 'NONE', #24264, #237 ) ;
#10914=LINE ( 'NONE', #6508, #2659 ) ;
#10919=ORIENTED_EDGE ( 'NONE', *, *, #10618, .T. ) ;
#10920=ORIENTED_EDGE ( 'NONE', *, *, #20149, .T. ) ;
#10924=LINE ( 'NONE', #4310, #19060 ) ;
#10929=VERTEX_POINT ( 'NONE', #16605 ) ;
#10930=AXIS2_PLACEMENT_3D ( 'NONE', #20835, #18678, #27425 ) ;
#10931=DIRECTION ( 'NONE',  ( 0.4528218681374919785, 0.8916010070297542001, -0.000000000000000000 ) ) ;
#10933=VECTOR ( 'NONE', #172, 1000.000000000000227 ) ;
#10934=ORIENTED_EDGE ( 'NONE', *, *, #27526, .T. ) ;
#10935=EDGE_CURVE ( 'NONE', #9674, #16172, #14455, .T. ) ;
#10937=ADVANCED_FACE ( 'NONE', ( #24804 ), #13905, .F. ) ;
#10940=ORIENTED_EDGE ( 'NONE', *, *, #28105, .T. ) ;
#10945=CARTESIAN_POINT ( 'NONE',  ( 157.4999999999996874, 271.4114376538935289, -45.00000000000000000 ) ) ;
#10955=ADVANCED_FACE ( 'NONE', ( #18480 ), #7569, .F. ) ;
#10956=EDGE_CURVE ( 'NONE', #17690, #15187, #3234, .T. ) ;
#10957=CARTESIAN_POINT ( 'NONE',  ( 158.0000000000009663, 113.1613746771971876, 45.00000000000000000 ) ) ;
#10962=DIRECTION ( 'NONE',  ( -0.8916010070293409751, -0.4528218681383056610, 0.000000000000000000 ) ) ;
#10967=ORIENTED_EDGE ( 'NONE', *, *, #22948, .F. ) ;
#10971=CARTESIAN_POINT ( 'NONE',  ( 157.9999999999998010, 233.5393750375350237, -45.00000000000000000 ) ) ;
#10976=VECTOR ( 'NONE', #17970, 1000.000000000000000 ) ;
#10977=EDGE_CURVE ( 'NONE', #17587, #18428, #20689, .T. ) ;
#10979=EDGE_CURVE ( 'NONE', #27519, #2485, #10067, .T. ) ;
#10982=CARTESIAN_POINT ( 'NONE',  ( 157.4999999999998579, 143.5098122710352015, -45.00000000000000000 ) ) ;
#10983=CARTESIAN_POINT ( 'NONE',  ( 157.4999999999996305, 283.9508126914284958, -45.00000000000000000 ) ) ;
#10984=DIRECTION ( 'NONE',  ( 0.4528218681383305855, -0.8916010070293283185, 0.000000000000000000 ) ) ;
#10988=VECTOR ( 'NONE', #23514, 1000.000000000000114 ) ;
#10989=PLANE ( 'NONE',  #26228 ) ;
#10990=CARTESIAN_POINT ( 'NONE',  ( 158.0000000000009095, 120.6849996997183183, 45.00000000000000000 ) ) ;
#10992=ORIENTED_EDGE ( 'NONE', *, *, #1668, .T. ) ;
#10994=VECTOR ( 'NONE', #11650, 1000.000000000000000 ) ;
#10995=ORIENTED_EDGE ( 'NONE', *, *, #18247, .T. ) ;
#10999=LINE ( 'NONE', #13164, #23021 ) ;
#11005=ORIENTED_EDGE ( 'NONE', *, *, #18565, .T. ) ;
#11008=ORIENTED_EDGE ( 'NONE', *, *, #24681, .T. ) ;
#11009=CARTESIAN_POINT ( 'NONE',  ( 158.0000000000014779, 63.51174953456337136, 45.00000000000000000 ) ) ;
#11010=VECTOR ( 'NONE', #2233, 1000.000000000000114 ) ;
#11017=EDGE_CURVE ( 'NONE', #5089, #12678, #25426, .T. ) ;
#11020=FACE_OUTER_BOUND ( 'NONE', #17077, .T. ) ;
#11021=CARTESIAN_POINT ( 'NONE',  ( 158.0000000000003695, 173.3503748573662051, 45.00000000000000000 ) ) ;
#11022=LINE ( 'NONE', #22073, #23047 ) ;
#11023=DIRECTION ( 'NONE',  ( -0.000000000000000000, 0.000000000000000000, -1.000000000000000000 ) ) ;
#11025=LINE ( 'NONE', #21933, #22555 ) ;
#11027=CARTESIAN_POINT ( 'NONE',  ( 158.0000000000000000, 206.4606249624626457, 45.00000000000000000 ) ) ;
#11030=VECTOR ( 'NONE', #23806, 1000.000000000000000 ) ;
#11032=CARTESIAN_POINT ( 'NONE',  ( 157.9999999999998010, 239.0630000600560550, 45.00000000000000000 ) ) ;
#11035=AXIS2_PLACEMENT_3D ( 'NONE', #21302, #8377, #28033 ) ;
#11039=VERTEX_POINT ( 'NONE', #20836 ) ;
#11040=ORIENTED_EDGE ( 'NONE', *, *, #3205, .T. ) ;
#11043=ORIENTED_EDGE ( 'NONE', *, *, #25133, .F. ) ;
#11045=EDGE_CURVE ( 'NONE', #26706, #19122, #18964, .T. ) ;
#11048=DIRECTION ( 'NONE',  ( 0.8916010070297948342, -0.4528218681374120425, 0.000000000000000000 ) ) ;
#11052=LINE ( 'NONE', #23983, #6449 ) ;
#11053=CARTESIAN_POINT ( 'NONE',  ( 158.0000000000007674, 131.2243747372535267, 45.00000000000000000 ) ) ;
#11055=CARTESIAN_POINT ( 'NONE',  ( 157.4999999999996874, 266.3956876388795649, 45.00000000000000000 ) ) ;
#11061=CARTESIAN_POINT ( 'NONE',  ( 157.9999999999996874, 264.1417501351260171, -45.00000000000000000 ) ) ;
#11064=ORIENTED_EDGE ( 'NONE', *, *, #14326, .F. ) ;
#11072=AXIS2_PLACEMENT_3D ( 'NONE', #25015, #1299, #24874 ) ;
#11074=PLANE ( 'NONE',  #2399 ) ;
#11076=VERTEX_POINT ( 'NONE', #12794 ) ;
#11079=CARTESIAN_POINT ( 'NONE',  ( 157.4999999999995168, 208.7145624662163925, -45.00000000000000000 ) ) ;
#11089=EDGE_LOOP ( 'NONE', ( #26182, #22530, #14614, #13601 ) ) ;
#11092=DIRECTION ( 'NONE',  ( 1.000000000000000000, 0.000000000000000000, -0.000000000000000000 ) ) ;
#11095=EDGE_CURVE ( 'NONE', #24747, #9674, #26412, .T. ) ;
#11102=VECTOR ( 'NONE', #8970, 1000.000000000000114 ) ;
#11105=ORIENTED_EDGE ( 'NONE', *, *, #19305, .T. ) ;
#11108=DIRECTION ( 'NONE',  ( 0.8916010070296226386, -0.4528218681377511046, 0.000000000000000000 ) ) ;
#11111=VERTEX_POINT ( 'NONE', #21687 ) ;
#11114=ADVANCED_FACE ( 'NONE', ( #137 ), #8331, .F. ) ;
#11117=LINE ( 'NONE', #7091, #23122 ) ;
#11118=CARTESIAN_POINT ( 'NONE',  ( 157.9999999999999432, 213.4763749774776045, 45.00000000000000000 ) ) ;
#11123=ORIENTED_EDGE ( 'NONE', *, *, #2124, .T. ) ;
#11124=VECTOR ( 'NONE', #22437, 999.9999999999998863 ) ;
#11132=DIRECTION ( 'NONE',  ( 0.8916010070299166257, -0.4528218681371722343, 0.000000000000000000 ) ) ;
#11143=ORIENTED_EDGE ( 'NONE', *, *, #21385, .F. ) ;
#11152=ORIENTED_EDGE ( 'NONE', *, *, #20508, .F. ) ;
#11159=CARTESIAN_POINT ( 'NONE',  ( 157.4999999999994884, 211.2224374737238577, 45.00000000000000000 ) ) ;
#11160=CARTESIAN_POINT ( 'NONE',  ( 187.4999999999996305, 40.68693696324645970, -45.00000000000000000 ) ) ;
#11162=DIRECTION ( 'NONE',  ( -0.000000000000000000, 0.000000000000000000, -1.000000000000000000 ) ) ;
#11164=DIRECTION ( 'NONE',  ( 1.000000000000000000, 0.000000000000000000, -0.000000000000000000 ) ) ;
#11176=VERTEX_POINT ( 'NONE', #11351 ) ;
#11182=ORIENTED_EDGE ( 'NONE', *, *, #4388, .F. ) ;
#11183=EDGE_LOOP ( 'NONE', ( #21006, #1938, #7970, #8738 ) ) ;
#11193=LINE ( 'NONE', #15226, #19912 ) ;
#11196=CARTESIAN_POINT ( 'NONE',  ( 158.0000000000011937, 93.09837461714084839, 45.00000000000000000 ) ) ;
#11201=CARTESIAN_POINT ( 'NONE',  ( 157.9999999999997158, 261.6338751276190351, -45.00000000000000000 ) ) ;
#11203=DIRECTION ( 'NONE',  ( -0.000000000000000000, -0.000000000000000000, -1.000000000000000000 ) ) ;
#11205=CARTESIAN_POINT ( 'NONE',  ( 158.0000000000009948, 108.6534996696901345, 45.00000000000000000 ) ) ;
#11207=ORIENTED_EDGE ( 'NONE', *, *, #8217, .T. ) ;
#11211=EDGE_CURVE ( 'NONE', #3398, #16038, #13651, .T. ) ;
#11214=DIRECTION ( 'NONE',  ( -0.000000000000000000, 0.000000000000000000, -1.000000000000000000 ) ) ;
#11218=AXIS2_PLACEMENT_3D ( 'NONE', #6770, #15276, #13259 ) ;
#11219=ORIENTED_EDGE ( 'NONE', *, *, #11972, .F. ) ;
#11226=LINE ( 'NONE', #17679, #9593 ) ;
#11232=CARTESIAN_POINT ( 'NONE',  ( 157.4999999999997158, 263.8878126313725829, -45.00000000000000000 ) ) ;
#11237=EDGE_LOOP ( 'NONE', ( #3980, #24149, #22528, #18771 ) ) ;
#11238=DIRECTION ( 'NONE',  ( -0.8916010070297948342, 0.4528218681374120425, 0.000000000000000000 ) ) ;
#11239=EDGE_CURVE ( 'NONE', #14420, #26421, #15662, .T. ) ;
#11241=CARTESIAN_POINT ( 'NONE',  ( 157.4999999999998579, 163.5728123310915407, 45.00000000000000000 ) ) ;
#11242=CARTESIAN_POINT ( 'NONE',  ( 157.4999999999998579, 63.25781203080982351, 45.00000000000000000 ) ) ;
#11244=LINE ( 'NONE', #6351, #24268 ) ;
#11255=CARTESIAN_POINT ( 'NONE',  ( 157.9999999999996589, 276.1732501651540588, -45.00000000000000000 ) ) ;
#11256=DIRECTION ( 'NONE',  ( 0.000000000000000000, -1.000000000000000000, 0.000000000000000000 ) ) ;
#11257=ORIENTED_EDGE ( 'NONE', *, *, #15670, .T. ) ;
#11261=DIRECTION ( 'NONE',  ( 0.4528218681369723941, 0.8916010070300182111, -0.000000000000000000 ) ) ;
#11265=CARTESIAN_POINT ( 'NONE',  ( 157.4999999999998579, 156.0491873085704242, 45.00000000000000000 ) ) ;
#11274=EDGE_CURVE ( 'NONE', #18947, #26586, #10037, .T. ) ;
#11275=EDGE_CURVE ( 'NONE', #7481, #16156, #16372, .T. ) ;
#11277=DIRECTION ( 'NONE',  ( -0.000000000000000000, 0.000000000000000000, -1.000000000000000000 ) ) ;
#11279=LINE ( 'NONE', #17584, #8332 ) ;
#11280=PLANE ( 'NONE',  #7307 ) ;
#11281=CARTESIAN_POINT ( 'NONE',  ( 157.4999999999998579, 135.9861872485140850, 45.00000000000000000 ) ) ;
#11282=VERTEX_POINT ( 'NONE', #5856 ) ;
#11283=DIRECTION ( 'NONE',  ( -0.000000000000000000, 0.000000000000000000, -1.000000000000000000 ) ) ;
#11286=CARTESIAN_POINT ( 'NONE',  ( 157.4999999999998295, 218.7460624962465090, 45.00000000000000000 ) ) ;
#11289=CARTESIAN_POINT ( 'NONE',  ( 157.4999999999998579, 125.9546872184859012, 45.00000000000000000 ) ) ;
#11290=EDGE_LOOP ( 'NONE', ( #26832, #10373, #22950, #12108 ) ) ;
#11295=LINE ( 'NONE', #16036, #26873 ) ;
#11300=CARTESIAN_POINT ( 'NONE',  ( 157.4999999999997726, 243.8248125713165280, 45.00000000000000000 ) ) ;
#11304=ORIENTED_EDGE ( 'NONE', *, *, #6743, .T. ) ;
#11305=EDGE_CURVE ( 'NONE', #24279, #26566, #8159, .T. ) ;
#11309=FACE_OUTER_BOUND ( 'NONE', #11183, .T. ) ;
#11311=CARTESIAN_POINT ( 'NONE',  ( 157.4999999999998579, 128.4625622259929401, 45.00000000000000000 ) ) ;
#11313=CARTESIAN_POINT ( 'NONE',  ( 157.9999999999997442, 251.6023750975910218, -45.00000000000000000 ) ) ;
#11314=CARTESIAN_POINT ( 'NONE',  ( 158.0000000000006253, 146.2716247822957598, 45.00000000000000000 ) ) ;
#11317=CARTESIAN_POINT ( 'NONE',  ( 158.0000000000016485, 50.46449948952111697, -45.00000000000000000 ) ) ;
#11318=VECTOR ( 'NONE', #1592, 1000.000000000000227 ) ;
#11324=VECTOR ( 'NONE', #14314, 1000.000000000000000 ) ;
#11325=ORIENTED_EDGE ( 'NONE', *, *, #19437, .T. ) ;
#11326=EDGE_CURVE ( 'NONE', #1637, #9971, #27266, .T. ) ;
#11331=ORIENTED_EDGE ( 'NONE', *, *, #19086, .T. ) ;
#11334=VERTEX_POINT ( 'NONE', #23250 ) ;
#11336=VECTOR ( 'NONE', #14032, 1000.000000000000114 ) ;
#11337=DIRECTION ( 'NONE',  ( -0.8916010070293510781, 0.4528218681382856214, 0.000000000000000000 ) ) ;
#11339=DIRECTION ( 'NONE',  ( -0.000000000000000000, 0.000000000000000000, -1.000000000000000000 ) ) ;
#11344=LINE ( 'NONE', #4713, #15273 ) ;
#11346=CARTESIAN_POINT ( 'NONE',  ( 158.0000000000014211, 70.52749954957745615, 45.00000000000000000 ) ) ;
#11351=CARTESIAN_POINT ( 'NONE',  ( 157.4999999999998579, 133.4783122410070462, -45.00000000000000000 ) ) ;
#11352=DIRECTION ( 'NONE',  ( 0.8916010070299267287, -0.4528218681371523058, 0.000000000000000000 ) ) ;
#11353=DIRECTION ( 'NONE',  ( 0.8916010070293383105, -0.4528218681383106015, 0.000000000000000000 ) ) ;
#11359=CARTESIAN_POINT ( 'NONE',  ( 157.4999999999998579, 95.86018712840139244, 45.00000000000000000 ) ) ;
#11364=VERTEX_POINT ( 'NONE', #20949 ) ;
#11370=CARTESIAN_POINT ( 'NONE',  ( 157.4999999999998579, 223.7618125112605298, 45.00000000000000000 ) ) ;
#11373=ORIENTED_EDGE ( 'NONE', *, *, #19137, .T. ) ;
#11378=EDGE_CURVE ( 'NONE', #17634, #10196, #12063, .T. ) ;
#11381=CARTESIAN_POINT ( 'NONE',  ( 158.0000000000017337, 40.94087446699997912, 45.00000000000000000 ) ) ;
#11384=DIRECTION ( 'NONE',  ( -0.000000000000000000, -0.000000000000000000, -1.000000000000000000 ) ) ;
#11388=VERTEX_POINT ( 'NONE', #25402 ) ;
#11390=VECTOR ( 'NONE', #18237, 1000.000000000000000 ) ;
#11393=CARTESIAN_POINT ( 'NONE',  ( 157.9999999999996874, 266.6496251426330559, 45.00000000000000000 ) ) ;
#11394=ORIENTED_EDGE ( 'NONE', *, *, #8102, .F. ) ;
#11400=ORIENTED_EDGE ( 'NONE', *, *, #17090, .T. ) ;
#11403=EDGE_CURVE ( 'NONE', #22271, #21564, #4267, .T. ) ;
#11414=CARTESIAN_POINT ( 'NONE',  ( 158.0000000000011653, 93.60624962464788723, 45.00000000000000000 ) ) ;
#11418=CARTESIAN_POINT ( 'NONE',  ( 157.4999999999998579, 138.4940622560211239, -45.00000000000000000 ) ) ;
#11421=ORIENTED_EDGE ( 'NONE', *, *, #20673, .T. ) ;
#11428=VERTEX_POINT ( 'NONE', #15202 ) ;
#11433=ORIENTED_EDGE ( 'NONE', *, *, #4245, .F. ) ;
#11435=LINE ( 'NONE', #21911, #28070 ) ;
#11436=ORIENTED_EDGE ( 'NONE', *, *, #25957, .T. ) ;
#11437=VECTOR ( 'NONE', #17095, 1000.000000000000000 ) ;
#11442=VERTEX_POINT ( 'NONE', #23816 ) ;
#11445=LINE ( 'NONE', #27216, #16383 ) ;
#11447=VECTOR ( 'NONE', #22891, 1000.000000000000000 ) ;
#11454=CARTESIAN_POINT ( 'NONE',  ( 157.9999999999997726, 246.5866250825770294, 45.00000000000000000 ) ) ;
#11461=EDGE_CURVE ( 'NONE', #23433, #13313, #25677, .T. ) ;
#11464=CARTESIAN_POINT ( 'NONE',  ( 157.9999999999996874, 266.1417501351260171, 45.00000000000000000 ) ) ;
#11467=ORIENTED_EDGE ( 'NONE', *, *, #24668, .T. ) ;
#11469=PLANE ( 'NONE',  #6415 ) ;
#11470=CARTESIAN_POINT ( 'NONE',  ( 157.4999999999995453, 206.2066874587088989, 45.00000000000000000 ) ) ;
#11473=EDGE_CURVE ( 'NONE', #16305, #13433, #8725, .T. ) ;
#11474=AXIS2_PLACEMENT_3D ( 'NONE', #1023, #11541, #7640 ) ;
#11476=VERTEX_POINT ( 'NONE', #6147 ) ;
#11477=DIRECTION ( 'NONE',  ( -0.000000000000000000, -0.000000000000000000, -1.000000000000000000 ) ) ;
#11478=ORIENTED_EDGE ( 'NONE', *, *, #670, .T. ) ;
#11483=ORIENTED_EDGE ( 'NONE', *, *, #25881, .F. ) ;
#11485=CARTESIAN_POINT ( 'NONE',  ( 157.4999999999995168, 208.7145624662163925, 45.00000000000000000 ) ) ;
#11486=DIRECTION ( 'NONE',  ( 0.000000000000000000, -1.000000000000000000, 0.000000000000000000 ) ) ;
#11491=LINE ( 'NONE', #15806, #23979 ) ;
#11492=CARTESIAN_POINT ( 'NONE',  ( 157.9999999999996305, 286.7126252026890256, 45.00000000000000000 ) ) ;
#11493=EDGE_CURVE ( 'NONE', #749, #12783, #4405, .T. ) ;
#11495=CARTESIAN_POINT ( 'NONE',  ( 157.4999999999998579, 166.0806873385985796, -45.00000000000000000 ) ) ;
#11497=FACE_OUTER_BOUND ( 'NONE', #12438, .T. ) ;
#11507=ORIENTED_EDGE ( 'NONE', *, *, #25656, .F. ) ;
#11508=EDGE_CURVE ( 'NONE', #27514, #13811, #2244, .T. ) ;
#11509=DIRECTION ( 'NONE',  ( 0.4528218681371711241, -0.8916010070299172918, 0.000000000000000000 ) ) ;
#11511=ORIENTED_EDGE ( 'NONE', *, *, #6623, .F. ) ;
#11513=EDGE_CURVE ( 'NONE', #22677, #6513, #16921, .T. ) ;
#11516=DIRECTION ( 'NONE',  ( -0.8916010070293283185, -0.4528218681383305855, 0.000000000000000000 ) ) ;
#11520=EDGE_CURVE ( 'NONE', #1215, #9638, #14920, .T. ) ;
#11523=FACE_OUTER_BOUND ( 'NONE', #16690, .T. ) ;
#11526=VERTEX_POINT ( 'NONE', #8449 ) ;
#11528=CARTESIAN_POINT ( 'NONE',  ( 157.4999999999998295, 231.2854375337815327, -45.00000000000000000 ) ) ;
#11530=CARTESIAN_POINT ( 'NONE',  ( 157.9999999999998295, 228.5236250225210313, 45.00000000000000000 ) ) ;
#11531=EDGE_CURVE ( 'NONE', #27897, #27519, #12909, .T. ) ;
#11534=ORIENTED_EDGE ( 'NONE', *, *, #1441, .F. ) ;
#11536=CARTESIAN_POINT ( 'NONE',  ( 158.0000000000014211, 73.03537455708450921, 45.00000000000000000 ) ) ;
#11540=ORIENTED_EDGE ( 'NONE', *, *, #17869, .F. ) ;
#11541=DIRECTION ( 'NONE',  ( 1.000000000000000000, 0.000000000000000000, -0.000000000000000000 ) ) ;
#11547=EDGE_CURVE ( 'NONE', #17151, #24242, #2526, .T. ) ;
#11551=VERTEX_POINT ( 'NONE', #4970 ) ;
#11552=ORIENTED_EDGE ( 'NONE', *, *, #16340, .F. ) ;
#11555=CARTESIAN_POINT ( 'NONE',  ( 158.0000000000005684, 153.2873747973098659, -45.00000000000000000 ) ) ;
#11556=ORIENTED_EDGE ( 'NONE', *, *, #2518, .T. ) ;
#11557=DIRECTION ( 'NONE',  ( -0.8916010070296124246, -0.4528218681377710886, 0.000000000000000000 ) ) ;
#11562=CARTESIAN_POINT ( 'NONE',  ( 158.0000000000001137, 195.9212499249295831, 45.00000000000000000 ) ) ;
#11563=LINE ( 'NONE', #21889, #17616 ) ;
#11566=LINE ( 'NONE', #25182, #11447 ) ;
#11568=EDGE_CURVE ( 'NONE', #1420, #11388, #534, .T. ) ;
#11569=DIRECTION ( 'NONE',  ( -0.8916010070295616874, -0.4528218681378710642, 0.000000000000000000 ) ) ;
#11570=CARTESIAN_POINT ( 'NONE',  ( 158.0000000000003979, 170.8424998498591663, -45.00000000000000000 ) ) ;
#11571=LINE ( 'NONE', #20312, #13273 ) ;
#11575=ORIENTED_EDGE ( 'NONE', *, *, #10351, .F. ) ;
#11585=VERTEX_POINT ( 'NONE', #13617 ) ;
#11587=EDGE_CURVE ( 'NONE', #11476, #21473, #20059, .T. ) ;
#11592=PLANE ( 'NONE',  #7622 ) ;
#11593=ORIENTED_EDGE ( 'NONE', *, *, #7675, .T. ) ;
#11594=ORIENTED_EDGE ( 'NONE', *, *, #17975, .T. ) ;
#11596=ORIENTED_EDGE ( 'NONE', *, *, #3390, .F. ) ;
#11597=ORIENTED_EDGE ( 'NONE', *, *, #4290, .F. ) ;
#11603=VECTOR ( 'NONE', #5171, 1000.000000000000000 ) ;
#11604=AXIS2_PLACEMENT_3D ( 'NONE', #2394, #2685, #13478 ) ;
#11605=DIRECTION ( 'NONE',  ( 0.000000000000000000, -1.000000000000000000, 0.000000000000000000 ) ) ;
#11606=DIRECTION ( 'NONE',  ( 0.8916010070293409751, 0.4528218681383056610, 0.000000000000000000 ) ) ;
#11611=DIRECTION ( 'NONE',  ( 0.8916010070293710621, -0.4528218681382463195, 0.000000000000000000 ) ) ;
#11613=ORIENTED_EDGE ( 'NONE', *, *, #24459, .T. ) ;
#11619=CARTESIAN_POINT ( 'NONE',  ( 158.0000000000010516, 105.6377496546760568, -45.00000000000000000 ) ) ;
#11621=VECTOR ( 'NONE', #12214, 1000.000000000000114 ) ;
#11624=EDGE_CURVE ( 'NONE', #16770, #689, #22513, .T. ) ;
#11626=ORIENTED_EDGE ( 'NONE', *, *, #5112, .T. ) ;
#11627=VECTOR ( 'NONE', #10012, 1000.000000000000114 ) ;
#11633=DIRECTION ( 'NONE',  ( 0.4528218681382856770, 0.8916010070293511891, -0.000000000000000000 ) ) ;
#11634=CARTESIAN_POINT ( 'NONE',  ( 157.9999999999996589, 281.1890001801680796, 45.00000000000000000 ) ) ;
#11635=DIRECTION ( 'NONE',  ( -0.8916010070295715684, 0.4528218681378515797, 0.000000000000000000 ) ) ;
#11636=FACE_OUTER_BOUND ( 'NONE', #13953, .T. ) ;
#11644=VECTOR ( 'NONE', #8865, 1000.000000000000227 ) ;
#11650=DIRECTION ( 'NONE',  ( -0.000000000000000000, -0.000000000000000000, -1.000000000000000000 ) ) ;
#11651=DIRECTION ( 'NONE',  ( -0.000000000000000000, -0.000000000000000000, -1.000000000000000000 ) ) ;
#11656=DIRECTION ( 'NONE',  ( 1.000000000000000000, 0.000000000000000000, -0.000000000000000000 ) ) ;
#11658=AXIS2_PLACEMENT_3D ( 'NONE', #8326, #1845, #10624 ) ;
#11659=ORIENTED_EDGE ( 'NONE', *, *, #11868, .T. ) ;
#11660=EDGE_CURVE ( 'NONE', #1387, #27519, #20351, .T. ) ;
#11665=EDGE_LOOP ( 'NONE', ( #26967, #16905, #25977, #8842 ) ) ;
#11666=VECTOR ( 'NONE', #17444, 1000.000000000000114 ) ;
#11669=CARTESIAN_POINT ( 'NONE',  ( 158.0000000000005400, 155.7952498048169048, 45.00000000000000000 ) ) ;
#11673=DIRECTION ( 'NONE',  ( 0.000000000000000000, -1.000000000000000000, 0.000000000000000000 ) ) ;
#11675=EDGE_CURVE ( 'NONE', #25368, #800, #391, .T. ) ;
#11677=DIRECTION ( 'NONE',  ( 0.4528218681375119625, 0.8916010070297440970, -0.000000000000000000 ) ) ;
#11681=CARTESIAN_POINT ( 'NONE',  ( 158.0000000000003979, 170.8424998498591663, 45.00000000000000000 ) ) ;
#11685=DIRECTION ( 'NONE',  ( 0.000000000000000000, 0.000000000000000000, -1.000000000000000000 ) ) ;
#11689=ORIENTED_EDGE ( 'NONE', *, *, #17253, .T. ) ;
#11693=VECTOR ( 'NONE', #11841, 1000.000000000000000 ) ;
#11694=VERTEX_POINT ( 'NONE', #18207 ) ;
#11695=LINE ( 'NONE', #22452, #26014 ) ;
#11698=VERTEX_POINT ( 'NONE', #15918 ) ;
#11706=FACE_OUTER_BOUND ( 'NONE', #12045, .T. ) ;
#11709=DIRECTION ( 'NONE',  ( 0.000000000000000000, -1.000000000000000000, 0.000000000000000000 ) ) ;
#11714=LINE ( 'NONE', #11570, #24386 ) ;
#11717=ORIENTED_EDGE ( 'NONE', *, *, #22068, .T. ) ;
#11719=LINE ( 'NONE', #7396, #27919 ) ;
#11720=EDGE_LOOP ( 'NONE', ( #12532, #22676, #8932, #20605 ) ) ;
#11725=LINE ( 'NONE', #27209, #4182 ) ;
#11729=LINE ( 'NONE', #7261, #12497 ) ;
#11730=LINE ( 'NONE', #16176, #13597 ) ;
#11737=ORIENTED_EDGE ( 'NONE', *, *, #8314, .T. ) ;
#11739=VECTOR ( 'NONE', #4119, 1000.000000000000000 ) ;
#11744=AXIS2_PLACEMENT_3D ( 'NONE', #17294, #10555, #15157 ) ;
#11745=ADVANCED_FACE ( 'NONE', ( #9724 ), #12171, .F. ) ;
#11747=CARTESIAN_POINT ( 'NONE',  ( 157.4999999999998010, 238.8090625563025071, 45.00000000000000000 ) ) ;
#11748=FACE_OUTER_BOUND ( 'NONE', #27604, .T. ) ;
#11752=LINE ( 'NONE', #22655, #26852 ) ;
#11755=CARTESIAN_POINT ( 'NONE',  ( 157.9999999999998295, 224.0157500150140208, 45.00000000000000000 ) ) ;
#11763=LINE ( 'NONE', #18631, #8402 ) ;
#11764=EDGE_LOOP ( 'NONE', ( #17730, #14685, #7512, #3877 ) ) ;
#11767=VERTEX_POINT ( 'NONE', #3381 ) ;
#11772=LINE ( 'NONE', #27525, #20304 ) ;
#11776=UNCERTAINTY_MEASURE_WITH_UNIT (LENGTH_MEASURE( 1.000000000000000082E-05 ), #25645, 'distance_accuracy_value', 'NONE');
#11777=VECTOR ( 'NONE', #8431, 1000.000000000000000 ) ;
#11779=CARTESIAN_POINT ( 'NONE',  ( 158.0000000000013927, 75.54324956459154805, 45.00000000000000000 ) ) ;
#11785=VECTOR ( 'NONE', #5685, 1000.000000000000000 ) ;
#11786=CARTESIAN_POINT ( 'NONE',  ( 158.0000000000000853, 198.9369999399436892, -45.00000000000000000 ) ) ;
#11792=LINE ( 'NONE', #22550, #1502 ) ;
#11799=ORIENTED_EDGE ( 'NONE', *, *, #27223, .T. ) ;
#11800=DIRECTION ( 'NONE',  ( 1.000000000000000000, 0.000000000000000000, -0.000000000000000000 ) ) ;
#11801=LINE ( 'NONE', #9637, #22778 ) ;
#11802=ORIENTED_EDGE ( 'NONE', *, *, #2440, .T. ) ;
#11804=DIRECTION ( 'NONE',  ( 0.8916010070297749612, 0.4528218681374510668, 0.000000000000000000 ) ) ;
#11806=EDGE_CURVE ( 'NONE', #2305, #12610, #954, .T. ) ;
#11807=CARTESIAN_POINT ( 'NONE',  ( 157.4999999999998579, 60.74993702330277756, 45.00000000000000000 ) ) ;
#11815=CARTESIAN_POINT ( 'NONE',  ( 158.0000000000007674, 133.2243747372535267, 45.00000000000000000 ) ) ;
#11817=PLANE ( 'NONE',  #17085 ) ;
#11818=DIRECTION ( 'NONE',  ( 1.000000000000000000, 0.000000000000000000, -0.000000000000000000 ) ) ;
#11825=ORIENTED_EDGE ( 'NONE', *, *, #2690, .T. ) ;
#11826=ADVANCED_FACE ( 'NONE', ( #3662 ), #25087, .F. ) ;
#11830=ORIENTED_EDGE ( 'NONE', *, *, #23855, .F. ) ;
#11832=EDGE_LOOP ( 'NONE', ( #5173, #21341, #24786, #26354 ) ) ;
#11834=LINE ( 'NONE', #18005, #23569 ) ;
#11835=LINE ( 'NONE', #7655, #1330 ) ;
#11836=ORIENTED_EDGE ( 'NONE', *, *, #1400, .T. ) ;
#11838=ORIENTED_EDGE ( 'NONE', *, *, #5323, .T. ) ;
#11839=FACE_OUTER_BOUND ( 'NONE', #7855, .T. ) ;
#11840=DIRECTION ( 'NONE',  ( -0.000000000000000000, -0.000000000000000000, -1.000000000000000000 ) ) ;
#11841=DIRECTION ( 'NONE',  ( -0.000000000000000000, -0.000000000000000000, -1.000000000000000000 ) ) ;
#11848=ORIENTED_EDGE ( 'NONE', *, *, #27692, .T. ) ;
#11854=CARTESIAN_POINT ( 'NONE',  ( 157.9999999999999432, 213.4763749774776045, -45.00000000000000000 ) ) ;
#11857=CARTESIAN_POINT ( 'NONE',  ( 157.9999999999999432, 211.4763749774776045, 45.00000000000000000 ) ) ;
#11859=ORIENTED_EDGE ( 'NONE', *, *, #22561, .F. ) ;
#11866=DIRECTION ( 'NONE',  ( -0.8916010070298056034, -0.4528218681373908372, 0.000000000000000000 ) ) ;
#11867=ORIENTED_EDGE ( 'NONE', *, *, #10879, .T. ) ;
#11868=EDGE_CURVE ( 'NONE', #13193, #11551, #21192, .T. ) ;
#11871=LINE ( 'NONE', #20615, #9493 ) ;
#11875=EDGE_CURVE ( 'NONE', #3644, #7560, #25639, .T. ) ;
#11876=ORIENTED_EDGE ( 'NONE', *, *, #3141, .F. ) ;
#11877=ORIENTED_EDGE ( 'NONE', *, *, #9815, .F. ) ;
#11882=DIRECTION ( 'NONE',  ( 0.000000000000000000, -1.000000000000000000, 0.000000000000000000 ) ) ;
#11885=VECTOR ( 'NONE', #21115, 1000.000000000000000 ) ;
#11887=DIRECTION ( 'NONE',  ( -0.8916010070300384172, 0.4528218681369324261, 0.000000000000000000 ) ) ;
#11888=EDGE_CURVE ( 'NONE', #13449, #26259, #12872, .T. ) ;
#11890=CARTESIAN_POINT ( 'NONE',  ( 158.0000000000001990, 186.3976249024084666, 45.00000000000000000 ) ) ;
#11898=ORIENTED_EDGE ( 'NONE', *, *, #11473, .F. ) ;
#11905=EDGE_CURVE ( 'NONE', #26049, #15387, #23920, .T. ) ;
#11907=EDGE_CURVE ( 'NONE', #23339, #26492, #19463, .T. ) ;
#11911=DIRECTION ( 'NONE',  ( 0.000000000000000000, -1.000000000000000000, 0.000000000000000000 ) ) ;
#11912=PLANE ( 'NONE',  #10899 ) ;
#11918=CARTESIAN_POINT ( 'NONE',  ( 158.0000000000008242, 126.2086247222394206, 45.00000000000000000 ) ) ;
#11921=DIRECTION ( 'NONE',  ( 0.8916010070293584056, 0.4528218681382713551, 0.000000000000000000 ) ) ;
#11925=CARTESIAN_POINT ( 'NONE',  ( 157.4999999999998579, 223.7618125112605298, -45.00000000000000000 ) ) ;
#11928=CARTESIAN_POINT ( 'NONE',  ( 158.0000000000007105, 136.2401247522676044, 45.00000000000000000 ) ) ;
#11933=LINE ( 'NONE', #1276, #18004 ) ;
#11934=VERTEX_POINT ( 'NONE', #1652 ) ;
#11937=EDGE_CURVE ( 'NONE', #16168, #6585, #21334, .T. ) ;
#11938=LINE ( 'NONE', #2582, #6080 ) ;
#11940=VERTEX_POINT ( 'NONE', #3946 ) ;
#11953=DIRECTION ( 'NONE',  ( 1.000000000000000000, 0.000000000000000000, -0.000000000000000000 ) ) ;
#11955=VERTEX_POINT ( 'NONE', #14887 ) ;
#11957=EDGE_CURVE ( 'NONE', #12076, #15277, #23637, .T. ) ;
#11958=VECTOR ( 'NONE', #3197, 1000.000000000000000 ) ;
#11960=CARTESIAN_POINT ( 'NONE',  ( 157.4999999999998579, 146.0176872785422404, 45.00000000000000000 ) ) ;
#11964=VERTEX_POINT ( 'NONE', #8124 ) ;
#11967=LINE ( 'NONE', #14261, #25979 ) ;
#11968=EDGE_CURVE ( 'NONE', #10398, #18134, #21472, .T. ) ;
#11971=CARTESIAN_POINT ( 'NONE',  ( 157.9999999999996874, 264.1417501351260171, 45.00000000000000000 ) ) ;
#11972=EDGE_CURVE ( 'NONE', #26778, #14369, #19320, .T. ) ;
#11973=CARTESIAN_POINT ( 'NONE',  ( 157.4999999999998579, 60.74993702330277756, 45.00000000000000000 ) ) ;
#11975=ORIENTED_EDGE ( 'NONE', *, *, #10666, .T. ) ;
#11976=DIRECTION ( 'NONE',  ( 0.000000000000000000, -1.000000000000000000, 0.000000000000000000 ) ) ;
#11977=ORIENTED_EDGE ( 'NONE', *, *, #17402, .F. ) ;
#11981=LINE ( 'NONE', #5355, #16280 ) ;
#11983=LINE ( 'NONE', #26775, #10033 ) ;
#11986=VECTOR ( 'NONE', #12697, 1000.000000000000227 ) ;
#11988=ORIENTED_EDGE ( 'NONE', *, *, #16810, .T. ) ;
#11989=LINE ( 'NONE', #18582, #1287 ) ;
#11992=ORIENTED_EDGE ( 'NONE', *, *, #12906, .F. ) ;
#12001=ORIENTED_EDGE ( 'NONE', *, *, #25282, .F. ) ;
#12008=ORIENTED_EDGE ( 'NONE', *, *, #25783, .T. ) ;
#12014=DIRECTION ( 'NONE',  ( 0.8916010070297244461, 0.4528218681375507093, 0.000000000000000000 ) ) ;
#12017=EDGE_CURVE ( 'NONE', #24036, #9050, #19741, .T. ) ;
#12019=CARTESIAN_POINT ( 'NONE',  ( 158.0000000000004263, 166.3346248423521274, 45.00000000000000000 ) ) ;
#12020=CARTESIAN_POINT ( 'NONE',  ( 157.4999999999998579, 141.0019372635281627, 45.00000000000000000 ) ) ;
#12022=VECTOR ( 'NONE', #6493, 1000.000000000000000 ) ;
#12026=DIRECTION ( 'NONE',  ( 0.4528218681382319422, 0.8916010070293783896, -0.000000000000000000 ) ) ;
#12029=ORIENTED_EDGE ( 'NONE', *, *, #22633, .F. ) ;
#12031=AXIS2_PLACEMENT_3D ( 'NONE', #27101, #20639, #27238 ) ;
#12032=CARTESIAN_POINT ( 'NONE',  ( 157.4999999999998579, 168.5885623461056184, 45.00000000000000000 ) ) ;
#12034=EDGE_CURVE ( 'NONE', #9697, #14502, #7102, .T. ) ;
#12036=DIRECTION ( 'NONE',  ( 0.8916010070293409751, 0.4528218681383056610, 0.000000000000000000 ) ) ;
#12039=EDGE_LOOP ( 'NONE', ( #15955, #15454, #9550, #25542 ) ) ;
#12040=LINE ( 'NONE', #547, #1806 ) ;
#12041=ORIENTED_EDGE ( 'NONE', *, *, #7692, .T. ) ;
#12045=EDGE_LOOP ( 'NONE', ( #22347, #23303, #20965, #10271 ) ) ;
#12050=FACE_OUTER_BOUND ( 'NONE', #21751, .T. ) ;
#12053=LINE ( 'NONE', #27118, #8246 ) ;
#12057=CARTESIAN_POINT ( 'NONE',  ( 157.4999999999998579, 118.4310621959647563, 45.00000000000000000 ) ) ;
#12063=LINE ( 'NONE', #20811, #5198 ) ;
#12064=VERTEX_POINT ( 'NONE', #16021 ) ;
#12069=LINE ( 'NONE', #19180, #9780 ) ;
#12070=VECTOR ( 'NONE', #20664, 1000.000000000000000 ) ;
#12071=VERTEX_POINT ( 'NONE', #65 ) ;
#12072=ORIENTED_EDGE ( 'NONE', *, *, #3569, .T. ) ;
#12074=CARTESIAN_POINT ( 'NONE',  ( 157.9999999999998863, 216.4921249924925348, -45.00000000000000000 ) ) ;
#12076=VERTEX_POINT ( 'NONE', #2638 ) ;
#12080=LINE ( 'NONE', #20827, #2023 ) ;
#12081=VECTOR ( 'NONE', #5951, 1000.000000000000114 ) ;
#12084=EDGE_CURVE ( 'NONE', #21404, #13671, #17874, .T. ) ;
#12087=FACE_OUTER_BOUND ( 'NONE', #23266, .T. ) ;
#12091=EDGE_CURVE ( 'NONE', #12823, #4413, #4501, .T. ) ;
#12092=DIRECTION ( 'NONE',  ( -0.8916010070296226386, -0.4528218681377511046, 0.000000000000000000 ) ) ;
#12094=EDGE_CURVE ( 'NONE', #2548, #7910, #22474, .T. ) ;
#12097=EDGE_CURVE ( 'NONE', #11940, #23711, #2489, .T. ) ;
#12099=CARTESIAN_POINT ( 'NONE',  ( 158.0000000000009663, 115.6692496847042264, -45.00000000000000000 ) ) ;
#12101=ORIENTED_EDGE ( 'NONE', *, *, #3517, .T. ) ;
#12102=VECTOR ( 'NONE', #14099, 1000.000000000000114 ) ;
#12104=CARTESIAN_POINT ( 'NONE',  ( 158.0000000000004832, 163.3188748273380213, -45.00000000000000000 ) ) ;
#12108=ORIENTED_EDGE ( 'NONE', *, *, #14326, .T. ) ;
#12110=LINE ( 'NONE', #13842, #8804 ) ;
#12111=CARTESIAN_POINT ( 'NONE',  ( 157.9999999999997158, 258.6181251126050711, 45.00000000000000000 ) ) ;
#12113=VERTEX_POINT ( 'NONE', #9409 ) ;
#12114=LINE ( 'NONE', #3743, #21425 ) ;
#12116=CARTESIAN_POINT ( 'NONE',  ( 158.0000000000016200, 52.97237449702815582, -45.00000000000000000 ) ) ;
#12117=ORIENTED_EDGE ( 'NONE', *, *, #12806, .F. ) ;
#12124=CARTESIAN_POINT ( 'NONE',  ( 158.0000000000014779, 65.51174953456337846, -45.00000000000000000 ) ) ;
#12126=DIRECTION ( 'NONE',  ( -0.8916010070293584056, -0.4528218681382712996, 0.000000000000000000 ) ) ;
#12127=VECTOR ( 'NONE', #12558, 1000.000000000000000 ) ;
#12132=CARTESIAN_POINT ( 'NONE',  ( 158.0000000000013074, 81.06687458711267880, 45.00000000000000000 ) ) ;
#12135=CARTESIAN_POINT ( 'NONE',  ( 158.0000000000005684, 153.2873747973098659, 45.00000000000000000 ) ) ;
#12141=EDGE_CURVE ( 'NONE', #20397, #1420, #24775, .T. ) ;
#12142=CARTESIAN_POINT ( 'NONE',  ( 157.9999999999999716, 210.9684999699701393, 45.00000000000000000 ) ) ;
#12143=DIRECTION ( 'NONE',  ( -0.000000000000000000, -0.000000000000000000, -1.000000000000000000 ) ) ;
#12146=DIRECTION ( 'NONE',  ( -0.000000000000000000, 0.000000000000000000, -1.000000000000000000 ) ) ;
#12148=VERTEX_POINT ( 'NONE', #18309 ) ;
#12152=ORIENTED_EDGE ( 'NONE', *, *, #25843, .T. ) ;
#12153=VECTOR ( 'NONE', #15415, 1000.000000000000227 ) ;
#12157=EDGE_LOOP ( 'NONE', ( #27025, #5869, #17076, #4543 ) ) ;
#12163=VECTOR ( 'NONE', #2561, 1000.000000000000114 ) ;
#12164=DIRECTION ( 'NONE',  ( -0.8916010070293995948, -0.4528218681381900867, 0.000000000000000000 ) ) ;
#12166=CARTESIAN_POINT ( 'NONE',  ( 157.9999999999997726, 248.5866250825770294, 45.00000000000000000 ) ) ;
#12168=AXIS2_PLACEMENT_3D ( 'NONE', #10856, #8560, #17309 ) ;
#12171=PLANE ( 'NONE',  #26751 ) ;
#12172=VERTEX_POINT ( 'NONE', #20595 ) ;
#12174=EDGE_CURVE ( 'NONE', #2119, #2123, #3346, .T. ) ;
#12175=EDGE_CURVE ( 'NONE', #1568, #11551, #21012, .T. ) ;
#12178=CARTESIAN_POINT ( 'NONE',  ( 158.0000000000015348, 60.49599951954928656, 45.00000000000000000 ) ) ;
#12180=VERTEX_POINT ( 'NONE', #27060 ) ;
#12191=EDGE_LOOP ( 'NONE', ( #4323, #11064, #28146, #19258 ) ) ;
#12196=PLANE ( 'NONE',  #13916 ) ;
#12198=DIRECTION ( 'NONE',  ( -0.000000000000000000, -0.000000000000000000, -1.000000000000000000 ) ) ;
#12206=VECTOR ( 'NONE', #23346, 1000.000000000000000 ) ;
#12209=ORIENTED_EDGE ( 'NONE', *, *, #18754, .T. ) ;
#12214=DIRECTION ( 'NONE',  ( 0.8916010070293383105, -0.4528218681383106015, 0.000000000000000000 ) ) ;
#12216=ORIENTED_EDGE ( 'NONE', *, *, #15762, .T. ) ;
#12219=VERTEX_POINT ( 'NONE', #3489 ) ;
#12222=ORIENTED_EDGE ( 'NONE', *, *, #25990, .F. ) ;
#12223=VECTOR ( 'NONE', #845, 1000.000000000000114 ) ;
#12226=VECTOR ( 'NONE', #16903, 1000.000000000000000 ) ;
#12228=DIRECTION ( 'NONE',  ( 0.000000000000000000, -1.000000000000000000, 0.000000000000000000 ) ) ;
#12229=EDGE_CURVE ( 'NONE', #5272, #9114, #20879, .T. ) ;
#12230=CARTESIAN_POINT ( 'NONE',  ( 157.4999999999998579, 93.35231212089433939, 45.00000000000000000 ) ) ;
#12234=CARTESIAN_POINT ( 'NONE',  ( 157.4999999999998579, 196.1751874286831026, 45.00000000000000000 ) ) ;
#12238=LINE ( 'NONE', #10345, #2209 ) ;
#12241=ORIENTED_EDGE ( 'NONE', *, *, #17710, .T. ) ;
#12247=AXIS2_PLACEMENT_3D ( 'NONE', #6103, #3943, #12308 ) ;
#12251=LINE ( 'NONE', #25575, #24595 ) ;
#12253=ADVANCED_FACE ( 'NONE', ( #3203 ), #9964, .F. ) ;
#12256=EDGE_CURVE ( 'NONE', #6469, #24347, #25328, .T. ) ;
#12258=EDGE_CURVE ( 'NONE', #7010, #27514, #13870, .T. ) ;
#12266=DIRECTION ( 'NONE',  ( 0.8916010070293584056, -0.4528218681382712996, 0.000000000000000000 ) ) ;
#12269=CARTESIAN_POINT ( 'NONE',  ( 157.4999999999997158, 258.8720626163585621, 45.00000000000000000 ) ) ;
#12272=DIRECTION ( 'NONE',  ( -0.8916010070295011802, -0.4528218681379903021, 0.000000000000000000 ) ) ;
#12274=PLANE ( 'NONE',  #23945 ) ;
#12276=ORIENTED_EDGE ( 'NONE', *, *, #9034, .T. ) ;
#12277=CARTESIAN_POINT ( 'NONE',  ( 157.4999999999998579, 191.1594374136689964, -45.00000000000000000 ) ) ;
#12278=EDGE_LOOP ( 'NONE', ( #5757, #7008, #6295, #8867 ) ) ;
#12282=EDGE_LOOP ( 'NONE', ( #1771, #21818, #17669, #12648 ) ) ;
#12283=PLANE ( 'NONE',  #27572 ) ;
#12284=DIRECTION ( 'NONE',  ( -0.000000000000000000, 0.000000000000000000, -1.000000000000000000 ) ) ;
#12285=VERTEX_POINT ( 'NONE', #7671 ) ;
#12288=EDGE_CURVE ( 'NONE', #27871, #11282, #25186, .T. ) ;
#12289=DIRECTION ( 'NONE',  ( 0.4528218681378310406, -0.8916010070295820045, 0.000000000000000000 ) ) ;
#12290=DIRECTION ( 'NONE',  ( 0.4528218681370124177, 0.8916010070299977830, -0.000000000000000000 ) ) ;
#12292=ORIENTED_EDGE ( 'NONE', *, *, #9537, .T. ) ;
#12296=EDGE_CURVE ( 'NONE', #16250, #11334, #2931, .T. ) ;
#12297=ORIENTED_EDGE ( 'NONE', *, *, #19617, .T. ) ;
#12298=ORIENTED_EDGE ( 'NONE', *, *, #8149, .F. ) ;
#12299=PLANE ( 'NONE',  #15754 ) ;
#12304=VECTOR ( 'NONE', #123, 1000.000000000000114 ) ;
#12305=CARTESIAN_POINT ( 'NONE',  ( 158.0000000000008242, 126.2086247222394206, 45.00000000000000000 ) ) ;
#12306=LINE ( 'NONE', #16746, #25939 ) ;
#12308=DIRECTION ( 'NONE',  ( -0.000000000000000000, 0.000000000000000000, -1.000000000000000000 ) ) ;
#12309=LINE ( 'NONE', #23635, #13387 ) ;
#12310=CARTESIAN_POINT ( 'NONE',  ( 157.4999999999995737, 203.6988124512014338, -45.00000000000000000 ) ) ;
#12313=DIRECTION ( 'NONE',  ( 0.8916010070296124246, -0.4528218681377710886, 0.000000000000000000 ) ) ;
#12315=DIRECTION ( 'NONE',  ( -0.000000000000000000, -0.000000000000000000, -1.000000000000000000 ) ) ;
#12318=EDGE_CURVE ( 'NONE', #11476, #26259, #5790, .T. ) ;
#12319=ORIENTED_EDGE ( 'NONE', *, *, #23496, .F. ) ;
#12321=EDGE_CURVE ( 'NONE', #23236, #11585, #6210, .T. ) ;
#12322=CARTESIAN_POINT ( 'NONE',  ( 157.4999999999997158, 258.8720626163585621, 45.00000000000000000 ) ) ;
#12326=ORIENTED_EDGE ( 'NONE', *, *, #22561, .T. ) ;
#12327=VERTEX_POINT ( 'NONE', #21729 ) ;
#12334=DIRECTION ( 'NONE',  ( 0.8916010070298556744, -0.4528218681372921384, 0.000000000000000000 ) ) ;
#12335=EDGE_CURVE ( 'NONE', #2081, #17634, #14853, .T. ) ;
#12336=CARTESIAN_POINT ( 'NONE',  ( 157.4999999999998579, 123.4468122109788482, 45.00000000000000000 ) ) ;
#12339=LINE ( 'NONE', #1399, #27435 ) ;
#12343=DIRECTION ( 'NONE',  ( -0.8916010070293383105, -0.4528218681383106015, 0.000000000000000000 ) ) ;
#12344=DIRECTION ( 'NONE',  ( 0.000000000000000000, -1.000000000000000000, 0.000000000000000000 ) ) ;
#12345=DIRECTION ( 'NONE',  ( 0.000000000000000000, -1.000000000000000000, 0.000000000000000000 ) ) ;
#12349=LINE ( 'NONE', #16512, #5569 ) ;
#12354=DIRECTION ( 'NONE',  ( 1.000000000000000000, 0.000000000000000000, -0.000000000000000000 ) ) ;
#12362=ORIENTED_EDGE ( 'NONE', *, *, #19827, .T. ) ;
#12363=VECTOR ( 'NONE', #17296, 999.9999999999998863 ) ;
#12365=VECTOR ( 'NONE', #1599, 1000.000000000000114 ) ;
#12370=DIRECTION ( 'NONE',  ( 0.000000000000000000, -1.000000000000000000, 0.000000000000000000 ) ) ;
#12371=VECTOR ( 'NONE', #12560, 1000.000000000000227 ) ;
#12372=VECTOR ( 'NONE', #454, 1000.000000000000000 ) ;
#12374=CARTESIAN_POINT ( 'NONE',  ( 158.0000000000002274, 183.8897498949014278, 45.00000000000000000 ) ) ;
#12375=DIRECTION ( 'NONE',  ( 1.000000000000000000, -0.000000000000000000, -0.000000000000000000 ) ) ;
#12376=EDGE_CURVE ( 'NONE', #5352, #61, #3624, .T. ) ;
#12382=EDGE_LOOP ( 'NONE', ( #1922, #778, #2797, #14870 ) ) ;
#12385=EDGE_CURVE ( 'NONE', #1176, #1637, #1615, .T. ) ;
#12390=ORIENTED_EDGE ( 'NONE', *, *, #956, .T. ) ;
#12397=CARTESIAN_POINT ( 'NONE',  ( 157.4999999999998010, 233.7933125412885147, 45.00000000000000000 ) ) ;
#12400=DIRECTION ( 'NONE',  ( 0.4528218681378310406, -0.8916010070295820045, 0.000000000000000000 ) ) ;
#12403=ORIENTED_EDGE ( 'NONE', *, *, #11905, .F. ) ;
#12408=DIRECTION ( 'NONE',  ( -0.000000000000000000, -0.000000000000000000, -1.000000000000000000 ) ) ;
#12415=LINE ( 'NONE', #6067, #1455 ) ;
#12416=DIRECTION ( 'NONE',  ( 0.8916010070299977830, -0.4528218681370124177, 0.000000000000000000 ) ) ;
#12418=PLANE ( 'NONE',  #19695 ) ;
#12419=EDGE_CURVE ( 'NONE', #7618, #22209, #14701, .T. ) ;
#12420=AXIS2_PLACEMENT_3D ( 'NONE', #21533, #19667, #23841 ) ;
#12421=VERTEX_POINT ( 'NONE', #28309 ) ;
#12424=CARTESIAN_POINT ( 'NONE',  ( 158.0000000000003695, 173.3503748573662051, -45.00000000000000000 ) ) ;
#12425=LINE ( 'NONE', #5372, #10329 ) ;
#12427=DIRECTION ( 'NONE',  ( -0.8916010070296838119, -0.4528218681376305899, 0.000000000000000000 ) ) ;
#12429=CARTESIAN_POINT ( 'NONE',  ( 157.4999999999998579, 125.9546872184859012, 45.00000000000000000 ) ) ;
#12431=VERTEX_POINT ( 'NONE', #8657 ) ;
#12432=ORIENTED_EDGE ( 'NONE', *, *, #3620, .F. ) ;
#12435=VECTOR ( 'NONE', #20726, 1000.000000000000000 ) ;
#12438=EDGE_LOOP ( 'NONE', ( #13509, #22096, #14724, #16653 ) ) ;
#12440=VECTOR ( 'NONE', #3487, 1000.000000000000000 ) ;
#12442=CARTESIAN_POINT ( 'NONE',  ( 187.4999999999996305, 288.9665627064425166, -45.00000000000000000 ) ) ;
#12448=EDGE_CURVE ( 'NONE', #6469, #19409, #10669, .T. ) ;
#12449=DIRECTION ( 'NONE',  ( 0.000000000000000000, -1.000000000000000000, 0.000000000000000000 ) ) ;
#12451=CARTESIAN_POINT ( 'NONE',  ( 158.0000000000000853, 198.4291249324366504, 45.00000000000000000 ) ) ;
#12457=DIRECTION ( 'NONE',  ( 0.8916010070296632728, -0.4528218681376712240, 0.000000000000000000 ) ) ;
#12458=DIRECTION ( 'NONE',  ( 0.000000000000000000, -1.000000000000000000, 0.000000000000000000 ) ) ;
#12460=ORIENTED_EDGE ( 'NONE', *, *, #12963, .F. ) ;
#12461=VECTOR ( 'NONE', #13831, 1000.000000000000114 ) ;
#12463=ORIENTED_EDGE ( 'NONE', *, *, #15147, .T. ) ;
#12465=EDGE_LOOP ( 'NONE', ( #14679, #4462, #13228, #13734 ) ) ;
#12469=ORIENTED_EDGE ( 'NONE', *, *, #6660, .F. ) ;
#12471=CARTESIAN_POINT ( 'NONE',  ( 158.0000000000001421, 193.4133749174225443, -45.00000000000000000 ) ) ;
#12473=VECTOR ( 'NONE', #2524, 1000.000000000000000 ) ;
#12474=CARTESIAN_POINT ( 'NONE',  ( 158.0000000000003411, 175.8582498648732440, 45.00000000000000000 ) ) ;
#12480=EDGE_CURVE ( 'NONE', #27327, #21761, #8791, .T. ) ;
#12489=EDGE_CURVE ( 'NONE', #17959, #4884, #6638, .T. ) ;
#12492=ORIENTED_EDGE ( 'NONE', *, *, #19561, .F. ) ;
#12497=VECTOR ( 'NONE', #5664, 1000.000000000000000 ) ;
#12499=VECTOR ( 'NONE', #10290, 1000.000000000000000 ) ;
#12501=ORIENTED_EDGE ( 'NONE', *, *, #12385, .T. ) ;
#12502=ORIENTED_EDGE ( 'NONE', *, *, #21182, .T. ) ;
#12509=VECTOR ( 'NONE', #21546, 1000.000000000000114 ) ;
#12517=CARTESIAN_POINT ( 'NONE',  ( 158.0000000000014495, 68.01962454207041731, 45.00000000000000000 ) ) ;
#12518=DIRECTION ( 'NONE',  ( 0.8916010070299064116, -0.4528218681371922183, 0.000000000000000000 ) ) ;
#12522=EDGE_CURVE ( 'NONE', #21564, #26706, #24303, .T. ) ;
#12524=ORIENTED_EDGE ( 'NONE', *, *, #5858, .T. ) ;
#12528=ORIENTED_EDGE ( 'NONE', *, *, #7031, .T. ) ;
#12531=DIRECTION ( 'NONE',  ( -0.000000000000000000, -0.000000000000000000, -1.000000000000000000 ) ) ;
#12532=ORIENTED_EDGE ( 'NONE', *, *, #24973, .T. ) ;
#12534=ORIENTED_EDGE ( 'NONE', *, *, #22789, .F. ) ;
#12536=DIRECTION ( 'NONE',  ( -0.8916010070293584056, 0.4528218681382713551, 0.000000000000000000 ) ) ;
#12537=VECTOR ( 'NONE', #12883, 1000.000000000000000 ) ;
#12539=CARTESIAN_POINT ( 'NONE',  ( 158.0000000000014779, 63.51174953456337136, 45.00000000000000000 ) ) ;
#12541=ORIENTED_EDGE ( 'NONE', *, *, #14579, .T. ) ;
#12545=EDGE_CURVE ( 'NONE', #27805, #6438, #24031, .T. ) ;
#12547=DIRECTION ( 'NONE',  ( 1.000000000000000000, 0.000000000000000000, -0.000000000000000000 ) ) ;
#12548=FACE_OUTER_BOUND ( 'NONE', #15787, .T. ) ;
#12549=VECTOR ( 'NONE', #6233, 1000.000000000000000 ) ;
#12550=PLANE ( 'NONE',  #21597 ) ;
#12552=ORIENTED_EDGE ( 'NONE', *, *, #17975, .F. ) ;
#12553=AXIS2_PLACEMENT_3D ( 'NONE', #7107, #19890, #2644 ) ;
#12554=LINE ( 'NONE', #14848, #16898 ) ;
#12556=FACE_OUTER_BOUND ( 'NONE', #26493, .T. ) ;
#12558=DIRECTION ( 'NONE',  ( -0.000000000000000000, -0.000000000000000000, -1.000000000000000000 ) ) ;
#12560=DIRECTION ( 'NONE',  ( 0.8916010070294699830, -0.4528218681380514199, 0.000000000000000000 ) ) ;
#12567=ORIENTED_EDGE ( 'NONE', *, *, #6434, .T. ) ;
#12570=ORIENTED_EDGE ( 'NONE', *, *, #12335, .T. ) ;
#12574=ORIENTED_EDGE ( 'NONE', *, *, #3638, .T. ) ;
#12575=AXIS2_PLACEMENT_3D ( 'NONE', #22312, #8808, #22022 ) ;
#12578=ORIENTED_EDGE ( 'NONE', *, *, #19957, .F. ) ;
#12579=VECTOR ( 'NONE', #1787, 1000.000000000000114 ) ;
#12581=DIRECTION ( 'NONE',  ( -0.8916010070296834789, -0.4528218681376312005, 0.000000000000000000 ) ) ;
#12582=ADVANCED_FACE ( 'NONE', ( #15553 ), #9223, .F. ) ;
#12583=FACE_OUTER_BOUND ( 'NONE', #5101, .T. ) ;
#12584=EDGE_CURVE ( 'NONE', #9066, #22237, #15698, .T. ) ;
#12585=CARTESIAN_POINT ( 'NONE',  ( 158.0000000000017053, 43.44874947450702507, -45.00000000000000000 ) ) ;
#12587=DIRECTION ( 'NONE',  ( 0.000000000000000000, -1.000000000000000000, 0.000000000000000000 ) ) ;
#12588=LINE ( 'NONE', #1778, #3910 ) ;
#12590=EDGE_LOOP ( 'NONE', ( #8098, #14969, #25763, #25932 ) ) ;
#12591=LINE ( 'NONE', #14884, #5787 ) ;
#12593=CARTESIAN_POINT ( 'NONE',  ( 158.0000000000005400, 153.7952498048169048, 45.00000000000000000 ) ) ;
#12595=ORIENTED_EDGE ( 'NONE', *, *, #24398, .T. ) ;
#12596=VECTOR ( 'NONE', #8610, 1000.000000000000000 ) ;
#12603=ORIENTED_EDGE ( 'NONE', *, *, #1761, .T. ) ;
#12606=LINE ( 'NONE', #20926, #20881 ) ;
#12608=ORIENTED_EDGE ( 'NONE', *, *, #23776, .T. ) ;
#12610=VERTEX_POINT ( 'NONE', #4609 ) ;
#12616=CARTESIAN_POINT ( 'NONE',  ( 157.9999999999999147, 215.9842499849850697, 45.00000000000000000 ) ) ;
#12618=EDGE_CURVE ( 'NONE', #3081, #27311, #1021, .T. ) ;
#12621=AXIS2_PLACEMENT_3D ( 'NONE', #5405, #7713, #10007 ) ;
#12622=CARTESIAN_POINT ( 'NONE',  ( 158.0000000000006253, 146.2716247822957598, -45.00000000000000000 ) ) ;
#12628=DIRECTION ( 'NONE',  ( -0.000000000000000000, -0.000000000000000000, -1.000000000000000000 ) ) ;
#12632=LINE ( 'NONE', #6150, #23831 ) ;
#12638=AXIS2_PLACEMENT_3D ( 'NONE', #18235, #22397, #11921 ) ;
#12642=VECTOR ( 'NONE', #3631, 1000.000000000000000 ) ;
#12643=ORIENTED_EDGE ( 'NONE', *, *, #1911, .T. ) ;
#12648=ORIENTED_EDGE ( 'NONE', *, *, #10331, .T. ) ;
#12651=ADVANCED_FACE ( 'NONE', ( #882 ), #25017, .F. ) ;
#12653=AXIS2_PLACEMENT_3D ( 'NONE', #2811, #7133, #16466 ) ;
#12654=VECTOR ( 'NONE', #100, 1000.000000000000000 ) ;
#12655=DIRECTION ( 'NONE',  ( -0.000000000000000000, -0.000000000000000000, -1.000000000000000000 ) ) ;
#12656=CARTESIAN_POINT ( 'NONE',  ( 157.4999999999998010, 236.3011875487955251, -45.00000000000000000 ) ) ;
#12661=DIRECTION ( 'NONE',  ( 0.4528218681379515553, 0.8916010070295208312, -0.000000000000000000 ) ) ;
#12666=CARTESIAN_POINT ( 'NONE',  ( 157.4999999999996305, 288.9665627064425735, 45.00000000000000000 ) ) ;
#12667=CARTESIAN_POINT ( 'NONE',  ( 158.0000000000011369, 98.11412463215494029, -45.00000000000000000 ) ) ;
#12668=VERTEX_POINT ( 'NONE', #748 ) ;
#12675=ADVANCED_FACE ( 'NONE', ( #18551 ), #2894, .F. ) ;
#12678=VERTEX_POINT ( 'NONE', #13980 ) ;
#12681=DIRECTION ( 'NONE',  ( 0.8916010070299876800, -0.4528218681370323462, 0.000000000000000000 ) ) ;
#12686=ORIENTED_EDGE ( 'NONE', *, *, #26592, .T. ) ;
#12690=LINE ( 'NONE', #18713, #3556 ) ;
#12691=VECTOR ( 'NONE', #4452, 1000.000000000000114 ) ;
#12693=VECTOR ( 'NONE', #16155, 1000.000000000000000 ) ;
#12696=VECTOR ( 'NONE', #2344, 1000.000000000000227 ) ;
#12697=DIRECTION ( 'NONE',  ( 0.8916010070298455714, -0.4528218681373120669, 0.000000000000000000 ) ) ;
#12698=PLANE ( 'NONE',  #1902 ) ;
#12700=VERTEX_POINT ( 'NONE', #22726 ) ;
#12705=LINE ( 'NONE', #28034, #26370 ) ;
#12706=ORIENTED_EDGE ( 'NONE', *, *, #6319, .F. ) ;
#12709=EDGE_CURVE ( 'NONE', #2123, #21119, #9375, .T. ) ;
#12710=LINE ( 'NONE', #27898, #6960 ) ;
#12714=ORIENTED_EDGE ( 'NONE', *, *, #10623, .T. ) ;
#12716=ORIENTED_EDGE ( 'NONE', *, *, #8957, .T. ) ;
#12717=ORIENTED_EDGE ( 'NONE', *, *, #3738, .F. ) ;
#12718=VERTEX_POINT ( 'NONE', #16404 ) ;
#12721=ADVANCED_FACE ( 'NONE', ( #3028 ), #7359, .F. ) ;
#12725=LINE ( 'NONE', #23484, #19282 ) ;
#12726=CARTESIAN_POINT ( 'NONE',  ( 157.4999999999998579, 176.1121873686267350, -45.00000000000000000 ) ) ;
#12728=ORIENTED_EDGE ( 'NONE', *, *, #24668, .F. ) ;
#12729=DIRECTION ( 'NONE',  ( -0.000000000000000000, 0.000000000000000000, -1.000000000000000000 ) ) ;
#12737=CARTESIAN_POINT ( 'NONE',  ( 158.0000000000009379, 118.1771246922112653, 45.00000000000000000 ) ) ;
#12739=FACE_OUTER_BOUND ( 'NONE', #25608, .T. ) ;
#12740=LINE ( 'NONE', #13026, #838 ) ;
#12743=ADVANCED_FACE ( 'NONE', ( #1160 ), #14250, .F. ) ;
#12748=EDGE_CURVE ( 'NONE', #14709, #13208, #26381, .T. ) ;
#12749=ORIENTED_EDGE ( 'NONE', *, *, #4290, .T. ) ;
#12751=VERTEX_POINT ( 'NONE', #8594 ) ;
#12752=ORIENTED_EDGE ( 'NONE', *, *, #23231, .T. ) ;
#12756=DIRECTION ( 'NONE',  ( 0.4528218681376912080, -0.8916010070296530587, 0.000000000000000000 ) ) ;
#12759=DIRECTION ( 'NONE',  ( 0.8916010070293486356, 0.4528218681382907285, 0.000000000000000000 ) ) ;
#12766=CARTESIAN_POINT ( 'NONE',  ( 157.4999999999997442, 253.8563126013445697, -45.00000000000000000 ) ) ;
#12767=ORIENTED_EDGE ( 'NONE', *, *, #11587, .F. ) ;
#12768=AXIS2_PLACEMENT_3D ( 'NONE', #23845, #4006, #12793 ) ;
#12769=AXIS2_PLACEMENT_3D ( 'NONE', #5363, #3061, #20167 ) ;
#12773=ORIENTED_EDGE ( 'NONE', *, *, #17923, .F. ) ;
#12774=VERTEX_POINT ( 'NONE', #8453 ) ;
#12778=VERTEX_POINT ( 'NONE', #19221 ) ;
#12780=ORIENTED_EDGE ( 'NONE', *, *, #25957, .F. ) ;
#12782=EDGE_LOOP ( 'NONE', ( #24061, #6766, #4033, #12326 ) ) ;
#12783=VERTEX_POINT ( 'NONE', #19506 ) ;
#12787=VECTOR ( 'NONE', #1681, 1000.000000000000114 ) ;
#12788=CARTESIAN_POINT ( 'NONE',  ( 157.4999999999998295, 228.7775625262745223, -45.00000000000000000 ) ) ;
#12789=LINE ( 'NONE', #3863, #18530 ) ;
#12793=DIRECTION ( 'NONE',  ( -0.000000000000000000, 0.000000000000000000, -1.000000000000000000 ) ) ;
#12794=CARTESIAN_POINT ( 'NONE',  ( 157.4999999999997158, 261.3799376238655441, 45.00000000000000000 ) ) ;
#12803=ADVANCED_FACE ( 'NONE', ( #4549 ), #25967, .F. ) ;
#12806=EDGE_CURVE ( 'NONE', #27311, #21270, #19359, .T. ) ;
#12807=VECTOR ( 'NONE', #17123, 1000.000000000000000 ) ;
#12811=ORIENTED_EDGE ( 'NONE', *, *, #11017, .T. ) ;
#12815=VERTEX_POINT ( 'NONE', #23819 ) ;
#12821=EDGE_LOOP ( 'NONE', ( #14896, #25919, #26165, #13306 ) ) ;
#12823=VERTEX_POINT ( 'NONE', #11032 ) ;
#12827=CARTESIAN_POINT ( 'NONE',  ( 157.9999999999996589, 273.6653751576470768, 45.00000000000000000 ) ) ;
#12834=LINE ( 'NONE', #16852, #15235 ) ;
#12838=AXIS2_PLACEMENT_3D ( 'NONE', #20103, #24850, #437 ) ;
#12847=EDGE_CURVE ( 'NONE', #1670, #6691, #17063, .T. ) ;
#12848=CARTESIAN_POINT ( 'NONE',  ( 157.9999999999996874, 268.6496251426330559, -45.00000000000000000 ) ) ;
#12850=ORIENTED_EDGE ( 'NONE', *, *, #20779, .T. ) ;
#12851=ORIENTED_EDGE ( 'NONE', *, *, #9471, .T. ) ;
#12854=VERTEX_POINT ( 'NONE', #8731 ) ;
#12855=EDGE_LOOP ( 'NONE', ( #833, #8787, #2256, #3283 ) ) ;
#12858=DIRECTION ( 'NONE',  ( 1.000000000000000000, 0.000000000000000000, -0.000000000000000000 ) ) ;
#12863=CARTESIAN_POINT ( 'NONE',  ( 157.9999999999998010, 236.5551250525490161, -45.00000000000000000 ) ) ;
#12865=DIRECTION ( 'NONE',  ( 0.8916010070293783896, -0.4528218681382319422, 0.000000000000000000 ) ) ;
#12866=EDGE_CURVE ( 'NONE', #8798, #11076, #23963, .T. ) ;
#12868=VERTEX_POINT ( 'NONE', #28383 ) ;
#12870=DIRECTION ( 'NONE',  ( 1.000000000000000000, 0.000000000000000000, -0.000000000000000000 ) ) ;
#12872=LINE ( 'NONE', #24065, #11666 ) ;
#12873=ORIENTED_EDGE ( 'NONE', *, *, #22508, .F. ) ;
#12878=DIRECTION ( 'NONE',  ( -0.8916010070298665546, -0.4528218681372709331, 0.000000000000000000 ) ) ;
#12879=CARTESIAN_POINT ( 'NONE',  ( 157.4999999999998579, 68.27356204582390831, -45.00000000000000000 ) ) ;
#12882=VECTOR ( 'NONE', #13423, 1000.000000000000000 ) ;
#12883=DIRECTION ( 'NONE',  ( 0.000000000000000000, -1.000000000000000000, 0.000000000000000000 ) ) ;
#12887=ORIENTED_EDGE ( 'NONE', *, *, #7075, .T. ) ;
#12889=FACE_OUTER_BOUND ( 'NONE', #19939, .T. ) ;
#12890=AXIS2_PLACEMENT_3D ( 'NONE', #14422, #685, #18210 ) ;
#12893=CARTESIAN_POINT ( 'NONE',  ( 158.0000000000000853, 198.4291249324366504, -45.00000000000000000 ) ) ;
#12894=ADVANCED_FACE ( 'NONE', ( #4976 ), #27100, .F. ) ;
#12896=CARTESIAN_POINT ( 'NONE',  ( 157.4999999999998579, 198.6830624361901414, 45.00000000000000000 ) ) ;
#12898=CARTESIAN_POINT ( 'NONE',  ( 157.4999999999998579, 173.6043123611196961, -45.00000000000000000 ) ) ;
#12899=DIRECTION ( 'NONE',  ( -0.000000000000000000, -0.000000000000000000, -1.000000000000000000 ) ) ;
#12903=VECTOR ( 'NONE', #24552, 1000.000000000000000 ) ;
#12906=EDGE_CURVE ( 'NONE', #17008, #24175, #26824, .T. ) ;
#12908=DIRECTION ( 'NONE',  ( -0.000000000000000000, 0.000000000000000000, -1.000000000000000000 ) ) ;
#12909=LINE ( 'NONE', #21654, #7508 ) ;
#12910=ORIENTED_EDGE ( 'NONE', *, *, #27399, .T. ) ;
#12917=ORIENTED_EDGE ( 'NONE', *, *, #20897, .T. ) ;
#12919=ORIENTED_EDGE ( 'NONE', *, *, #10754, .T. ) ;
#12920=VERTEX_POINT ( 'NONE', #6995 ) ;
#12922=VERTEX_POINT ( 'NONE', #22226 ) ;
#12923=ORIENTED_EDGE ( 'NONE', *, *, #20084, .F. ) ;
#12926=LINE ( 'NONE', #16940, #16865 ) ;
#12933=DIRECTION ( 'NONE',  ( 0.4528218681383106015, 0.8916010070293384215, -0.000000000000000000 ) ) ;
#12934=CARTESIAN_POINT ( 'NONE',  ( 158.0000000000005684, 153.2873747973098659, 45.00000000000000000 ) ) ;
#12939=CARTESIAN_POINT ( 'NONE',  ( 158.0000000000000853, 200.9369999399436892, -45.00000000000000000 ) ) ;
#12941=VECTOR ( 'NONE', #15427, 1000.000000000000000 ) ;
#12943=VERTEX_POINT ( 'NONE', #26668 ) ;
#12946=VECTOR ( 'NONE', #13441, 1000.000000000000114 ) ;
#12954=CARTESIAN_POINT ( 'NONE',  ( 157.4999999999998579, 173.6043123611196961, 45.00000000000000000 ) ) ;
#12961=LINE ( 'NONE', #14973, #12365 ) ;
#12963=EDGE_CURVE ( 'NONE', #12180, #3701, #20065, .T. ) ;
#12968=PLANE ( 'NONE',  #4288 ) ;
#12969=ADVANCED_FACE ( 'NONE', ( #26520 ), #22665, .F. ) ;
#12975=CARTESIAN_POINT ( 'NONE',  ( 158.0000000000010800, 101.1298746471690038, -45.00000000000000000 ) ) ;
#12976=ORIENTED_EDGE ( 'NONE', *, *, #8640, .F. ) ;
#12978=DIRECTION ( 'NONE',  ( -0.8916010070293383105, -0.4528218681383106015, 0.000000000000000000 ) ) ;
#12989=DIRECTION ( 'NONE',  ( -0.8916010070295816714, 0.4528218681378317068, 0.000000000000000000 ) ) ;
#12993=LINE ( 'NONE', #2048, #23949 ) ;
#12996=EDGE_LOOP ( 'NONE', ( #16695, #936, #3006, #8877 ) ) ;
#12999=VERTEX_POINT ( 'NONE', #2969 ) ;
#13002=ORIENTED_EDGE ( 'NONE', *, *, #25566, .F. ) ;
#13005=CARTESIAN_POINT ( 'NONE',  ( 158.0000000000014779, 65.51174953456337846, 45.00000000000000000 ) ) ;
#13006=VECTOR ( 'NONE', #4051, 1000.000000000000114 ) ;
#13011=VECTOR ( 'NONE', #1825, 999.9999999999998863 ) ;
#13012=DIRECTION ( 'NONE',  ( 0.8916010070293783896, -0.4528218681382319422, 0.000000000000000000 ) ) ;
#13013=CARTESIAN_POINT ( 'NONE',  ( 158.0000000000000853, 198.9369999399436892, 45.00000000000000000 ) ) ;
#13017=DIRECTION ( 'NONE',  ( -1.000000000000000000, 0.000000000000000000, 0.000000000000000000 ) ) ;
#13019=DIRECTION ( 'NONE',  ( -0.8916010070294497769, 0.4528218681380914989, 0.000000000000000000 ) ) ;
#13024=PLANE ( 'NONE',  #19247 ) ;
#13026=CARTESIAN_POINT ( 'NONE',  ( 158.0000000000013642, 76.05112457209858690, -45.00000000000000000 ) ) ;
#13027=ORIENTED_EDGE ( 'NONE', *, *, #16682, .T. ) ;
#13034=VECTOR ( 'NONE', #13294, 1000.000000000000000 ) ;
#13036=DIRECTION ( 'NONE',  ( 0.8916010070299070778, 0.4528218681371909971, 0.000000000000000000 ) ) ;
#13046=DIRECTION ( 'NONE',  ( -0.8916010070299376089, -0.4528218681371311005, 0.000000000000000000 ) ) ;
#13048=ADVANCED_FACE ( 'NONE', ( #21197 ), #22803, .F. ) ;
#13051=DIRECTION ( 'NONE',  ( 1.000000000000000000, 0.000000000000000000, -0.000000000000000000 ) ) ;
#13055=CARTESIAN_POINT ( 'NONE',  ( 158.0000000000000000, 208.4606249624626457, -45.00000000000000000 ) ) ;
#13071=ORIENTED_EDGE ( 'NONE', *, *, #7356, .F. ) ;
#13076=DIRECTION ( 'NONE',  ( -0.000000000000000000, 0.000000000000000000, -1.000000000000000000 ) ) ;
#13077=EDGE_CURVE ( 'NONE', #24186, #3711, #16618, .T. ) ;
#13078=DIRECTION ( 'NONE',  ( -0.000000000000000000, -0.000000000000000000, -1.000000000000000000 ) ) ;
#13083=DIRECTION ( 'NONE',  ( 0.8916010070296936929, -0.4528218681376112165, 0.000000000000000000 ) ) ;
#13090=VECTOR ( 'NONE', #13839, 1000.000000000000000 ) ;
#13093=EDGE_CURVE ( 'NONE', #1111, #22350, #18903, .T. ) ;
#13095=CARTESIAN_POINT ( 'NONE',  ( 157.9999999999997158, 261.6338751276190351, -45.00000000000000000 ) ) ;
#13096=EDGE_LOOP ( 'NONE', ( #19121, #9417, #15538, #6122 ) ) ;
#13101=EDGE_CURVE ( 'NONE', #22209, #9386, #16757, .T. ) ;
#13105=VECTOR ( 'NONE', #22649, 1000.000000000000000 ) ;
#13108=VECTOR ( 'NONE', #15199, 1000.000000000000227 ) ;
#13110=DIRECTION ( 'NONE',  ( -0.8916010070294909662, -0.4528218681380102306, 0.000000000000000000 ) ) ;
#13114=VECTOR ( 'NONE', #2287, 999.9999999999998863 ) ;
#13116=FACE_OUTER_BOUND ( 'NONE', #20990, .T. ) ;
#13125=VERTEX_POINT ( 'NONE', #23356 ) ;
#13126=VECTOR ( 'NONE', #13843, 1000.000000000000114 ) ;
#13127=CARTESIAN_POINT ( 'NONE',  ( 158.0000000000012506, 86.08262460212675649, -45.00000000000000000 ) ) ;
#13128=DIRECTION ( 'NONE',  ( 0.8916010070293383105, -0.4528218681383106015, 0.000000000000000000 ) ) ;
#13129=LINE ( 'NONE', #14858, #22261 ) ;
#13130=VERTEX_POINT ( 'NONE', #18489 ) ;
#13132=EDGE_CURVE ( 'NONE', #410, #21206, #3386, .T. ) ;
#13135=EDGE_CURVE ( 'NONE', #19520, #19302, #20774, .T. ) ;
#13139=ORIENTED_EDGE ( 'NONE', *, *, #10390, .T. ) ;
#13140=VERTEX_POINT ( 'NONE', #3100 ) ;
#13148=PLANE ( 'NONE',  #10286 ) ;
#13150=VECTOR ( 'NONE', #3235, 999.9999999999998863 ) ;
#13153=CARTESIAN_POINT ( 'NONE',  ( 158.0000000000009663, 115.6692496847042264, 45.00000000000000000 ) ) ;
#13155=CARTESIAN_POINT ( 'NONE',  ( 157.9999999999997726, 241.5708750675630370, 45.00000000000000000 ) ) ;
#13157=PLANE ( 'NONE',  #24255 ) ;
#13158=DIRECTION ( 'NONE',  ( 0.8916010070296632728, -0.4528218681376712240, 0.000000000000000000 ) ) ;
#13159=ORIENTED_EDGE ( 'NONE', *, *, #1454, .T. ) ;
#13164=CARTESIAN_POINT ( 'NONE',  ( 158.0000000000001990, 186.3976249024084666, 45.00000000000000000 ) ) ;
#13165=CARTESIAN_POINT ( 'NONE',  ( 157.9999999999996589, 278.6811251726610976, 45.00000000000000000 ) ) ;
#13172=CARTESIAN_POINT ( 'NONE',  ( 158.0000000000015064, 63.00387452705633251, -45.00000000000000000 ) ) ;
#13174=ORIENTED_EDGE ( 'NONE', *, *, #4602, .T. ) ;
#13175=CARTESIAN_POINT ( 'NONE',  ( 157.9999999999997158, 261.1260001201120531, 45.00000000000000000 ) ) ;
#13182=CARTESIAN_POINT ( 'NONE',  ( 157.4999999999998579, 151.0334372935563465, 45.00000000000000000 ) ) ;
#13185=CARTESIAN_POINT ( 'NONE',  ( 157.4999999999998579, 141.0019372635281627, 45.00000000000000000 ) ) ;
#13186=PLANE ( 'NONE',  #6978 ) ;
#13187=CARTESIAN_POINT ( 'NONE',  ( 157.9999999999998579, 223.5078750075070104, 45.00000000000000000 ) ) ;
#13189=EDGE_CURVE ( 'NONE', #3105, #26789, #15029, .T. ) ;
#13190=DIRECTION ( 'NONE',  ( -0.000000000000000000, 0.000000000000000000, -1.000000000000000000 ) ) ;
#13191=CARTESIAN_POINT ( 'NONE',  ( 158.0000000000005400, 158.3031248123239436, -45.00000000000000000 ) ) ;
#13193=VERTEX_POINT ( 'NONE', #4094 ) ;
#13194=ADVANCED_FACE ( 'NONE', ( #12739 ), #1793, .F. ) ;
#13195=DIRECTION ( 'NONE',  ( 0.000000000000000000, -1.000000000000000000, 0.000000000000000000 ) ) ;
#13199=DIRECTION ( 'NONE',  ( 0.4528218681382319422, 0.8916010070293783896, -0.000000000000000000 ) ) ;
#13203=VECTOR ( 'NONE', #1841, 1000.000000000000000 ) ;
#13204=ORIENTED_EDGE ( 'NONE', *, *, #775, .F. ) ;
#13205=ADVANCED_FACE ( 'NONE', ( #26210 ), #19182, .F. ) ;
#13207=ORIENTED_EDGE ( 'NONE', *, *, #26700, .T. ) ;
#13208=VERTEX_POINT ( 'NONE', #28217 ) ;
#13210=DIRECTION ( 'NONE',  ( 0.4528218681377911836, 0.8916010070296023216, -0.000000000000000000 ) ) ;
#13217=PLANE ( 'NONE',  #3477 ) ;
#13219=CARTESIAN_POINT ( 'NONE',  ( 157.4999999999997442, 253.8563126013445697, 45.00000000000000000 ) ) ;
#13226=FACE_OUTER_BOUND ( 'NONE', #435, .T. ) ;
#13227=CARTESIAN_POINT ( 'NONE',  ( 158.0000000000011937, 91.09837461714084839, 45.00000000000000000 ) ) ;
#13228=ORIENTED_EDGE ( 'NONE', *, *, #19382, .F. ) ;
#13231=AXIS2_PLACEMENT_3D ( 'NONE', #6538, #2079, #2213 ) ;
#13232=CARTESIAN_POINT ( 'NONE',  ( 157.9999999999998010, 238.5551250525490161, -45.00000000000000000 ) ) ;
#13233=ORIENTED_EDGE ( 'NONE', *, *, #11972, .T. ) ;
#13235=ORIENTED_EDGE ( 'NONE', *, *, #10298, .T. ) ;
#13236=VECTOR ( 'NONE', #13761, 1000.000000000000000 ) ;
#13237=ADVANCED_FACE ( 'NONE', ( #21622 ), #19470, .F. ) ;
#13239=CARTESIAN_POINT ( 'NONE',  ( 157.4999999999994600, 216.2381874887387880, -45.00000000000000000 ) ) ;
#13244=VERTEX_POINT ( 'NONE', #19611 ) ;
#13247=ADVANCED_FACE ( 'NONE', ( #15174 ), #21771, .F. ) ;
#13248=VECTOR ( 'NONE', #23777, 1000.000000000000227 ) ;
#13252=AXIS2_PLACEMENT_3D ( 'NONE', #6805, #4790, #15587 ) ;
#13258=PLANE ( 'NONE',  #28061 ) ;
#13259=DIRECTION ( 'NONE',  ( -0.000000000000000000, 0.000000000000000000, -1.000000000000000000 ) ) ;
#13261=DIRECTION ( 'NONE',  ( 0.8916010070297542001, -0.4528218681374919230, 0.000000000000000000 ) ) ;
#13263=LINE ( 'NONE', #37, #7503 ) ;
#13270=VERTEX_POINT ( 'NONE', #2212 ) ;
#13273=VECTOR ( 'NONE', #9112, 1000.000000000000000 ) ;
#13275=CARTESIAN_POINT ( 'NONE',  ( 158.0000000000017337, 40.94087446699997912, 45.00000000000000000 ) ) ;
#13276=ORIENTED_EDGE ( 'NONE', *, *, #27105, .T. ) ;
#13286=CARTESIAN_POINT ( 'NONE',  ( 158.0000000000017337, 42.94087446699998623, 45.00000000000000000 ) ) ;
#13291=VECTOR ( 'NONE', #27252, 1000.000000000000000 ) ;
#13294=DIRECTION ( 'NONE',  ( -0.000000000000000000, -0.000000000000000000, -1.000000000000000000 ) ) ;
#13295=ORIENTED_EDGE ( 'NONE', *, *, #10407, .F. ) ;
#13296=DIRECTION ( 'NONE',  ( -0.8916010070295106171, 0.4528218681379715393, 0.000000000000000000 ) ) ;
#13305=CARTESIAN_POINT ( 'NONE',  ( 157.4999999999998579, 183.6358123911478799, -45.00000000000000000 ) ) ;
#13306=ORIENTED_EDGE ( 'NONE', *, *, #376, .F. ) ;
#13308=EDGE_LOOP ( 'NONE', ( #6645, #7881, #27700, #10920 ) ) ;
#13310=CARTESIAN_POINT ( 'NONE',  ( 158.0000000000010516, 105.6377496546760568, 45.00000000000000000 ) ) ;
#13313=VERTEX_POINT ( 'NONE', #15744 ) ;
#13314=VERTEX_POINT ( 'NONE', #19892 ) ;
#13328=DIRECTION ( 'NONE',  ( 0.4528218681383106015, -0.8916010070293384215, 0.000000000000000000 ) ) ;
#13331=ORIENTED_EDGE ( 'NONE', *, *, #7195, .T. ) ;
#13333=VECTOR ( 'NONE', #11882, 1000.000000000000000 ) ;
#13334=DIRECTION ( 'NONE',  ( 0.8916010070293383105, -0.4528218681383106015, 0.000000000000000000 ) ) ;
#13338=VECTOR ( 'NONE', #10533, 1000.000000000000000 ) ;
#13340=LINE ( 'NONE', #13630, #23973 ) ;
#13341=ORIENTED_EDGE ( 'NONE', *, *, #5359, .F. ) ;
#13344=ORIENTED_EDGE ( 'NONE', *, *, #14074, .T. ) ;
#13345=EDGE_LOOP ( 'NONE', ( #23399, #1173, #23543, #17391 ) ) ;
#13348=DIRECTION ( 'NONE',  ( 0.8916010070296732648, 0.4528218681376511845, 0.000000000000000000 ) ) ;
#13350=EDGE_CURVE ( 'NONE', #4902, #27901, #14431, .T. ) ;
#13351=VECTOR ( 'NONE', #20524, 1000.000000000000227 ) ;
#13353=PLANE ( 'NONE',  #13974 ) ;
#13356=LINE ( 'NONE', #24838, #22609 ) ;
#13357=CARTESIAN_POINT ( 'NONE',  ( 158.0000000000001137, 193.9212499249295831, 45.00000000000000000 ) ) ;
#13358=EDGE_CURVE ( 'NONE', #27297, #16487, #14568, .T. ) ;
#13363=EDGE_CURVE ( 'NONE', #11039, #22451, #1067, .T. ) ;
#13366=DIRECTION ( 'NONE',  ( -0.8916010070297345491, -0.4528218681375307253, 0.000000000000000000 ) ) ;
#13367=CARTESIAN_POINT ( 'NONE',  ( 157.4999999999998579, 153.5413123010633853, -45.00000000000000000 ) ) ;
#13369=ORIENTED_EDGE ( 'NONE', *, *, #19674, .T. ) ;
#13372=CARTESIAN_POINT ( 'NONE',  ( 157.4999999999998579, 73.28931206083800021, 45.00000000000000000 ) ) ;
#13374=ORIENTED_EDGE ( 'NONE', *, *, #27412, .F. ) ;
#13375=EDGE_LOOP ( 'NONE', ( #3742, #25099, #10437, #18943 ) ) ;
#13377=DIRECTION ( 'NONE',  ( 0.000000000000000000, -1.000000000000000000, 0.000000000000000000 ) ) ;
#13379=ORIENTED_EDGE ( 'NONE', *, *, #17090, .F. ) ;
#13382=EDGE_CURVE ( 'NONE', #1139, #749, #1205, .T. ) ;
#13383=LINE ( 'NONE', #22134, #10976 ) ;
#13384=ORIENTED_EDGE ( 'NONE', *, *, #24504, .F. ) ;
#13387=VECTOR ( 'NONE', #8268, 1000.000000000000114 ) ;
#13388=DIRECTION ( 'NONE',  ( -0.000000000000000000, 0.000000000000000000, -1.000000000000000000 ) ) ;
#13389=AXIS2_PLACEMENT_3D ( 'NONE', #5900, #1591, #14674 ) ;
#13399=ORIENTED_EDGE ( 'NONE', *, *, #8741, .T. ) ;
#13401=CARTESIAN_POINT ( 'NONE',  ( 157.4999999999997158, 263.8878126313725829, -45.00000000000000000 ) ) ;
#13402=DIRECTION ( 'NONE',  ( 0.8916010070296429557, -0.4528218681377111920, 0.000000000000000000 ) ) ;
#13403=ORIENTED_EDGE ( 'NONE', *, *, #21709, .F. ) ;
#13404=ORIENTED_EDGE ( 'NONE', *, *, #6181, .F. ) ;
#13406=EDGE_CURVE ( 'NONE', #17461, #16305, #22770, .T. ) ;
#13407=VECTOR ( 'NONE', #9963, 1000.000000000000227 ) ;
#13409=LINE ( 'NONE', #13701, #26403 ) ;
#13411=LINE ( 'NONE', #2131, #19444 ) ;
#13413=PLANE ( 'NONE',  #18666 ) ;
#13418=CARTESIAN_POINT ( 'NONE',  ( 158.0000000000009663, 113.1613746771971876, -45.00000000000000000 ) ) ;
#13419=DIRECTION ( 'NONE',  ( -0.000000000000000000, -0.000000000000000000, -1.000000000000000000 ) ) ;
#13421=CARTESIAN_POINT ( 'NONE',  ( 158.0000000000009095, 118.6849996997183041, 45.00000000000000000 ) ) ;
#13422=VECTOR ( 'NONE', #17046, 1000.000000000000000 ) ;
#13423=DIRECTION ( 'NONE',  ( -0.000000000000000000, -0.000000000000000000, -1.000000000000000000 ) ) ;
#13425=VERTEX_POINT ( 'NONE', #7400 ) ;
#13427=VECTOR ( 'NONE', #18410, 1000.000000000000000 ) ;
#13428=CARTESIAN_POINT ( 'NONE',  ( 157.9999999999998010, 234.0472500450420341, -45.00000000000000000 ) ) ;
#13430=VECTOR ( 'NONE', #23560, 1000.000000000000227 ) ;
#13432=DIRECTION ( 'NONE',  ( -0.000000000000000000, -0.000000000000000000, -1.000000000000000000 ) ) ;
#13433=VERTEX_POINT ( 'NONE', #3354 ) ;
#13436=EDGE_LOOP ( 'NONE', ( #10253, #24352, #22090, #23154 ) ) ;
#13441=DIRECTION ( 'NONE',  ( 0.8916010070297037959, -0.4528218681375912325, 0.000000000000000000 ) ) ;
#13444=EDGE_LOOP ( 'NONE', ( #9278, #3219, #14527, #21736 ) ) ;
#13449=VERTEX_POINT ( 'NONE', #7956 ) ;
#13451=DIRECTION ( 'NONE',  ( 0.8916010070293584056, -0.4528218681382712996, 0.000000000000000000 ) ) ;
#13454=EDGE_CURVE ( 'NONE', #19970, #17350, #12425, .T. ) ;
#13457=VECTOR ( 'NONE', #14522, 1000.000000000000000 ) ;
#13462=CARTESIAN_POINT ( 'NONE',  ( 157.9999999999997442, 256.1102501050980322, 45.00000000000000000 ) ) ;
#13469=CARTESIAN_POINT ( 'NONE',  ( 157.4999999999998579, 156.0491873085704242, -45.00000000000000000 ) ) ;
#13472=CARTESIAN_POINT ( 'NONE',  ( 158.0000000000009095, 120.6849996997183183, 45.00000000000000000 ) ) ;
#13473=VECTOR ( 'NONE', #16443, 999.9999999999998863 ) ;
#13477=ORIENTED_EDGE ( 'NONE', *, *, #8287, .F. ) ;
#13478=DIRECTION ( 'NONE',  ( 0.8916010070296935819, 0.4528218681376112165, 0.000000000000000000 ) ) ;
#13480=LINE ( 'NONE', #6439, #4483 ) ;
#13485=EDGE_CURVE ( 'NONE', #24950, #19061, #12705, .T. ) ;
#13489=ORIENTED_EDGE ( 'NONE', *, *, #758, .T. ) ;
#13490=LINE ( 'NONE', #22678, #8128 ) ;
#13494=PLANE ( 'NONE',  #6871 ) ;
#13496=CARTESIAN_POINT ( 'NONE',  ( 157.4999999999996589, 278.9350626764145318, 45.00000000000000000 ) ) ;
#13500=CARTESIAN_POINT ( 'NONE',  ( 157.9999999999997726, 246.5866250825770294, -45.00000000000000000 ) ) ;
#13501=DIRECTION ( 'NONE',  ( -0.8916010070293584056, -0.4528218681382712996, 0.000000000000000000 ) ) ;
#13502=CARTESIAN_POINT ( 'NONE',  ( 158.0000000000013358, 78.55899957960562574, 45.00000000000000000 ) ) ;
#13503=DIRECTION ( 'NONE',  ( 0.4528218681374719945, 0.8916010070297644141, -0.000000000000000000 ) ) ;
#13504=DIRECTION ( 'NONE',  ( 0.8916010070295715684, -0.4528218681378516353, 0.000000000000000000 ) ) ;
#13505=LINE ( 'NONE', #7178, #6360 ) ;
#13508=DIRECTION ( 'NONE',  ( -0.000000000000000000, -0.000000000000000000, -1.000000000000000000 ) ) ;
#13509=ORIENTED_EDGE ( 'NONE', *, *, #22707, .T. ) ;
#13512=CARTESIAN_POINT ( 'NONE',  ( 157.9999999999996589, 274.1732501651540588, -45.00000000000000000 ) ) ;
#13524=EDGE_CURVE ( 'NONE', #12071, #15387, #10677, .T. ) ;
#13526=ORIENTED_EDGE ( 'NONE', *, *, #2985, .T. ) ;
#13528=VECTOR ( 'NONE', #18115, 1000.000000000000000 ) ;
#13532=VECTOR ( 'NONE', #20586, 1000.000000000000000 ) ;
#13534=DIRECTION ( 'NONE',  ( -0.000000000000000000, -0.000000000000000000, -1.000000000000000000 ) ) ;
#13539=CARTESIAN_POINT ( 'NONE',  ( 158.0000000000000568, 201.4448749474510407, 45.00000000000000000 ) ) ;
#13546=EDGE_CURVE ( 'NONE', #19895, #12172, #13129, .T. ) ;
#13551=ORIENTED_EDGE ( 'NONE', *, *, #11461, .F. ) ;
#13553=CARTESIAN_POINT ( 'NONE',  ( 158.0000000000010516, 105.6377496546760568, 45.00000000000000000 ) ) ;
#13558=EDGE_LOOP ( 'NONE', ( #11005, #8112, #4467, #7781 ) ) ;
#13559=DIRECTION ( 'NONE',  ( 0.4528218681373520904, 0.8916010070298252543, -0.000000000000000000 ) ) ;
#13560=ADVANCED_FACE ( 'NONE', ( #24035 ), #21872, .F. ) ;
#13561=CARTESIAN_POINT ( 'NONE',  ( 158.0000000000006253, 146.2716247822957598, 45.00000000000000000 ) ) ;
#13562=ORIENTED_EDGE ( 'NONE', *, *, #20723, .T. ) ;
#13563=DIRECTION ( 'NONE',  ( 0.8916010070297953893, 0.4528218681374108212, 0.000000000000000000 ) ) ;
#13564=ORIENTED_EDGE ( 'NONE', *, *, #28331, .F. ) ;
#13565=CARTESIAN_POINT ( 'NONE',  ( 157.4999999999998579, 103.3838121509225090, -45.00000000000000000 ) ) ;
#13568=CARTESIAN_POINT ( 'NONE',  ( 157.4999999999998579, 171.0964373536126573, 45.00000000000000000 ) ) ;
#13574=LINE ( 'NONE', #19457, #12363 ) ;
#13577=VECTOR ( 'NONE', #22730, 1000.000000000000000 ) ;
#13582=DIRECTION ( 'NONE',  ( -0.8916010070296531698, -0.4528218681376911525, 0.000000000000000000 ) ) ;
#13593=FACE_OUTER_BOUND ( 'NONE', #22205, .T. ) ;
#13594=VERTEX_POINT ( 'NONE', #2752 ) ;
#13597=VECTOR ( 'NONE', #17892, 1000.000000000000000 ) ;
#13598=ORIENTED_EDGE ( 'NONE', *, *, #7195, .F. ) ;
#13599=EDGE_CURVE ( 'NONE', #6186, #26306, #17556, .T. ) ;
#13601=ORIENTED_EDGE ( 'NONE', *, *, #7515, .T. ) ;
#13608=DIRECTION ( 'NONE',  ( -0.000000000000000000, -0.000000000000000000, -1.000000000000000000 ) ) ;
#13609=EDGE_CURVE ( 'NONE', #14062, #152, #22442, .T. ) ;
#13617=CARTESIAN_POINT ( 'NONE',  ( 157.9999999999997442, 254.1102501050980322, -45.00000000000000000 ) ) ;
#13619=EDGE_CURVE ( 'NONE', #26072, #14776, #8796, .T. ) ;
#13620=ORIENTED_EDGE ( 'NONE', *, *, #21874, .F. ) ;
#13624=DIRECTION ( 'NONE',  ( 0.4528218681373709642, -0.8916010070298157064, 0.000000000000000000 ) ) ;
#13626=EDGE_CURVE ( 'NONE', #23386, #2647, #6924, .T. ) ;
#13628=AXIS2_PLACEMENT_3D ( 'NONE', #8687, #17441, #11277 ) ;
#13629=ORIENTED_EDGE ( 'NONE', *, *, #18162, .T. ) ;
#13630=CARTESIAN_POINT ( 'NONE',  ( 157.4999999999998295, 218.7460624962465090, -45.00000000000000000 ) ) ;
#13631=EDGE_LOOP ( 'NONE', ( #23915, #15469, #768, #13331 ) ) ;
#13632=CARTESIAN_POINT ( 'NONE',  ( 158.0000000000007390, 133.7322497447605656, -45.00000000000000000 ) ) ;
#13633=EDGE_LOOP ( 'NONE', ( #2161, #8428, #28317, #25520 ) ) ;
#13636=ORIENTED_EDGE ( 'NONE', *, *, #13454, .F. ) ;
#13637=ORIENTED_EDGE ( 'NONE', *, *, #10204, .T. ) ;
#13638=LINE ( 'NONE', #9882, #17306 ) ;
#13643=DIRECTION ( 'NONE',  ( 0.000000000000000000, -1.000000000000000000, 0.000000000000000000 ) ) ;
#13645=CARTESIAN_POINT ( 'NONE',  ( 157.9999999999997442, 249.0945000900840398, 45.00000000000000000 ) ) ;
#13649=DIRECTION ( 'NONE',  ( 0.8916010070293783896, -0.4528218681382319422, 0.000000000000000000 ) ) ;
#13651=LINE ( 'NONE', #569, #18497 ) ;
#13652=EDGE_CURVE ( 'NONE', #15187, #17412, #22154, .T. ) ;
#13656=CARTESIAN_POINT ( 'NONE',  ( 158.0000000000008527, 125.7007497147323818, -45.00000000000000000 ) ) ;
#13657=LINE ( 'NONE', #3134, #19383 ) ;
#13662=LINE ( 'NONE', #7186, #26709 ) ;
#13665=ORIENTED_EDGE ( 'NONE', *, *, #6714, .T. ) ;
#13666=ORIENTED_EDGE ( 'NONE', *, *, #422, .T. ) ;
#13670=ORIENTED_EDGE ( 'NONE', *, *, #19382, .T. ) ;
#13671=VERTEX_POINT ( 'NONE', #7219 ) ;
#13673=VECTOR ( 'NONE', #9925, 1000.000000000000227 ) ;
#13680=VECTOR ( 'NONE', #24086, 1000.000000000000000 ) ;
#13683=CARTESIAN_POINT ( 'NONE',  ( 157.9999999999999432, 211.4763749774776045, 45.00000000000000000 ) ) ;
#13686=ORIENTED_EDGE ( 'NONE', *, *, #9908, .F. ) ;
#13687=DIRECTION ( 'NONE',  ( -0.8916010070295820045, 0.4528218681378310406, 0.000000000000000000 ) ) ;
#13691=CARTESIAN_POINT ( 'NONE',  ( 158.0000000000000853, 196.4291249324366504, -45.00000000000000000 ) ) ;
#13701=CARTESIAN_POINT ( 'NONE',  ( 157.9999999999996305, 283.6968751876750616, -45.00000000000000000 ) ) ;
#13705=FACE_OUTER_BOUND ( 'NONE', #28322, .T. ) ;
#13707=VERTEX_POINT ( 'NONE', #753 ) ;
#13708=DIRECTION ( 'NONE',  ( -0.8916010070299571488, 0.4528218681370923537, 0.000000000000000000 ) ) ;
#13713=VECTOR ( 'NONE', #58, 1000.000000000000000 ) ;
#13722=ADVANCED_FACE ( 'NONE', ( #16408 ), #27575, .F. ) ;
#13724=PLANE ( 'NONE',  #15096 ) ;
#13725=DIRECTION ( 'NONE',  ( -0.000000000000000000, -0.000000000000000000, -1.000000000000000000 ) ) ;
#13726=VERTEX_POINT ( 'NONE', #18690 ) ;
#13730=VECTOR ( 'NONE', #17025, 1000.000000000000000 ) ;
#13731=DIRECTION ( 'NONE',  ( -0.8916010070294200229, -0.4528218681381501742, 0.000000000000000000 ) ) ;
#13734=ORIENTED_EDGE ( 'NONE', *, *, #10876, .T. ) ;
#13736=ORIENTED_EDGE ( 'NONE', *, *, #585, .F. ) ;
#13739=ORIENTED_EDGE ( 'NONE', *, *, #8766, .F. ) ;
#13744=FACE_OUTER_BOUND ( 'NONE', #3987, .T. ) ;
#13752=VECTOR ( 'NONE', #27946, 1000.000000000000114 ) ;
#13753=DIRECTION ( 'NONE',  ( 0.8916010070291696676, 0.4528218681386429467, 0.000000000000000000 ) ) ;
#13754=DIRECTION ( 'NONE',  ( -0.000000000000000000, -0.000000000000000000, -1.000000000000000000 ) ) ;
#13758=CARTESIAN_POINT ( 'NONE',  ( 157.9999999999998010, 236.5551250525490161, 45.00000000000000000 ) ) ;
#13761=DIRECTION ( 'NONE',  ( -0.000000000000000000, -0.000000000000000000, -1.000000000000000000 ) ) ;
#13762=CARTESIAN_POINT ( 'NONE',  ( 157.4999999999998579, 115.9231871884577174, 45.00000000000000000 ) ) ;
#13763=ORIENTED_EDGE ( 'NONE', *, *, #22716, .T. ) ;
#13765=VECTOR ( 'NONE', #1989, 1000.000000000000114 ) ;
#13768=DIRECTION ( 'NONE',  ( -0.000000000000000000, 0.000000000000000000, -1.000000000000000000 ) ) ;
#13773=CARTESIAN_POINT ( 'NONE',  ( 158.0000000000003411, 175.8582498648732440, 45.00000000000000000 ) ) ;
#13777=ORIENTED_EDGE ( 'NONE', *, *, #16658, .T. ) ;
#13782=ORIENTED_EDGE ( 'NONE', *, *, #19827, .F. ) ;
#13788=EDGE_CURVE ( 'NONE', #10864, #8063, #7643, .T. ) ;
#13790=CARTESIAN_POINT ( 'NONE',  ( 157.4999999999995453, 206.2066874587088989, -45.00000000000000000 ) ) ;
#13793=DIRECTION ( 'NONE',  ( -0.8916010070293383105, -0.4528218681383106015, 0.000000000000000000 ) ) ;
#13803=LINE ( 'NONE', #17661, #22082 ) ;
#13806=VERTEX_POINT ( 'NONE', #22588 ) ;
#13807=DIRECTION ( 'NONE',  ( 0.8916010070299171808, 0.4528218681371710685, 0.000000000000000000 ) ) ;
#13808=FACE_OUTER_BOUND ( 'NONE', #1839, .T. ) ;
#13811=VERTEX_POINT ( 'NONE', #5473 ) ;
#13815=ORIENTED_EDGE ( 'NONE', *, *, #13892, .T. ) ;
#13818=FACE_OUTER_BOUND ( 'NONE', #14110, .T. ) ;
#13820=AXIS2_PLACEMENT_3D ( 'NONE', #30, #28171, #26310 ) ;
#13821=CARTESIAN_POINT ( 'NONE',  ( 158.0000000000005400, 155.7952498048169048, -45.00000000000000000 ) ) ;
#13823=EDGE_CURVE ( 'NONE', #14497, #27805, #20563, .T. ) ;
#13826=FACE_OUTER_BOUND ( 'NONE', #28281, .T. ) ;
#13831=DIRECTION ( 'NONE',  ( -0.8916010070294909662, -0.4528218681380102306, 0.000000000000000000 ) ) ;
#13839=DIRECTION ( 'NONE',  ( 0.000000000000000000, -1.000000000000000000, 0.000000000000000000 ) ) ;
#13842=CARTESIAN_POINT ( 'NONE',  ( 157.4999999999996874, 271.4114376538935289, 45.00000000000000000 ) ) ;
#13843=DIRECTION ( 'NONE',  ( -0.8916010070293383105, -0.4528218681383106015, 0.000000000000000000 ) ) ;
#13846=ORIENTED_EDGE ( 'NONE', *, *, #12618, .F. ) ;
#13847=EDGE_CURVE ( 'NONE', #20397, #14251, #18416, .T. ) ;
#13851=DIRECTION ( 'NONE',  ( 0.000000000000000000, -1.000000000000000000, 0.000000000000000000 ) ) ;
#13852=EDGE_CURVE ( 'NONE', #7620, #17770, #10075, .T. ) ;
#13854=ORIENTED_EDGE ( 'NONE', *, *, #278, .F. ) ;
#13857=VECTOR ( 'NONE', #9559, 1000.000000000000114 ) ;
#13863=CARTESIAN_POINT ( 'NONE',  ( 158.0000000000016769, 47.95662448201407102, -45.00000000000000000 ) ) ;
#13866=ORIENTED_EDGE ( 'NONE', *, *, #11403, .F. ) ;
#13867=PLANE ( 'NONE',  #12769 ) ;
#13870=LINE ( 'NONE', #9827, #5697 ) ;
#13874=VECTOR ( 'NONE', #6386, 1000.000000000000000 ) ;
#13878=VERTEX_POINT ( 'NONE', #12667 ) ;
#13880=VECTOR ( 'NONE', #23192, 1000.000000000000227 ) ;
#13885=DIRECTION ( 'NONE',  ( -0.8916010070298157064, -0.4528218681373708532, 0.000000000000000000 ) ) ;
#13887=FACE_OUTER_BOUND ( 'NONE', #24649, .T. ) ;
#13892=EDGE_CURVE ( 'NONE', #24666, #14722, #21409, .T. ) ;
#13894=ORIENTED_EDGE ( 'NONE', *, *, #21810, .F. ) ;
#13902=VECTOR ( 'NONE', #1900, 1000.000000000000000 ) ;
#13903=LINE ( 'NONE', #25216, #23422 ) ;
#13904=CARTESIAN_POINT ( 'NONE',  ( 158.0000000000006537, 141.2558747672816821, 45.00000000000000000 ) ) ;
#13905=PLANE ( 'NONE',  #6097 ) ;
#13910=DIRECTION ( 'NONE',  ( -0.8916010070300285362, -0.4528218681369517995, 0.000000000000000000 ) ) ;
#13916=AXIS2_PLACEMENT_3D ( 'NONE', #20936, #3258, #9884 ) ;
#13921=CARTESIAN_POINT ( 'NONE',  ( 158.0000000000013642, 78.05112457209858690, 45.00000000000000000 ) ) ;
#13923=ORIENTED_EDGE ( 'NONE', *, *, #14468, .T. ) ;
#13924=VECTOR ( 'NONE', #26386, 1000.000000000000000 ) ;
#13927=ORIENTED_EDGE ( 'NONE', *, *, #9816, .T. ) ;
#13929=DIRECTION ( 'NONE',  ( 0.8916010070294498879, -0.4528218681380914434, 0.000000000000000000 ) ) ;
#13933=ADVANCED_FACE ( 'NONE', ( #8055 ), #19255, .F. ) ;
#13934=CARTESIAN_POINT ( 'NONE',  ( 157.4999999999998579, 166.0806873385985796, 45.00000000000000000 ) ) ;
#13938=DIRECTION ( 'NONE',  ( -0.000000000000000000, -0.000000000000000000, -1.000000000000000000 ) ) ;
#13940=VECTOR ( 'NONE', #14566, 1000.000000000000000 ) ;
#13942=CARTESIAN_POINT ( 'NONE',  ( 157.9999999999997726, 244.0787500750700474, 45.00000000000000000 ) ) ;
#13943=VECTOR ( 'NONE', #12345, 1000.000000000000000 ) ;
#13947=EDGE_CURVE ( 'NONE', #11388, #969, #21697, .T. ) ;
#13951=LINE ( 'NONE', #11928, #16648 ) ;
#13952=EDGE_LOOP ( 'NONE', ( #26820, #5912, #4476, #4341 ) ) ;
#13953=EDGE_LOOP ( 'NONE', ( #19681, #6164, #19230, #18419 ) ) ;
#13954=LINE ( 'NONE', #13512, #19242 ) ;
#13956=ORIENTED_EDGE ( 'NONE', *, *, #21988, .T. ) ;
#13960=LINE ( 'NONE', #9497, #9742 ) ;
#13963=VECTOR ( 'NONE', #9549, 1000.000000000000000 ) ;
#13964=ORIENTED_EDGE ( 'NONE', *, *, #9908, .T. ) ;
#13965=CARTESIAN_POINT ( 'NONE',  ( 157.4999999999998579, 65.76568703831686946, 45.00000000000000000 ) ) ;
#13970=DIRECTION ( 'NONE',  ( -0.8916010070296530587, 0.4528218681376912080, 0.000000000000000000 ) ) ;
#13972=CARTESIAN_POINT ( 'NONE',  ( 157.4999999999998579, 118.4310621959647563, -45.00000000000000000 ) ) ;
#13974=AXIS2_PLACEMENT_3D ( 'NONE', #23980, #24126, #13076 ) ;
#13975=EDGE_CURVE ( 'NONE', #4392, #17424, #3879, .T. ) ;
#13976=CARTESIAN_POINT ( 'NONE',  ( 158.0000000000003695, 171.3503748573662051, 45.00000000000000000 ) ) ;
#13978=CARTESIAN_POINT ( 'NONE',  ( 157.9999999999998579, 221.0000000000000284, 45.00000000000000000 ) ) ;
#13980=CARTESIAN_POINT ( 'NONE',  ( 157.4999999999997442, 253.8563126013445697, 45.00000000000000000 ) ) ;
#13981=ORIENTED_EDGE ( 'NONE', *, *, #16393, .F. ) ;
#13982=EDGE_CURVE ( 'NONE', #11176, #14709, #20106, .T. ) ;
#13984=EDGE_CURVE ( 'NONE', #18505, #5660, #6468, .T. ) ;
#13991=CARTESIAN_POINT ( 'NONE',  ( 158.0000000000015632, 55.98812451204224061, 45.00000000000000000 ) ) ;
#13995=DIRECTION ( 'NONE',  ( -0.000000000000000000, -0.000000000000000000, -1.000000000000000000 ) ) ;
#13999=ORIENTED_EDGE ( 'NONE', *, *, #26497, .T. ) ;
#14001=LINE ( 'NONE', #25172, #1968 ) ;
#14002=CARTESIAN_POINT ( 'NONE',  ( 157.4999999999998579, 221.2539375037535194, 45.00000000000000000 ) ) ;
#14005=DIRECTION ( 'NONE',  ( 0.8916010070293510781, -0.4528218681382856770, 0.000000000000000000 ) ) ;
#14006=LINE ( 'NONE', #11418, #485 ) ;
#14007=LINE ( 'NONE', #3198, #5637 ) ;
#14013=EDGE_LOOP ( 'NONE', ( #4840, #28004, #16144, #18969 ) ) ;
#14017=EDGE_CURVE ( 'NONE', #15637, #10398, #10924, .T. ) ;
#14019=EDGE_CURVE ( 'NONE', #24937, #17953, #4587, .T. ) ;
#14021=DIRECTION ( 'NONE',  ( 0.8916010070293783896, -0.4528218681382319422, 0.000000000000000000 ) ) ;
#14023=ORIENTED_EDGE ( 'NONE', *, *, #18403, .T. ) ;
#14031=VERTEX_POINT ( 'NONE', #6746 ) ;
#14032=DIRECTION ( 'NONE',  ( -0.8916010070293383105, -0.4528218681383106015, 0.000000000000000000 ) ) ;
#14033=ORIENTED_EDGE ( 'NONE', *, *, #7094, .F. ) ;
#14037=VECTOR ( 'NONE', #5260, 1000.000000000000000 ) ;
#14038=FACE_OUTER_BOUND ( 'NONE', #392, .T. ) ;
#14044=LINE ( 'NONE', #18615, #21212 ) ;
#14045=LINE ( 'NONE', #9580, #11324 ) ;
#14050=ORIENTED_EDGE ( 'NONE', *, *, #422, .F. ) ;
#14058=AXIS2_PLACEMENT_3D ( 'NONE', #6667, #10984, #20018 ) ;
#14059=CARTESIAN_POINT ( 'NONE',  ( 157.4999999999998579, 78.30506207585207790, -45.00000000000000000 ) ) ;
#14062=VERTEX_POINT ( 'NONE', #26091 ) ;
#14067=DIRECTION ( 'NONE',  ( 0.8916010070297852863, 0.4528218681374306942, 0.000000000000000000 ) ) ;
#14074=EDGE_CURVE ( 'NONE', #5015, #14898, #23953, .T. ) ;
#14075=CARTESIAN_POINT ( 'NONE',  ( 157.9999999999997158, 256.6181251126050711, 45.00000000000000000 ) ) ;
#14078=VECTOR ( 'NONE', #4825, 1000.000000000000000 ) ;
#14086=VERTEX_POINT ( 'NONE', #24324 ) ;
#14088=LINE ( 'NONE', #25126, #25342 ) ;
#14089=VERTEX_POINT ( 'NONE', #26055 ) ;
#14093=ORIENTED_EDGE ( 'NONE', *, *, #3507, .T. ) ;
#14097=PLANE ( 'NONE',  #20072 ) ;
#14099=DIRECTION ( 'NONE',  ( 0.8916010070293710621, -0.4528218681382463195, 0.000000000000000000 ) ) ;
#14100=ADVANCED_FACE ( 'NONE', ( #22176 ), #6798, .F. ) ;
#14101=DIRECTION ( 'NONE',  ( -0.8916010070293584056, 0.4528218681382713551, 0.000000000000000000 ) ) ;
#14102=DIRECTION ( 'NONE',  ( 0.8916010070297542001, -0.4528218681374919230, 0.000000000000000000 ) ) ;
#14103=VECTOR ( 'NONE', #19123, 1000.000000000000227 ) ;
#14106=LINE ( 'NONE', #18407, #20123 ) ;
#14109=DIRECTION ( 'NONE',  ( 0.000000000000000000, -1.000000000000000000, 0.000000000000000000 ) ) ;
#14110=EDGE_LOOP ( 'NONE', ( #9165, #18594, #1392, #19185 ) ) ;
#14116=VERTEX_POINT ( 'NONE', #8815 ) ;
#14120=CARTESIAN_POINT ( 'NONE',  ( 158.0000000000009663, 113.1613746771971876, -45.00000000000000000 ) ) ;
#14122=AXIS2_PLACEMENT_3D ( 'NONE', #11485, #11633, #11337 ) ;
#14123=ORIENTED_EDGE ( 'NONE', *, *, #3333, .F. ) ;
#14129=ORIENTED_EDGE ( 'NONE', *, *, #12256, .T. ) ;
#14130=LINE ( 'NONE', #4917, #23368 ) ;
#14132=CARTESIAN_POINT ( 'NONE',  ( 158.0000000000008242, 128.2086247222394206, 45.00000000000000000 ) ) ;
#14134=PLANE ( 'NONE',  #21346 ) ;
#14135=EDGE_CURVE ( 'NONE', #5095, #83, #10838, .T. ) ;
#14138=CARTESIAN_POINT ( 'NONE',  ( 157.4999999999994884, 211.2224374737238577, 45.00000000000000000 ) ) ;
#14139=CARTESIAN_POINT ( 'NONE',  ( 157.4999999999997158, 261.3799376238655441, 45.00000000000000000 ) ) ;
#14140=DIRECTION ( 'NONE',  ( 0.4528218681372321863, 0.8916010070298862056, -0.000000000000000000 ) ) ;
#14141=VECTOR ( 'NONE', #6307, 1000.000000000000000 ) ;
#14142=ORIENTED_EDGE ( 'NONE', *, *, #22893, .F. ) ;
#14143=PLANE ( 'NONE',  #9084 ) ;
#14146=CARTESIAN_POINT ( 'NONE',  ( 157.4999999999998579, 168.5885623461056184, 45.00000000000000000 ) ) ;
#14148=ORIENTED_EDGE ( 'NONE', *, *, #4426, .T. ) ;
#14155=DIRECTION ( 'NONE',  ( 0.8916010070299774659, -0.4528218681370523302, 0.000000000000000000 ) ) ;
#14162=LINE ( 'NONE', #2949, #24641 ) ;
#14163=VERTEX_POINT ( 'NONE', #17157 ) ;
#14170=EDGE_CURVE ( 'NONE', #28088, #14580, #23765, .T. ) ;
#14171=CARTESIAN_POINT ( 'NONE',  ( 157.9999999999997158, 258.6181251126050711, 45.00000000000000000 ) ) ;
#14178=DIRECTION ( 'NONE',  ( -0.000000000000000000, -0.000000000000000000, -1.000000000000000000 ) ) ;
#14181=ORIENTED_EDGE ( 'NONE', *, *, #7673, .T. ) ;
#14186=CARTESIAN_POINT ( 'NONE',  ( 157.4999999999998579, 188.6515624061619576, -45.00000000000000000 ) ) ;
#14189=DIRECTION ( 'NONE',  ( 1.000000000000000000, 0.000000000000000000, -0.000000000000000000 ) ) ;
#14191=EDGE_CURVE ( 'NONE', #10929, #21594, #21606, .T. ) ;
#14193=ORIENTED_EDGE ( 'NONE', *, *, #22375, .T. ) ;
#14195=VERTEX_POINT ( 'NONE', #4491 ) ;
#14197=ORIENTED_EDGE ( 'NONE', *, *, #13626, .T. ) ;
#14201=LINE ( 'NONE', #3541, #15976 ) ;
#14202=CARTESIAN_POINT ( 'NONE',  ( 157.4999999999998579, 90.84443711338730054, -45.00000000000000000 ) ) ;
#14204=EDGE_CURVE ( 'NONE', #2585, #20893, #2338, .T. ) ;
#14209=CARTESIAN_POINT ( 'NONE',  ( 157.9999999999996874, 264.1417501351260171, -45.00000000000000000 ) ) ;
#14213=CARTESIAN_POINT ( 'NONE',  ( 158.0000000000008242, 128.2086247222394206, 45.00000000000000000 ) ) ;
#14217=ORIENTED_EDGE ( 'NONE', *, *, #5592, .F. ) ;
#14218=VECTOR ( 'NONE', #20559, 1000.000000000000227 ) ;
#14219=LINE ( 'NONE', #26854, #26562 ) ;
#14225=AXIS2_PLACEMENT_3D ( 'NONE', #10149, #1517, #27649 ) ;
#14226=PLANE ( 'NONE',  #21669 ) ;
#14232=EDGE_CURVE ( 'NONE', #13878, #3041, #10376, .T. ) ;
#14243=EDGE_CURVE ( 'NONE', #25694, #16854, #3195, .T. ) ;
#14250=PLANE ( 'NONE',  #3388 ) ;
#14251=VERTEX_POINT ( 'NONE', #1049 ) ;
#14253=VECTOR ( 'NONE', #21041, 1000.000000000000000 ) ;
#14255=ORIENTED_EDGE ( 'NONE', *, *, #6109, .F. ) ;
#14257=EDGE_LOOP ( 'NONE', ( #16835, #26327, #22935, #1110 ) ) ;
#14259=ADVANCED_FACE ( 'NONE', ( #6453 ), #1188, .F. ) ;
#14261=CARTESIAN_POINT ( 'NONE',  ( 157.4999999999997158, 263.8878126313725829, 45.00000000000000000 ) ) ;
#14262=ORIENTED_EDGE ( 'NONE', *, *, #5594, .T. ) ;
#14263=ORIENTED_EDGE ( 'NONE', *, *, #26347, .T. ) ;
#14265=LINE ( 'NONE', #9530, #632 ) ;
#14267=ORIENTED_EDGE ( 'NONE', *, *, #22948, .T. ) ;
#14271=EDGE_CURVE ( 'NONE', #16287, #10929, #18852, .T. ) ;
#14273=ADVANCED_FACE ( 'NONE', ( #5779 ), #14276, .F. ) ;
#14274=CARTESIAN_POINT ( 'NONE',  ( 157.4999999999998579, 65.76568703831686946, -45.00000000000000000 ) ) ;
#14276=PLANE ( 'NONE',  #22304 ) ;
#14278=LINE ( 'NONE', #23447, #27117 ) ;
#14282=FACE_OUTER_BOUND ( 'NONE', #1245, .T. ) ;
#14283=DIRECTION ( 'NONE',  ( -0.000000000000000000, 0.000000000000000000, -1.000000000000000000 ) ) ;
#14291=CARTESIAN_POINT ( 'NONE',  ( 157.4999999999997442, 253.8563126013445697, 45.00000000000000000 ) ) ;
#14293=ORIENTED_EDGE ( 'NONE', *, *, #19029, .T. ) ;
#14294=CARTESIAN_POINT ( 'NONE',  ( 158.0000000000005400, 158.3031248123239436, 45.00000000000000000 ) ) ;
#14299=ORIENTED_EDGE ( 'NONE', *, *, #19137, .F. ) ;
#14301=DIRECTION ( 'NONE',  ( 0.8916010070295922185, -0.4528218681378110566, 0.000000000000000000 ) ) ;
#14302=ORIENTED_EDGE ( 'NONE', *, *, #6743, .F. ) ;
#14306=CARTESIAN_POINT ( 'NONE',  ( 157.9999999999998295, 224.0157500150140208, 45.00000000000000000 ) ) ;
#14307=EDGE_CURVE ( 'NONE', #18107, #25491, #21287, .T. ) ;
#14309=CARTESIAN_POINT ( 'NONE',  ( 157.9999999999998579, 219.0000000000000284, 45.00000000000000000 ) ) ;
#14311=LINE ( 'NONE', #16194, #19076 ) ;
#14313=VECTOR ( 'NONE', #4789, 1000.000000000000000 ) ;
#14314=DIRECTION ( 'NONE',  ( -0.000000000000000000, -0.000000000000000000, -1.000000000000000000 ) ) ;
#14318=CARTESIAN_POINT ( 'NONE',  ( 158.0000000000001421, 193.4133749174225443, 45.00000000000000000 ) ) ;
#14326=EDGE_CURVE ( 'NONE', #4287, #15447, #1328, .T. ) ;
#14328=CARTESIAN_POINT ( 'NONE',  ( 157.9999999999998010, 233.5393750375350237, 45.00000000000000000 ) ) ;
#14330=DIRECTION ( 'NONE',  ( -0.8916010070299369428, 0.4528218681371322663, 0.000000000000000000 ) ) ;
#14332=EDGE_CURVE ( 'NONE', #21244, #27897, #7024, .T. ) ;
#14336=ORIENTED_EDGE ( 'NONE', *, *, #21385, .T. ) ;
#14343=AXIS2_PLACEMENT_3D ( 'NONE', #9053, #26563, #15672 ) ;
#14345=LINE ( 'NONE', #11779, #15255 ) ;
#14346=DIRECTION ( 'NONE',  ( -0.8916010070296940260, -0.4528218681376106058, 0.000000000000000000 ) ) ;
#14347=DIRECTION ( 'NONE',  ( 0.4528218681378710087, -0.8916010070295616874, 0.000000000000000000 ) ) ;
#14359=CARTESIAN_POINT ( 'NONE',  ( 158.0000000000002274, 185.8897498949014278, 45.00000000000000000 ) ) ;
#14364=ADVANCED_FACE ( 'NONE', ( #15808 ), #6879, .F. ) ;
#14365=FACE_OUTER_BOUND ( 'NONE', #17605, .T. ) ;
#14369=VERTEX_POINT ( 'NONE', #21830 ) ;
#14373=AXIS2_PLACEMENT_3D ( 'NONE', #20300, #5066, #24760 ) ;
#14374=CARTESIAN_POINT ( 'NONE',  ( 158.0000000000006537, 143.2558747672816821, -45.00000000000000000 ) ) ;
#14380=CARTESIAN_POINT ( 'NONE',  ( 157.4999999999998579, 98.36806213590843129, -45.00000000000000000 ) ) ;
#14385=LINE ( 'NONE', #23143, #10154 ) ;
#14386=CARTESIAN_POINT ( 'NONE',  ( 158.0000000000014211, 73.03537455708450921, 45.00000000000000000 ) ) ;
#14390=EDGE_CURVE ( 'NONE', #5230, #22744, #18093, .T. ) ;
#14392=EDGE_CURVE ( 'NONE', #3701, #26778, #8897, .T. ) ;
#14399=FACE_OUTER_BOUND ( 'NONE', #189, .T. ) ;
#14401=EDGE_LOOP ( 'NONE', ( #330, #24779, #23834, #23579 ) ) ;
#14402=ORIENTED_EDGE ( 'NONE', *, *, #26309, .T. ) ;
#14405=CARTESIAN_POINT ( 'NONE',  ( 158.0000000000010516, 105.6377496546760568, 45.00000000000000000 ) ) ;
#14408=EDGE_LOOP ( 'NONE', ( #10582, #4727, #18661, #23121 ) ) ;
#14410=LINE ( 'NONE', #16146, #17571 ) ;
#14414=DIRECTION ( 'NONE',  ( -0.000000000000000000, -0.000000000000000000, -1.000000000000000000 ) ) ;
#14419=EDGE_CURVE ( 'NONE', #14195, #13314, #9041, .T. ) ;
#14420=VERTEX_POINT ( 'NONE', #11495 ) ;
#14422=CARTESIAN_POINT ( 'NONE',  ( 158.0000000000012790, 85.57474959461971764, 45.00000000000000000 ) ) ;
#14424=CARTESIAN_POINT ( 'NONE',  ( 158.0000000000013642, 78.05112457209858690, 45.00000000000000000 ) ) ;
#14425=VERTEX_POINT ( 'NONE', #17654 ) ;
#14431=LINE ( 'NONE', #5797, #19961 ) ;
#14432=ORIENTED_EDGE ( 'NONE', *, *, #14866, .T. ) ;
#14433=FACE_OUTER_BOUND ( 'NONE', #11290, .T. ) ;
#14434=CARTESIAN_POINT ( 'NONE',  ( 157.9999999999998579, 221.5078750075070104, -45.00000000000000000 ) ) ;
#14438=LINE ( 'NONE', #14574, #13880 ) ;
#14444=ORIENTED_EDGE ( 'NONE', *, *, #11508, .T. ) ;
#14445=ORIENTED_EDGE ( 'NONE', *, *, #24047, .T. ) ;
#14448=CARTESIAN_POINT ( 'NONE',  ( 158.0000000000007674, 133.2243747372535267, 45.00000000000000000 ) ) ;
#14449=CARTESIAN_POINT ( 'NONE',  ( 157.9999999999998295, 226.5236250225210313, 45.00000000000000000 ) ) ;
#14451=VECTOR ( 'NONE', #6170, 1000.000000000000000 ) ;
#14455=LINE ( 'NONE', #1371, #7923 ) ;
#14456=CARTESIAN_POINT ( 'NONE',  ( 158.0000000000005969, 148.7794997898028271, 45.00000000000000000 ) ) ;
#14460=ORIENTED_EDGE ( 'NONE', *, *, #7863, .F. ) ;
#14466=ORIENTED_EDGE ( 'NONE', *, *, #16241, .T. ) ;
#14468=EDGE_CURVE ( 'NONE', #8924, #5313, #2275, .T. ) ;
#14470=ORIENTED_EDGE ( 'NONE', *, *, #17787, .F. ) ;
#14473=VECTOR ( 'NONE', #9291, 1000.000000000000000 ) ;
#14474=VECTOR ( 'NONE', #4826, 1000.000000000000000 ) ;
#14475=ORIENTED_EDGE ( 'NONE', *, *, #24020, .F. ) ;
#14479=ORIENTED_EDGE ( 'NONE', *, *, #9420, .T. ) ;
#14480=DIRECTION ( 'NONE',  ( 0.4528218681382713551, 0.8916010070293584056, -0.000000000000000000 ) ) ;
#14481=EDGE_CURVE ( 'NONE', #26306, #21594, #4716, .T. ) ;
#14486=LINE ( 'NONE', #19205, #27963 ) ;
#14487=LINE ( 'NONE', #11918, #6345 ) ;
#14489=DIRECTION ( 'NONE',  ( -0.000000000000000000, -0.000000000000000000, -1.000000000000000000 ) ) ;
#14491=DIRECTION ( 'NONE',  ( -0.000000000000000000, 0.000000000000000000, -1.000000000000000000 ) ) ;
#14492=EDGE_CURVE ( 'NONE', #10929, #15393, #23106, .T. ) ;
#14495=CARTESIAN_POINT ( 'NONE',  ( 158.0000000000006253, 148.2716247822957882, 45.00000000000000000 ) ) ;
#14497=VERTEX_POINT ( 'NONE', #18234 ) ;
#14500=AXIS2_PLACEMENT_3D ( 'NONE', #11346, #26547, #24549 ) ;
#14501=VERTEX_POINT ( 'NONE', #981 ) ;
#14502=VERTEX_POINT ( 'NONE', #10032 ) ;
#14511=ORIENTED_EDGE ( 'NONE', *, *, #23785, .T. ) ;
#14512=VECTOR ( 'NONE', #3178, 1000.000000000000000 ) ;
#14515=VECTOR ( 'NONE', #27230, 1000.000000000000000 ) ;
#14517=EDGE_CURVE ( 'NONE', #18450, #26868, #26983, .T. ) ;
#14522=DIRECTION ( 'NONE',  ( -0.8916010070293783896, -0.4528218681382319422, 0.000000000000000000 ) ) ;
#14525=CARTESIAN_POINT ( 'NONE',  ( 158.0000000000000000, 208.4606249624626457, -45.00000000000000000 ) ) ;
#14527=ORIENTED_EDGE ( 'NONE', *, *, #25944, .F. ) ;
#14528=VECTOR ( 'NONE', #3221, 1000.000000000000114 ) ;
#14531=CARTESIAN_POINT ( 'NONE',  ( 157.9999999999997442, 251.6023750975910218, 45.00000000000000000 ) ) ;
#14534=ORIENTED_EDGE ( 'NONE', *, *, #27910, .F. ) ;
#14538=CARTESIAN_POINT ( 'NONE',  ( 157.9999999999996874, 268.6496251426330559, 45.00000000000000000 ) ) ;
#14539=ORIENTED_EDGE ( 'NONE', *, *, #13382, .T. ) ;
#14540=ORIENTED_EDGE ( 'NONE', *, *, #25436, .T. ) ;
#14541=CARTESIAN_POINT ( 'NONE',  ( 157.4999999999998579, 198.6830624361901414, -45.00000000000000000 ) ) ;
#14542=DIRECTION ( 'NONE',  ( -0.000000000000000000, -0.000000000000000000, -1.000000000000000000 ) ) ;
#14547=EDGE_LOOP ( 'NONE', ( #25451, #4879, #829, #6490 ) ) ;
#14548=VECTOR ( 'NONE', #27585, 1000.000000000000227 ) ;
#14553=DIRECTION ( 'NONE',  ( 0.8916010070293783896, -0.4528218681382319422, 0.000000000000000000 ) ) ;
#14555=CARTESIAN_POINT ( 'NONE',  ( 158.0000000000009663, 115.6692496847042264, 45.00000000000000000 ) ) ;
#14557=DIRECTION ( 'NONE',  ( -0.000000000000000000, -0.000000000000000000, -1.000000000000000000 ) ) ;
#14561=DIRECTION ( 'NONE',  ( 1.000000000000000000, 0.000000000000000000, -0.000000000000000000 ) ) ;
#14564=LINE ( 'NONE', #25602, #20601 ) ;
#14566=DIRECTION ( 'NONE',  ( -0.000000000000000000, -0.000000000000000000, -1.000000000000000000 ) ) ;
#14568=LINE ( 'NONE', #18455, #27290 ) ;
#14572=ORIENTED_EDGE ( 'NONE', *, *, #19305, .F. ) ;
#14574=CARTESIAN_POINT ( 'NONE',  ( 157.9999999999998010, 231.5393750375350237, 45.00000000000000000 ) ) ;
#14575=CARTESIAN_POINT ( 'NONE',  ( 157.9999999999997158, 263.6338751276190351, -45.00000000000000000 ) ) ;
#14576=ORIENTED_EDGE ( 'NONE', *, *, #10005, .F. ) ;
#14579=EDGE_CURVE ( 'NONE', #22232, #3081, #27393, .T. ) ;
#14580=VERTEX_POINT ( 'NONE', #3266 ) ;
#14583=ORIENTED_EDGE ( 'NONE', *, *, #10364, .T. ) ;
#14588=CARTESIAN_POINT ( 'NONE',  ( 158.0000000000006821, 140.7479997597746433, -45.00000000000000000 ) ) ;
#14589=DIRECTION ( 'NONE',  ( 0.000000000000000000, -1.000000000000000000, 0.000000000000000000 ) ) ;
#14590=DIRECTION ( 'NONE',  ( 0.8916010070293584056, -0.4528218681382712996, 0.000000000000000000 ) ) ;
#14593=CARTESIAN_POINT ( 'NONE',  ( 158.0000000000008811, 121.1928747072253572, 45.00000000000000000 ) ) ;
#14594=PLANE ( 'NONE',  #3259 ) ;
#14595=LINE ( 'NONE', #21191, #9586 ) ;
#14602=DIRECTION ( 'NONE',  ( 0.8916010070296023216, -0.4528218681377911281, 0.000000000000000000 ) ) ;
#14604=VECTOR ( 'NONE', #18096, 1000.000000000000114 ) ;
#14606=VERTEX_POINT ( 'NONE', #3691 ) ;
#14607=CARTESIAN_POINT ( 'NONE',  ( 158.0000000000012790, 85.57474959461971764, 45.00000000000000000 ) ) ;
#14609=ORIENTED_EDGE ( 'NONE', *, *, #3016, .F. ) ;
#14612=ADVANCED_FACE ( 'NONE', ( #16642 ), #23669, .F. ) ;
#14614=ORIENTED_EDGE ( 'NONE', *, *, #41, .F. ) ;
#14616=DIRECTION ( 'NONE',  ( 0.8916010070299977830, -0.4528218681370124177, 0.000000000000000000 ) ) ;
#14618=VECTOR ( 'NONE', #24735, 1000.000000000000114 ) ;
#14624=EDGE_CURVE ( 'NONE', #7082, #15954, #5715, .T. ) ;
#14626=ADVANCED_FACE ( 'NONE', ( #5995 ), #24602, .F. ) ;
#14628=AXIS2_PLACEMENT_3D ( 'NONE', #4492, #2339, #21361 ) ;
#14631=LINE ( 'NONE', #14774, #21005 ) ;
#14633=ORIENTED_EDGE ( 'NONE', *, *, #20672, .T. ) ;
#14642=ORIENTED_EDGE ( 'NONE', *, *, #26575, .F. ) ;
#14644=ORIENTED_EDGE ( 'NONE', *, *, #11095, .T. ) ;
#14646=ORIENTED_EDGE ( 'NONE', *, *, #2794, .F. ) ;
#14647=ADVANCED_FACE ( 'NONE', ( #2102 ), #2382, .F. ) ;
#14650=CARTESIAN_POINT ( 'NONE',  ( 158.0000000000002842, 180.8739998798873501, -45.00000000000000000 ) ) ;
#14653=DIRECTION ( 'NONE',  ( 0.8916010070296327417, 0.4528218681377311206, 0.000000000000000000 ) ) ;
#14662=LINE ( 'NONE', #19107, #25277 ) ;
#14663=DIRECTION ( 'NONE',  ( 0.8916010070298151513, -0.4528218681373720744, 0.000000000000000000 ) ) ;
#14664=VERTEX_POINT ( 'NONE', #2240 ) ;
#14665=CARTESIAN_POINT ( 'NONE',  ( 157.4999999999998579, 133.4783122410070462, 45.00000000000000000 ) ) ;
#14666=AXIS2_PLACEMENT_3D ( 'NONE', #14806, #13210, #17785 ) ;
#14668=ORIENTED_EDGE ( 'NONE', *, *, #14517, .T. ) ;
#14670=ORIENTED_EDGE ( 'NONE', *, *, #3517, .F. ) ;
#14672=ORIENTED_EDGE ( 'NONE', *, *, #22006, .T. ) ;
#14673=EDGE_CURVE ( 'NONE', #12815, #19423, #17760, .T. ) ;
#14674=DIRECTION ( 'NONE',  ( -0.8916010070298759915, 0.4528218681372521703, 0.000000000000000000 ) ) ;
#14675=CIRCLE ( 'NONE', #8233, 6.000000000000005329 ) ;
#14678=ADVANCED_FACE ( 'NONE', ( #22217 ), #6701, .F. ) ;
#14679=ORIENTED_EDGE ( 'NONE', *, *, #13599, .T. ) ;
#14680=DIRECTION ( 'NONE',  ( -0.8916010070299477119, -0.4528218681371110610, 0.000000000000000000 ) ) ;
#14685=ORIENTED_EDGE ( 'NONE', *, *, #19597, .F. ) ;
#14692=LINE ( 'NONE', #10098, #7755 ) ;
#14693=DIRECTION ( 'NONE',  ( -0.000000000000000000, 0.000000000000000000, -1.000000000000000000 ) ) ;
#14700=DIRECTION ( 'NONE',  ( -0.000000000000000000, 0.000000000000000000, -1.000000000000000000 ) ) ;
#14701=LINE ( 'NONE', #10813, #24974 ) ;
#14702=ORIENTED_EDGE ( 'NONE', *, *, #735, .F. ) ;
#14704=VECTOR ( 'NONE', #926, 1000.000000000000114 ) ;
#14707=DIRECTION ( 'NONE',  ( 1.000000000000000000, 0.000000000000000000, -0.000000000000000000 ) ) ;
#14709=VERTEX_POINT ( 'NONE', #247 ) ;
#14710=LINE ( 'NONE', #10120, #77 ) ;
#14711=DIRECTION ( 'NONE',  ( -0.000000000000000000, -0.000000000000000000, -1.000000000000000000 ) ) ;
#14716=LINE ( 'NONE', #15001, #1906 ) ;
#14721=CARTESIAN_POINT ( 'NONE',  ( 158.0000000000011653, 93.60624962464788723, -45.00000000000000000 ) ) ;
#14722=VERTEX_POINT ( 'NONE', #11313 ) ;
#14724=ORIENTED_EDGE ( 'NONE', *, *, #25843, .F. ) ;
#14726=CARTESIAN_POINT ( 'NONE',  ( 158.0000000000013074, 83.06687458711267880, 45.00000000000000000 ) ) ;
#14728=DIRECTION ( 'NONE',  ( -0.000000000000000000, -0.000000000000000000, -1.000000000000000000 ) ) ;
#14730=CARTESIAN_POINT ( 'NONE',  ( 157.4999999999998579, 161.0649373235845019, -45.00000000000000000 ) ) ;
#14735=FACE_OUTER_BOUND ( 'NONE', #3064, .T. ) ;
#14736=CARTESIAN_POINT ( 'NONE',  ( 157.4999999999998579, 221.2539375037535194, 45.00000000000000000 ) ) ;
#14741=EDGE_CURVE ( 'NONE', #8883, #3705, #2522, .T. ) ;
#14742=EDGE_CURVE ( 'NONE', #13433, #8883, #26657, .T. ) ;
#14744=FACE_OUTER_BOUND ( 'NONE', #25653, .T. ) ;
#14747=DIRECTION ( 'NONE',  ( -0.8916010070293383105, -0.4528218681383106015, 0.000000000000000000 ) ) ;
#14750=VECTOR ( 'NONE', #19538, 1000.000000000000000 ) ;
#14752=ORIENTED_EDGE ( 'NONE', *, *, #28046, .F. ) ;
#14753=ADVANCED_FACE ( 'NONE', ( #17334 ), #4401, .F. ) ;
#14754=DIRECTION ( 'NONE',  ( 0.8916010070299369428, -0.4528218681371322663, 0.000000000000000000 ) ) ;
#14755=VERTEX_POINT ( 'NONE', #24945 ) ;
#14758=EDGE_LOOP ( 'NONE', ( #6291, #2544, #6218, #8072 ) ) ;
#14759=VERTEX_POINT ( 'NONE', #24805 ) ;
#14761=CARTESIAN_POINT ( 'NONE',  ( 158.0000000000005116, 158.8109998198309825, -45.00000000000000000 ) ) ;
#14762=DIRECTION ( 'NONE',  ( 0.4528218681377710886, 0.8916010070296124246, -0.000000000000000000 ) ) ;
#14771=DIRECTION ( 'NONE',  ( 1.000000000000000000, -0.000000000000000000, -0.000000000000000000 ) ) ;
#14772=PLANE ( 'NONE',  #28199 ) ;
#14774=CARTESIAN_POINT ( 'NONE',  ( 158.0000000000017337, 42.94087446699998623, -45.00000000000000000 ) ) ;
#14775=CARTESIAN_POINT ( 'NONE',  ( 157.4999999999998295, 231.2854375337815327, 45.00000000000000000 ) ) ;
#14776=VERTEX_POINT ( 'NONE', #22795 ) ;
#14782=ORIENTED_EDGE ( 'NONE', *, *, #17402, .T. ) ;
#14785=ORIENTED_EDGE ( 'NONE', *, *, #3021, .T. ) ;
#14787=VECTOR ( 'NONE', #10962, 1000.000000000000114 ) ;
#14789=ORIENTED_EDGE ( 'NONE', *, *, #27927, .T. ) ;
#14792=EDGE_LOOP ( 'NONE', ( #20265, #25743, #25519, #21522 ) ) ;
#14794=ORIENTED_EDGE ( 'NONE', *, *, #18841, .T. ) ;
#14795=LINE ( 'NONE', #1987, #13203 ) ;
#14799=VECTOR ( 'NONE', #25078, 1000.000000000000000 ) ;
#14806=CARTESIAN_POINT ( 'NONE',  ( 157.4999999999998579, 151.0334372935563465, 45.00000000000000000 ) ) ;
#14809=EDGE_CURVE ( 'NONE', #16142, #14865, #14045, .T. ) ;
#14819=EDGE_LOOP ( 'NONE', ( #1108, #15151, #21581, #24492 ) ) ;
#14820=VECTOR ( 'NONE', #2769, 1000.000000000000000 ) ;
#14824=AXIS2_PLACEMENT_3D ( 'NONE', #13227, #6605, #17662 ) ;
#14825=DIRECTION ( 'NONE',  ( 0.4528218681383106015, -0.8916010070293384215, 0.000000000000000000 ) ) ;
#14828=VECTOR ( 'NONE', #13504, 1000.000000000000000 ) ;
#14829=ORIENTED_EDGE ( 'NONE', *, *, #22761, .F. ) ;
#14830=DIRECTION ( 'NONE',  ( 0.4528218681383106015, -0.8916010070293384215, 0.000000000000000000 ) ) ;
#14834=ORIENTED_EDGE ( 'NONE', *, *, #13982, .T. ) ;
#14840=LINE ( 'NONE', #3758, #15039 ) ;
#14842=VECTOR ( 'NONE', #24320, 1000.000000000000000 ) ;
#14848=CARTESIAN_POINT ( 'NONE',  ( 158.0000000000003695, 171.3503748573662051, -45.00000000000000000 ) ) ;
#14849=EDGE_CURVE ( 'NONE', #17961, #24788, #18481, .T. ) ;
#14850=FACE_OUTER_BOUND ( 'NONE', #27381, .T. ) ;
#14853=LINE ( 'NONE', #5927, #26798 ) ;
#14858=CARTESIAN_POINT ( 'NONE',  ( 158.0000000000012506, 86.08262460212675649, 45.00000000000000000 ) ) ;
#14860=DIRECTION ( 'NONE',  ( 1.000000000000000000, 0.000000000000000000, 0.000000000000000000 ) ) ;
#14862=VERTEX_POINT ( 'NONE', #679 ) ;
#14865=VERTEX_POINT ( 'NONE', #18058 ) ;
#14866=EDGE_CURVE ( 'NONE', #16038, #19152, #1089, .T. ) ;
#14867=VECTOR ( 'NONE', #22573, 1000.000000000000227 ) ;
#14870=ORIENTED_EDGE ( 'NONE', *, *, #13609, .T. ) ;
#14872=ORIENTED_EDGE ( 'NONE', *, *, #1960, .F. ) ;
#14875=CARTESIAN_POINT ( 'NONE',  ( 158.0000000000012221, 88.59049960963380954, -45.00000000000000000 ) ) ;
#14877=LINE ( 'NONE', #10136, #3200 ) ;
#14880=CARTESIAN_POINT ( 'NONE',  ( 157.4999999999998579, 108.3995621659365867, 45.00000000000000000 ) ) ;
#14881=CARTESIAN_POINT ( 'NONE',  ( 157.4999999999998579, 133.4783122410070462, 45.00000000000000000 ) ) ;
#14884=CARTESIAN_POINT ( 'NONE',  ( 158.0000000000014211, 71.03537455708449500, -45.00000000000000000 ) ) ;
#14885=DIRECTION ( 'NONE',  ( 0.4528218681382713551, 0.8916010070293584056, -0.000000000000000000 ) ) ;
#14887=CARTESIAN_POINT ( 'NONE',  ( 158.0000000000001705, 188.9054999099155054, -45.00000000000000000 ) ) ;
#14893=DIRECTION ( 'NONE',  ( 0.4528218681383106015, 0.8916010070293384215, -0.000000000000000000 ) ) ;
#14896=ORIENTED_EDGE ( 'NONE', *, *, #16697, .F. ) ;
#14898=VERTEX_POINT ( 'NONE', #7135 ) ;
#14899=LINE ( 'NONE', #3958, #14942 ) ;
#14900=ORIENTED_EDGE ( 'NONE', *, *, #20281, .F. ) ;
#14905=DIRECTION ( 'NONE',  ( 0.8916010070296022105, 0.4528218681377911281, 0.000000000000000000 ) ) ;
#14910=VECTOR ( 'NONE', #1382, 1000.000000000000227 ) ;
#14915=EDGE_CURVE ( 'NONE', #19302, #27032, #20489, .T. ) ;
#14918=DIRECTION ( 'NONE',  ( -0.8916010070297142320, -0.4528218681375706933, 0.000000000000000000 ) ) ;
#14920=LINE ( 'NONE', #19356, #19408 ) ;
#14932=VECTOR ( 'NONE', #19148, 1000.000000000000000 ) ;
#14934=VERTEX_POINT ( 'NONE', #7423 ) ;
#14938=ADVANCED_FACE ( 'NONE', ( #14735 ), #25364, .F. ) ;
#14939=DIRECTION ( 'NONE',  ( 0.8916010070293409751, 0.4528218681383056610, 0.000000000000000000 ) ) ;
#14942=VECTOR ( 'NONE', #7998, 1000.000000000000114 ) ;
#14945=EDGE_CURVE ( 'NONE', #21625, #17150, #1783, .T. ) ;
#14946=CARTESIAN_POINT ( 'NONE',  ( 158.0000000000014211, 71.03537455708449500, -45.00000000000000000 ) ) ;
#14948=CARTESIAN_POINT ( 'NONE',  ( 157.4999999999998579, 198.6830624361901414, -45.00000000000000000 ) ) ;
#14950=EDGE_CURVE ( 'NONE', #24050, #10433, #12591, .T. ) ;
#14953=CARTESIAN_POINT ( 'NONE',  ( 157.4999999999998010, 236.3011875487955251, -45.00000000000000000 ) ) ;
#14954=LINE ( 'NONE', #8190, #19365 ) ;
#14955=ORIENTED_EDGE ( 'NONE', *, *, #8817, .F. ) ;
#14957=DIRECTION ( 'NONE',  ( 0.8916010070296226386, -0.4528218681377511046, 0.000000000000000000 ) ) ;
#14958=VERTEX_POINT ( 'NONE', #21330 ) ;
#14960=AXIS2_PLACEMENT_3D ( 'NONE', #11492, #10658, #26270 ) ;
#14962=VECTOR ( 'NONE', #23008, 1000.000000000000114 ) ;
#14965=CARTESIAN_POINT ( 'NONE',  ( 157.4999999999998579, 161.0649373235845019, 45.00000000000000000 ) ) ;
#14967=ORIENTED_EDGE ( 'NONE', *, *, #9659, .T. ) ;
#14968=VECTOR ( 'NONE', #23026, 999.9999999999998863 ) ;
#14969=ORIENTED_EDGE ( 'NONE', *, *, #14191, .F. ) ;
#14973=CARTESIAN_POINT ( 'NONE',  ( 158.0000000000011653, 93.60624962464788723, 45.00000000000000000 ) ) ;
#14974=ORIENTED_EDGE ( 'NONE', *, *, #23837, .T. ) ;
#14978=CARTESIAN_POINT ( 'NONE',  ( 157.4999999999996874, 268.9035626463865469, -45.00000000000000000 ) ) ;
#14979=DIRECTION ( 'NONE',  ( 0.8916010070295309342, -0.4528218681379315713, 0.000000000000000000 ) ) ;
#14981=CARTESIAN_POINT ( 'NONE',  ( 158.0000000000006537, 145.7637497747887210, 45.00000000000000000 ) ) ;
#14983=ORIENTED_EDGE ( 'NONE', *, *, #23454, .T. ) ;
#14985=EDGE_CURVE ( 'NONE', #14089, #3705, #1511, .T. ) ;
#14986=PLANE ( 'NONE',  #18719 ) ;
#14995=DIRECTION ( 'NONE',  ( 1.000000000000000000, 0.000000000000000000, -0.000000000000000000 ) ) ;
#14996=EDGE_LOOP ( 'NONE', ( #9876, #4244, #12976, #12603 ) ) ;
#15001=CARTESIAN_POINT ( 'NONE',  ( 158.0000000000000568, 203.4448749474510407, 45.00000000000000000 ) ) ;
#15004=VECTOR ( 'NONE', #14301, 1000.000000000000000 ) ;
#15005=ORIENTED_EDGE ( 'NONE', *, *, #6319, .T. ) ;
#15018=ORIENTED_EDGE ( 'NONE', *, *, #23113, .F. ) ;
#15021=CARTESIAN_POINT ( 'NONE',  ( 157.4999999999995453, 206.2066874587088989, 45.00000000000000000 ) ) ;
#15029=LINE ( 'NONE', #1935, #24539 ) ;
#15030=DIRECTION ( 'NONE',  ( 0.000000000000000000, -1.000000000000000000, 0.000000000000000000 ) ) ;
#15032=CARTESIAN_POINT ( 'NONE',  ( 157.4999999999998579, 158.5570623160774630, -45.00000000000000000 ) ) ;
#15035=ORIENTED_EDGE ( 'NONE', *, *, #11875, .T. ) ;
#15039=VECTOR ( 'NONE', #27459, 1000.000000000000000 ) ;
#15040=ORIENTED_EDGE ( 'NONE', *, *, #8614, .T. ) ;
#15041=VERTEX_POINT ( 'NONE', #14456 ) ;
#15045=DIRECTION ( 'NONE',  ( -0.8916010070293409751, -0.4528218681383056610, 0.000000000000000000 ) ) ;
#15049=CARTESIAN_POINT ( 'NONE',  ( 158.0000000000008527, 123.7007497147323960, 45.00000000000000000 ) ) ;
#15053=DIRECTION ( 'NONE',  ( 0.8916010070296834789, -0.4528218681376312005, 0.000000000000000000 ) ) ;
#15054=DIRECTION ( 'NONE',  ( 0.000000000000000000, -1.000000000000000000, 0.000000000000000000 ) ) ;
#15065=ORIENTED_EDGE ( 'NONE', *, *, #24211, .T. ) ;
#15067=ORIENTED_EDGE ( 'NONE', *, *, #3016, .T. ) ;
#15069=ORIENTED_EDGE ( 'NONE', *, *, #12097, .F. ) ;
#15070=EDGE_CURVE ( 'NONE', #9313, #21412, #1230, .T. ) ;
#15072=EDGE_CURVE ( 'NONE', #9774, #14497, #19317, .T. ) ;
#15073=ADVANCED_FACE ( 'NONE', ( #28062 ), #25776, .F. ) ;
#15075=EDGE_CURVE ( 'NONE', #3625, #5724, #10142, .T. ) ;
#15078=VERTEX_POINT ( 'NONE', #17870 ) ;
#15090=PLANE ( 'NONE',  #3161 ) ;
#15092=CARTESIAN_POINT ( 'NONE',  ( 157.4999999999998579, 178.6200623761337738, -45.00000000000000000 ) ) ;
#15096=AXIS2_PLACEMENT_3D ( 'NONE', #6672, #20459, #2637 ) ;
#15097=ADVANCED_FACE ( 'NONE', ( #8967 ), #28341, .F. ) ;
#15099=VECTOR ( 'NONE', #12092, 1000.000000000000227 ) ;
#15103=VERTEX_POINT ( 'NONE', #24196 ) ;
#15105=VERTEX_POINT ( 'NONE', #22182 ) ;
#15110=ORIENTED_EDGE ( 'NONE', *, *, #20387, .F. ) ;
#15112=EDGE_CURVE ( 'NONE', #24882, #15116, #6526, .T. ) ;
#15116=VERTEX_POINT ( 'NONE', #13155 ) ;
#15119=CARTESIAN_POINT ( 'NONE',  ( 157.4999999999998579, 80.81293708335913095, -45.00000000000000000 ) ) ;
#15122=PLANE ( 'NONE',  #23290 ) ;
#15123=VECTOR ( 'NONE', #27011, 1000.000000000000000 ) ;
#15124=PLANE ( 'NONE',  #23442 ) ;
#15125=EDGE_LOOP ( 'NONE', ( #27208, #25576, #1665, #12008 ) ) ;
#15128=FACE_OUTER_BOUND ( 'NONE', #8792, .T. ) ;
#15131=DIRECTION ( 'NONE',  ( -0.000000000000000000, -0.000000000000000000, -1.000000000000000000 ) ) ;
#15133=CARTESIAN_POINT ( 'NONE',  ( 157.9999999999998295, 231.0315000300280417, 45.00000000000000000 ) ) ;
#15136=ORIENTED_EDGE ( 'NONE', *, *, #7453, .T. ) ;
#15139=ORIENTED_EDGE ( 'NONE', *, *, #6623, .T. ) ;
#15140=VECTOR ( 'NONE', #18488, 1000.000000000000227 ) ;
#15144=ORIENTED_EDGE ( 'NONE', *, *, #495, .F. ) ;
#15147=EDGE_CURVE ( 'NONE', #19302, #18838, #208, .T. ) ;
#15151=ORIENTED_EDGE ( 'NONE', *, *, #26628, .F. ) ;
#15152=CARTESIAN_POINT ( 'NONE',  ( 157.4999999999994600, 213.7303124812313513, -45.00000000000000000 ) ) ;
#15153=VECTOR ( 'NONE', #22650, 1000.000000000000000 ) ;
#15157=DIRECTION ( 'NONE',  ( -0.8916010070295719014, 0.4528218681378510801, 0.000000000000000000 ) ) ;
#15159=ADVANCED_FACE ( 'NONE', ( #9110 ), #26340, .F. ) ;
#15161=VECTOR ( 'NONE', #14021, 1000.000000000000000 ) ;
#15162=LINE ( 'NONE', #13153, #3615 ) ;
#15164=ORIENTED_EDGE ( 'NONE', *, *, #9758, .F. ) ;
#15167=DIRECTION ( 'NONE',  ( -0.8916010070293383105, -0.4528218681383106015, 0.000000000000000000 ) ) ;
#15168=CARTESIAN_POINT ( 'NONE',  ( 157.9999999999999432, 211.4763749774776045, -45.00000000000000000 ) ) ;
#15170=ORIENTED_EDGE ( 'NONE', *, *, #17813, .F. ) ;
#15171=CARTESIAN_POINT ( 'NONE',  ( 158.0000000000002558, 183.3818748873943889, 45.00000000000000000 ) ) ;
#15173=PLANE ( 'NONE',  #3656 ) ;
#15174=FACE_OUTER_BOUND ( 'NONE', #3049, .T. ) ;
#15179=EDGE_LOOP ( 'NONE', ( #22272, #19906, #7555, #26531 ) ) ;
#15183=EDGE_CURVE ( 'NONE', #5204, #16487, #4488, .T. ) ;
#15185=VECTOR ( 'NONE', #1474, 1000.000000000000114 ) ;
#15187=VERTEX_POINT ( 'NONE', #8824 ) ;
#15192=LINE ( 'NONE', #2375, #26847 ) ;
#15193=CARTESIAN_POINT ( 'NONE',  ( 158.0000000000016485, 50.46449948952111697, -45.00000000000000000 ) ) ;
#15197=VECTOR ( 'NONE', #10807, 1000.000000000000000 ) ;
#15199=DIRECTION ( 'NONE',  ( -0.8916010070295314893, -0.4528218681379303501, 0.000000000000000000 ) ) ;
#15202=CARTESIAN_POINT ( 'NONE',  ( 158.0000000000009379, 118.1771246922112653, -45.00000000000000000 ) ) ;
#15204=ORIENTED_EDGE ( 'NONE', *, *, #19633, .F. ) ;
#15206=EDGE_CURVE ( 'NONE', #8537, #12718, #15583, .T. ) ;
#15209=DIRECTION ( 'NONE',  ( 0.000000000000000000, -1.000000000000000000, 0.000000000000000000 ) ) ;
#15214=ORIENTED_EDGE ( 'NONE', *, *, #26653, .F. ) ;
#15216=ORIENTED_EDGE ( 'NONE', *, *, #17205, .T. ) ;
#15218=VECTOR ( 'NONE', #12628, 1000.000000000000000 ) ;
#15220=EDGE_LOOP ( 'NONE', ( #4353, #10002, #22478, #23259 ) ) ;
#15224=VECTOR ( 'NONE', #9454, 1000.000000000000000 ) ;
#15226=CARTESIAN_POINT ( 'NONE',  ( 158.0000000000003695, 173.3503748573662051, 45.00000000000000000 ) ) ;
#15227=DIRECTION ( 'NONE',  ( -0.000000000000000000, -0.000000000000000000, -1.000000000000000000 ) ) ;
#15230=CARTESIAN_POINT ( 'NONE',  ( 158.0000000000013358, 80.55899957960563995, 45.00000000000000000 ) ) ;
#15235=VECTOR ( 'NONE', #25599, 1000.000000000000000 ) ;
#15236=CARTESIAN_POINT ( 'NONE',  ( 157.9999999999998010, 234.0472500450420341, 45.00000000000000000 ) ) ;
#15237=ADVANCED_FACE ( 'NONE', ( #15879 ), #14143, .F. ) ;
#15239=CARTESIAN_POINT ( 'NONE',  ( 157.4999999999997726, 248.8405625863305204, 45.00000000000000000 ) ) ;
#15241=VECTOR ( 'NONE', #10123, 1000.000000000000000 ) ;
#15242=VERTEX_POINT ( 'NONE', #9685 ) ;
#15244=( GEOMETRIC_REPRESENTATION_CONTEXT ( 3 ) GLOBAL_UNCERTAINTY_ASSIGNED_CONTEXT ( ( #18368 ) ) GLOBAL_UNIT_ASSIGNED_CONTEXT ( ( #8943, #4618, #6779 ) ) REPRESENTATION_CONTEXT ( 'NONE', 'WORKASPACE' ) );
#15247=DIRECTION ( 'NONE',  ( 0.000000000000000000, -1.000000000000000000, 0.000000000000000000 ) ) ;
#15250=ORIENTED_EDGE ( 'NONE', *, *, #3358, .T. ) ;
#15254=ORIENTED_EDGE ( 'NONE', *, *, #6654, .T. ) ;
#15255=VECTOR ( 'NONE', #12198, 1000.000000000000000 ) ;
#15257=VECTOR ( 'NONE', #6918, 1000.000000000000000 ) ;
#15258=CARTESIAN_POINT ( 'NONE',  ( 157.4999999999998579, 128.4625622259929401, 45.00000000000000000 ) ) ;
#15263=CARTESIAN_POINT ( 'NONE',  ( 157.9999999999998295, 231.0315000300280417, 45.00000000000000000 ) ) ;
#15268=ADVANCED_FACE ( 'NONE', ( #18444 ), #13867, .F. ) ;
#15269=DIRECTION ( 'NONE',  ( -0.000000000000000000, 0.000000000000000000, -1.000000000000000000 ) ) ;
#15270=ORIENTED_EDGE ( 'NONE', *, *, #4183, .F. ) ;
#15273=VECTOR ( 'NONE', #5148, 1000.000000000000114 ) ;
#15275=LINE ( 'NONE', #21727, #8355 ) ;
#15276=DIRECTION ( 'NONE',  ( 1.000000000000000000, 0.000000000000000000, -0.000000000000000000 ) ) ;
#15277=VERTEX_POINT ( 'NONE', #1056 ) ;
#15279=FACE_OUTER_BOUND ( 'NONE', #23160, .T. ) ;
#15280=VECTOR ( 'NONE', #17374, 1000.000000000000000 ) ;
#15281=CARTESIAN_POINT ( 'NONE',  ( 157.4999999999998579, 43.19481197075347723, 45.00000000000000000 ) ) ;
#15286=ORIENTED_EDGE ( 'NONE', *, *, #12141, .T. ) ;
#15290=ORIENTED_EDGE ( 'NONE', *, *, #26347, .F. ) ;
#15294=ORIENTED_EDGE ( 'NONE', *, *, #12296, .F. ) ;
#15301=DIRECTION ( 'NONE',  ( 0.000000000000000000, -1.000000000000000000, 0.000000000000000000 ) ) ;
#15305=CARTESIAN_POINT ( 'NONE',  ( 158.0000000000005400, 156.3031248123239436, 45.00000000000000000 ) ) ;
#15306=FACE_OUTER_BOUND ( 'NONE', #15179, .T. ) ;
#15310=DIRECTION ( 'NONE',  ( 0.4528218681382463751, 0.8916010070293711731, -0.000000000000000000 ) ) ;
#15312=DIRECTION ( 'NONE',  ( -0.8916010070293409751, -0.4528218681383056610, 0.000000000000000000 ) ) ;
#15314=FACE_OUTER_BOUND ( 'NONE', #20288, .T. ) ;
#15315=EDGE_CURVE ( 'NONE', #8063, #19692, #11989, .T. ) ;
#15319=CARTESIAN_POINT ( 'NONE',  ( 157.9999999999998579, 221.0000000000000284, 45.00000000000000000 ) ) ;
#15320=CARTESIAN_POINT ( 'NONE',  ( 157.4999999999996874, 268.9035626463865469, -45.00000000000000000 ) ) ;
#15322=VECTOR ( 'NONE', #11673, 1000.000000000000000 ) ;
#15325=ORIENTED_EDGE ( 'NONE', *, *, #15688, .T. ) ;
#15329=EDGE_CURVE ( 'NONE', #12943, #5065, #15733, .T. ) ;
#15331=DIRECTION ( 'NONE',  ( -0.000000000000000000, -0.000000000000000000, -1.000000000000000000 ) ) ;
#15335=CARTESIAN_POINT ( 'NONE',  ( 157.9999999999999716, 208.9684999699701393, -45.00000000000000000 ) ) ;
#15339=DIRECTION ( 'NONE',  ( -0.8916010070293384215, 0.4528218681383106015, 0.000000000000000000 ) ) ;
#15349=DIRECTION ( 'NONE',  ( -0.000000000000000000, 0.000000000000000000, -1.000000000000000000 ) ) ;
#15350=EDGE_CURVE ( 'NONE', #20506, #23733, #2633, .T. ) ;
#15351=EDGE_CURVE ( 'NONE', #21319, #2405, #16298, .T. ) ;
#15352=CARTESIAN_POINT ( 'NONE',  ( 163.8948362858342591, 258.6181251126050711, 1.387778780781445676E-14 ) ) ;
#15355=ORIENTED_EDGE ( 'NONE', *, *, #12335, .F. ) ;
#15361=VECTOR ( 'NONE', #12266, 999.9999999999998863 ) ;
#15367=LINE ( 'NONE', #19797, #5378 ) ;
#15369=ADVANCED_FACE ( 'NONE', ( #5924 ), #3906, .F. ) ;
#15370=CARTESIAN_POINT ( 'NONE',  ( 157.4999999999998579, 48.21056198576756202, -45.00000000000000000 ) ) ;
#15372=LINE ( 'NONE', #8750, #12596 ) ;
#15375=DIRECTION ( 'NONE',  ( 0.000000000000000000, -1.000000000000000000, 0.000000000000000000 ) ) ;
#15378=CARTESIAN_POINT ( 'NONE',  ( 157.4999999999998579, 95.86018712840139244, -45.00000000000000000 ) ) ;
#15387=VERTEX_POINT ( 'NONE', #25184 ) ;
#15388=ORIENTED_EDGE ( 'NONE', *, *, #10548, .T. ) ;
#15393=VERTEX_POINT ( 'NONE', #27606 ) ;
#15395=CARTESIAN_POINT ( 'NONE',  ( 158.0000000000011369, 96.11412463215494029, 45.00000000000000000 ) ) ;
#15396=CARTESIAN_POINT ( 'NONE',  ( 157.9999999999996874, 269.1575001501400379, 45.00000000000000000 ) ) ;
#15401=ADVANCED_FACE ( 'NONE', ( #14282 ), #1334, .F. ) ;
#15403=VERTEX_POINT ( 'NONE', #25464 ) ;
#15406=LINE ( 'NONE', #15119, #9795 ) ;
#15407=DIRECTION ( 'NONE',  ( -0.000000000000000000, 0.000000000000000000, -1.000000000000000000 ) ) ;
#15413=PLANE ( 'NONE',  #1847 ) ;
#15415=DIRECTION ( 'NONE',  ( 0.8916010070299571488, -0.4528218681370922982, 0.000000000000000000 ) ) ;
#15416=VECTOR ( 'NONE', #26197, 1000.000000000000227 ) ;
#15417=EDGE_LOOP ( 'NONE', ( #20060, #26450, #17922, #16313 ) ) ;
#15418=VECTOR ( 'NONE', #21311, 1000.000000000000000 ) ;
#15421=LINE ( 'NONE', #24173, #7464 ) ;
#15423=EDGE_LOOP ( 'NONE', ( #3555, #9625, #1351, #1437 ) ) ;
#15425=VECTOR ( 'NONE', #6732, 1000.000000000000000 ) ;
#15427=DIRECTION ( 'NONE',  ( 0.000000000000000000, -1.000000000000000000, 0.000000000000000000 ) ) ;
#15430=EDGE_CURVE ( 'NONE', #17350, #27032, #25325, .T. ) ;
#15434=DIRECTION ( 'NONE',  ( 0.8916010070296124246, 0.4528218681377710886, 0.000000000000000000 ) ) ;
#15439=DIRECTION ( 'NONE',  ( 0.8916010070297846202, -0.4528218681374320265, 0.000000000000000000 ) ) ;
#15447=VERTEX_POINT ( 'NONE', #27747 ) ;
#15452=ORIENTED_EDGE ( 'NONE', *, *, #6916, .T. ) ;
#15454=ORIENTED_EDGE ( 'NONE', *, *, #12448, .F. ) ;
#15455=LINE ( 'NONE', #15596, #10222 ) ;
#15459=CARTESIAN_POINT ( 'NONE',  ( 157.9999999999997442, 249.0945000900840398, -45.00000000000000000 ) ) ;
#15460=PLANE ( 'NONE',  #17981 ) ;
#15461=EDGE_LOOP ( 'NONE', ( #7220, #19849, #22560, #9662 ) ) ;
#15463=EDGE_CURVE ( 'NONE', #21241, #27621, #12554, .T. ) ;
#15466=ORIENTED_EDGE ( 'NONE', *, *, #3391, .F. ) ;
#15467=LINE ( 'NONE', #13172, #16348 ) ;
#15468=EDGE_CURVE ( 'NONE', #12778, #27297, #26498, .T. ) ;
#15469=ORIENTED_EDGE ( 'NONE', *, *, #18656, .F. ) ;
#15471=LINE ( 'NONE', #24218, #10833 ) ;
#15475=LINE ( 'NONE', #8574, #20075 ) ;
#15480=VECTOR ( 'NONE', #2877, 999.9999999999998863 ) ;
#15486=PLANE ( 'NONE',  #15671 ) ;
#15487=DIRECTION ( 'NONE',  ( 1.000000000000000000, 0.000000000000000000, -0.000000000000000000 ) ) ;
#15488=DIRECTION ( 'NONE',  ( -0.000000000000000000, -0.000000000000000000, -1.000000000000000000 ) ) ;
#15489=ORIENTED_EDGE ( 'NONE', *, *, #10407, .T. ) ;
#15493=FACE_OUTER_BOUND ( 'NONE', #12996, .T. ) ;
#15495=EDGE_CURVE ( 'NONE', #17587, #19047, #23451, .T. ) ;
#15498=VERTEX_POINT ( 'NONE', #1612 ) ;
#15503=EDGE_LOOP ( 'NONE', ( #22781, #25064, #20860, #24630 ) ) ;
#15504=ORIENTED_EDGE ( 'NONE', *, *, #21111, .T. ) ;
#15506=CARTESIAN_POINT ( 'NONE',  ( 158.0000000000005969, 150.7794997898028271, -45.00000000000000000 ) ) ;
#15508=EDGE_CURVE ( 'NONE', #12180, #23386, #23734, .T. ) ;
#15513=DIRECTION ( 'NONE',  ( -1.000000000000000000, 0.000000000000000000, 0.000000000000000000 ) ) ;
#15515=CARTESIAN_POINT ( 'NONE',  ( 157.9999999999996305, 284.2047501951820436, 45.00000000000000000 ) ) ;
#15517=LINE ( 'NONE', #22251, #10324 ) ;
#15523=DIRECTION ( 'NONE',  ( -0.000000000000000000, -0.000000000000000000, -1.000000000000000000 ) ) ;
#15535=CARTESIAN_POINT ( 'NONE',  ( 158.0000000000014779, 65.51174953456337846, 45.00000000000000000 ) ) ;
#15537=VECTOR ( 'NONE', #19283, 1000.000000000000000 ) ;
#15538=ORIENTED_EDGE ( 'NONE', *, *, #799, .F. ) ;
#15539=LINE ( 'NONE', #17533, #5822 ) ;
#15541=CARTESIAN_POINT ( 'NONE',  ( 157.9999999999996589, 281.1890001801680796, -45.00000000000000000 ) ) ;
#15544=DIRECTION ( 'NONE',  ( -0.000000000000000000, -0.000000000000000000, -1.000000000000000000 ) ) ;
#15548=VERTEX_POINT ( 'NONE', #4606 ) ;
#15549=PLANE ( 'NONE',  #3574 ) ;
#15553=FACE_OUTER_BOUND ( 'NONE', #2067, .T. ) ;
#15557=ADVANCED_FACE ( 'NONE', ( #2452 ), #15549, .F. ) ;
#15558=CARTESIAN_POINT ( 'NONE',  ( 157.9999999999999432, 211.4763749774776045, 45.00000000000000000 ) ) ;
#15561=EDGE_CURVE ( 'NONE', #16958, #24084, #28170, .T. ) ;
#15562=ORIENTED_EDGE ( 'NONE', *, *, #23058, .T. ) ;
#15567=VECTOR ( 'NONE', #24581, 1000.000000000000000 ) ;
#15570=VECTOR ( 'NONE', #13334, 1000.000000000000114 ) ;
#15583=LINE ( 'NONE', #6384, #10461 ) ;
#15586=LINE ( 'NONE', #21897, #10185 ) ;
#15587=DIRECTION ( 'NONE',  ( 1.000000000000000000, -1.850371707708594366E-15, 0.000000000000000000 ) ) ;
#15591=FACE_OUTER_BOUND ( 'NONE', #22196, .T. ) ;
#15592=ADVANCED_FACE ( 'NONE', ( #22000 ), #14986, .F. ) ;
#15594=ORIENTED_EDGE ( 'NONE', *, *, #4998, .T. ) ;
#15595=EDGE_CURVE ( 'NONE', #11364, #1874, #8788, .T. ) ;
#15596=CARTESIAN_POINT ( 'NONE',  ( 157.4999999999996874, 271.4114376538935289, -45.00000000000000000 ) ) ;
#15599=ORIENTED_EDGE ( 'NONE', *, *, #22025, .T. ) ;
#15601=LINE ( 'NONE', #23927, #6511 ) ;
#15602=ORIENTED_EDGE ( 'NONE', *, *, #18053, .F. ) ;
#15603=AXIS2_PLACEMENT_3D ( 'NONE', #12474, #16637, #19203 ) ;
#15605=ORIENTED_EDGE ( 'NONE', *, *, #10979, .F. ) ;
#15609=DIRECTION ( 'NONE',  ( -0.000000000000000000, 0.000000000000000000, -1.000000000000000000 ) ) ;
#15626=CARTESIAN_POINT ( 'NONE',  ( 157.4999999999996874, 271.4114376538935289, 45.00000000000000000 ) ) ;
#15630=DIRECTION ( 'NONE',  ( -0.000000000000000000, -0.000000000000000000, -1.000000000000000000 ) ) ;
#15633=EDGE_CURVE ( 'NONE', #26492, #16142, #26886, .T. ) ;
#15634=LINE ( 'NONE', #18211, #15140 ) ;
#15635=CARTESIAN_POINT ( 'NONE',  ( 157.9999999999996874, 271.1575001501400379, 45.00000000000000000 ) ) ;
#15637=VERTEX_POINT ( 'NONE', #18267 ) ;
#15642=EDGE_LOOP ( 'NONE', ( #22843, #7756, #4700, #10125 ) ) ;
#15644=ORIENTED_EDGE ( 'NONE', *, *, #28361, .F. ) ;
#15647=DIRECTION ( 'NONE',  ( 0.000000000000000000, -1.000000000000000000, 0.000000000000000000 ) ) ;
#15652=EDGE_CURVE ( 'NONE', #689, #14759, #745, .T. ) ;
#15656=LINE ( 'NONE', #26844, #22945 ) ;
#15657=ADVANCED_FACE ( 'NONE', ( #27160 ), #321, .F. ) ;
#15662=LINE ( 'NONE', #24408, #14828 ) ;
#15665=LINE ( 'NONE', #2282, #19779 ) ;
#15668=ORIENTED_EDGE ( 'NONE', *, *, #18816, .T. ) ;
#15670=EDGE_CURVE ( 'NONE', #7590, #22406, #2601, .T. ) ;
#15671=AXIS2_PLACEMENT_3D ( 'NONE', #11464, #4681, #13190 ) ;
#15672=DIRECTION ( 'NONE',  ( -1.000000000000000000, 0.000000000000000000, 0.000000000000000000 ) ) ;
#15674=EDGE_LOOP ( 'NONE', ( #13739, #15605, #8198, #2616, #5274, #11575, #6224, #25349, #19252, #9655, #9871, #9938, #27790, #6200, #7723, #27827, #24119, #25089, #25758, #24039, #1705, #24458, #10967, #21982, #16935, #697, #28385, #26971, #16591, #2163, #20677, #26533, #15705, #1557, #26610, #1282, #12923, #20531, #9800, #16245, #3312, #14955, #965, #27219, #6282, #2719, #15934, #26907, #940, #26098, #2150, #4070, #7683, #1494, #13866, #16320, #18463, #17670, #18209, #8465, #15644, #3002, #9987, #13404, #21314, #12403, #18466, #8602, #3492, #24085, #23796, #151, #1278, #7716, #16621, #19332, #20618, #19930, #9429, #5345, #4140, #24314, #1314, #7473, #28345, #12717, #9306, #21275, #28260, #27924, #16712, #17066, #28113, #18151, #15270, #14534, #23183, #9943, #14670, #23370, #1458, #6929, #18024, #8091, #12117, #13846, #11182, #21847, #23860, #21559, #16631, #9242, #18310, #16571, #2689, #26565, #19625, #4282, #2284, #16181, #14123, #21381, #22771, #11219, #5443, #12534, #405, #2252, #7753, #26346, #26171, #13686, #20221, #2222, #306, #7068, #3736, #20932, #23865, #5561, #16373, #19172, #4888, #21948, #7957, #6148, #24384, #6622, #12298, #18773, #14900, #730, #7741, #19414, #20181, #10503, #2039, #12222, #26490, #26934, #6682, #23364, #23794, #17820, #22921, #7538, #13636, #2789, #21747, #24080, #18591, #5837, #15164, #17890, #8920, #25595, #21775, #18913, #19435, #21600, #23326, #19477, #162, #28180, #22984, #15760, #13341, #11540, #798, #6901, #26081, #22491, #19591, #2926, #18114, #11876, #20187, #14470, #20398, #7364, #21875, #14460, #6506, #22980, #10615, #15794, #24680, #11552, #23440, #1104, #10600, #13002, #8598, #9703, #25858, #1584, #3587, #87, #9234, #17204, #930, #9843, #15719, #18952, #16545, #23725, #6945, #5130, #16216, #21951, #25024, #16801, #4158, #3559, #9171, #4870, #11507, #27045, #1589, #27978, #17387, #24600, #13981, #16560, #14576, #14299, #7271, #9298, #18660, #28037, #28188, #20101, #27247, #2185, #5809, #18485, #13551, #6651, #24708, #18078, #17878, #4558, #12469, #9553, #22597, #8914, #8200, #11043, #7813, #3619, #9392, #7299, #14702, #17525, #28397, #24425, #19094, #4771, #28327, #12029, #11511, #22698, #7785, #25925, #18292, #13295, #1035, #8312, #18443, #890, #21553, #18564, #12552, #14642, #7436, #17210, #3469, #19654, #15110, #17608 ) ) ;
#15675=ORIENTED_EDGE ( 'NONE', *, *, #23333, .T. ) ;
#15676=ORIENTED_EDGE ( 'NONE', *, *, #20866, .F. ) ;
#15684=LINE ( 'NONE', #9065, #25627 ) ;
#15687=CARTESIAN_POINT ( 'NONE',  ( 158.0000000000007674, 131.2243747372535267, 45.00000000000000000 ) ) ;
#15688=EDGE_CURVE ( 'NONE', #5089, #11585, #14106, .T. ) ;
#15693=VECTOR ( 'NONE', #23820, 1000.000000000000000 ) ;
#15694=EDGE_LOOP ( 'NONE', ( #11373, #9737, #374, #2034 ) ) ;
#15698=LINE ( 'NONE', #4334, #27255 ) ;
#15700=PLANE ( 'NONE',  #25636 ) ;
#15705=ORIENTED_EDGE ( 'NONE', *, *, #1003, .F. ) ;
#15708=VECTOR ( 'NONE', #5189, 1000.000000000000000 ) ;
#15713=ORIENTED_EDGE ( 'NONE', *, *, #11045, .T. ) ;
#15714=EDGE_CURVE ( 'NONE', #17167, #15103, #20415, .T. ) ;
#15715=DIRECTION ( 'NONE',  ( 0.8916010070298049373, -0.4528218681373920584, 0.000000000000000000 ) ) ;
#15718=ORIENTED_EDGE ( 'NONE', *, *, #18436, .T. ) ;
#15719=ORIENTED_EDGE ( 'NONE', *, *, #9125, .F. ) ;
#15722=EDGE_CURVE ( 'NONE', #24374, #5556, #3025, .T. ) ;
#15724=ADVANCED_FACE ( 'NONE', ( #879 ), #25014, .F. ) ;
#15725=DIRECTION ( 'NONE',  ( -0.000000000000000000, -0.000000000000000000, -1.000000000000000000 ) ) ;
#15733=LINE ( 'NONE', #24482, #18277 ) ;
#15734=DIRECTION ( 'NONE',  ( 0.4528218681383106015, -0.8916010070293384215, 0.000000000000000000 ) ) ;
#15742=FACE_OUTER_BOUND ( 'NONE', #12282, .T. ) ;
#15744=CARTESIAN_POINT ( 'NONE',  ( 157.9999999999997442, 253.6023750975910502, -45.00000000000000000 ) ) ;
#15748=ADVANCED_FACE ( 'NONE', ( #24446 ), #26737, .F. ) ;
#15749=EDGE_LOOP ( 'NONE', ( #13174, #9988, #8821, #5595 ) ) ;
#15752=PLANE ( 'NONE',  #21371 ) ;
#15753=EDGE_LOOP ( 'NONE', ( #12524, #16521, #18362, #13207 ) ) ;
#15754=AXIS2_PLACEMENT_3D ( 'NONE', #6372, #16740, #8254 ) ;
#15755=EDGE_LOOP ( 'NONE', ( #14479, #26862, #27403, #23873 ) ) ;
#15758=VECTOR ( 'NONE', #28215, 1000.000000000000000 ) ;
#15760=ORIENTED_EDGE ( 'NONE', *, *, #20404, .F. ) ;
#15762=EDGE_CURVE ( 'NONE', #18196, #2545, #22434, .T. ) ;
#15767=LINE ( 'NONE', #27088, #23406 ) ;
#15769=FACE_OUTER_BOUND ( 'NONE', #23054, .T. ) ;
#15772=DIRECTION ( 'NONE',  ( -0.8916010070297852863, -0.4528218681374307497, 0.000000000000000000 ) ) ;
#15777=VECTOR ( 'NONE', #3716, 1000.000000000000000 ) ;
#15778=DIRECTION ( 'NONE',  ( 1.000000000000000000, 0.000000000000000000, -0.000000000000000000 ) ) ;
#15781=LINE ( 'NONE', #9302, #2738 ) ;
#15787=EDGE_LOOP ( 'NONE', ( #5626, #3566, #13379, #21596 ) ) ;
#15789=ORIENTED_EDGE ( 'NONE', *, *, #2856, .F. ) ;
#15794=ORIENTED_EDGE ( 'NONE', *, *, #18796, .F. ) ;
#15796=AXIS2_PLACEMENT_3D ( 'NONE', #6095, #19454, #25911 ) ;
#15797=DIRECTION ( 'NONE',  ( -0.8916010070299679180, -0.4528218681370710375, 0.000000000000000000 ) ) ;
#15799=EDGE_CURVE ( 'NONE', #20330, #5281, #12238, .T. ) ;
#15806=CARTESIAN_POINT ( 'NONE',  ( 158.0000000000006821, 140.7479997597746433, -45.00000000000000000 ) ) ;
#15808=FACE_OUTER_BOUND ( 'NONE', #6444, .T. ) ;
#15815=DIRECTION ( 'NONE',  ( 0.000000000000000000, -1.000000000000000000, 0.000000000000000000 ) ) ;
#15823=ORIENTED_EDGE ( 'NONE', *, *, #27781, .T. ) ;
#15824=VECTOR ( 'NONE', #10751, 1000.000000000000000 ) ;
#15826=ORIENTED_EDGE ( 'NONE', *, *, #19536, .T. ) ;
#15827=EDGE_CURVE ( 'NONE', #16038, #17953, #9927, .T. ) ;
#15828=LINE ( 'NONE', #2871, #24415 ) ;
#15834=LINE ( 'NONE', #7201, #4073 ) ;
#15835=EDGE_LOOP ( 'NONE', ( #23828, #10158, #2978, #13526 ) ) ;
#15844=ORIENTED_EDGE ( 'NONE', *, *, #26911, .T. ) ;
#15847=CARTESIAN_POINT ( 'NONE',  ( 157.4999999999997158, 261.3799376238655441, -45.00000000000000000 ) ) ;
#15854=VECTOR ( 'NONE', #3086, 1000.000000000000227 ) ;
#15856=AXIS2_PLACEMENT_3D ( 'NONE', #4402, #26094, #1963 ) ;
#15860=ORIENTED_EDGE ( 'NONE', *, *, #24459, .F. ) ;
#15861=VECTOR ( 'NONE', #24455, 1000.000000000000000 ) ;
#15863=CARTESIAN_POINT ( 'NONE',  ( 158.0000000000000284, 205.9527499549551806, 45.00000000000000000 ) ) ;
#15864=LINE ( 'NONE', #7518, #27611 ) ;
#15869=EDGE_CURVE ( 'NONE', #2371, #14116, #24136, .T. ) ;
#15871=DIRECTION ( 'NONE',  ( 0.8916010070293384215, 0.4528218681383106015, 0.000000000000000000 ) ) ;
#15872=DIRECTION ( 'NONE',  ( -0.000000000000000000, 0.000000000000000000, -1.000000000000000000 ) ) ;
#15874=CARTESIAN_POINT ( 'NONE',  ( 157.4999999999995168, 208.7145624662163925, -45.00000000000000000 ) ) ;
#15877=FACE_OUTER_BOUND ( 'NONE', #6615, .T. ) ;
#15878=VERTEX_POINT ( 'NONE', #15236 ) ;
#15879=FACE_OUTER_BOUND ( 'NONE', #14257, .T. ) ;
#15884=ORIENTED_EDGE ( 'NONE', *, *, #11274, .T. ) ;
#15886=CARTESIAN_POINT ( 'NONE',  ( 158.0000000000011653, 93.60624962464788723, 45.00000000000000000 ) ) ;
#15892=ORIENTED_EDGE ( 'NONE', *, *, #28296, .F. ) ;
#15900=ADVANCED_FACE ( 'NONE', ( #17659 ), #19537, .F. ) ;
#15902=EDGE_LOOP ( 'NONE', ( #3186, #1949, #6333, #941 ) ) ;
#15903=CARTESIAN_POINT ( 'NONE',  ( 157.4999999999998579, 50.71843699327460797, 45.00000000000000000 ) ) ;
#15904=ORIENTED_EDGE ( 'NONE', *, *, #15508, .T. ) ;
#15905=EDGE_LOOP ( 'NONE', ( #10898, #3784, #3852, #11613 ) ) ;
#15906=AXIS2_PLACEMENT_3D ( 'NONE', #3479, #16707, #5496 ) ;
#15907=ORIENTED_EDGE ( 'NONE', *, *, #14741, .T. ) ;
#15910=FACE_OUTER_BOUND ( 'NONE', #21936, .T. ) ;
#15915=DIRECTION ( 'NONE',  ( -0.8916010070298056034, -0.4528218681373908372, 0.000000000000000000 ) ) ;
#15917=FACE_OUTER_BOUND ( 'NONE', #27833, .T. ) ;
#15918=CARTESIAN_POINT ( 'NONE',  ( 157.9999999999997442, 251.0945000900840398, 45.00000000000000000 ) ) ;
#15921=CARTESIAN_POINT ( 'NONE',  ( 157.9999999999998863, 218.4921249924925348, 45.00000000000000000 ) ) ;
#15922=DIRECTION ( 'NONE',  ( 0.8916010070298155954, 0.4528218681373709087, 0.000000000000000000 ) ) ;
#15923=DIRECTION ( 'NONE',  ( -0.000000000000000000, -0.000000000000000000, -1.000000000000000000 ) ) ;
#15925=VECTOR ( 'NONE', #9149, 1000.000000000000000 ) ;
#15926=ORIENTED_EDGE ( 'NONE', *, *, #2928, .T. ) ;
#15930=DIRECTION ( 'NONE',  ( 0.4528218681381900867, -0.8916010070293997058, 0.000000000000000000 ) ) ;
#15933=EDGE_LOOP ( 'NONE', ( #14967, #19697, #10111, #2869 ) ) ;
#15934=ORIENTED_EDGE ( 'NONE', *, *, #19903, .F. ) ;
#15947=LINE ( 'NONE', #13502, #15197 ) ;
#15950=LINE ( 'NONE', #2569, #10994 ) ;
#15954=VERTEX_POINT ( 'NONE', #6602 ) ;
#15955=ORIENTED_EDGE ( 'NONE', *, *, #27982, .T. ) ;
#15956=VECTOR ( 'NONE', #27284, 1000.000000000000000 ) ;
#15960=EDGE_CURVE ( 'NONE', #27632, #24388, #13505, .T. ) ;
#15961=CARTESIAN_POINT ( 'NONE',  ( 157.4999999999996874, 266.3956876388795649, 45.00000000000000000 ) ) ;
#15962=EDGE_CURVE ( 'NONE', #10433, #13314, #289, .T. ) ;
#15963=ORIENTED_EDGE ( 'NONE', *, *, #14232, .T. ) ;
#15964=ORIENTED_EDGE ( 'NONE', *, *, #18117, .F. ) ;
#15966=DIRECTION ( 'NONE',  ( -0.000000000000000000, -0.000000000000000000, -1.000000000000000000 ) ) ;
#15969=VERTEX_POINT ( 'NONE', #26699 ) ;
#15976=VECTOR ( 'NONE', #27524, 1000.000000000000000 ) ;
#15977=DIRECTION ( 'NONE',  ( 0.4528218681376912080, 0.8916010070296530587, -0.000000000000000000 ) ) ;
#15979=LINE ( 'NONE', #5460, #22255 ) ;
#15985=LINE ( 'NONE', #2744, #23907 ) ;
#15986=CARTESIAN_POINT ( 'NONE',  ( 158.0000000000001990, 186.3976249024084666, -45.00000000000000000 ) ) ;
#15997=DIRECTION ( 'NONE',  ( -0.000000000000000000, -0.000000000000000000, -1.000000000000000000 ) ) ;
#15998=DIRECTION ( 'NONE',  ( -0.000000000000000000, 0.000000000000000000, -1.000000000000000000 ) ) ;
#16001=PLANE ( 'NONE',  #10424 ) ;
#16002=DIRECTION ( 'NONE',  ( 0.8916010070297142320, 0.4528218681375707488, 0.000000000000000000 ) ) ;
#16005=FACE_OUTER_BOUND ( 'NONE', #4200, .T. ) ;
#16006=ORIENTED_EDGE ( 'NONE', *, *, #22794, .F. ) ;
#16007=PLANE ( 'NONE',  #14373 ) ;
#16010=DIRECTION ( 'NONE',  ( -0.000000000000000000, -0.000000000000000000, -1.000000000000000000 ) ) ;
#16011=LINE ( 'NONE', #5495, #17168 ) ;
#16015=CARTESIAN_POINT ( 'NONE',  ( 157.4999999999998010, 241.3169375638095460, 45.00000000000000000 ) ) ;
#16016=EDGE_CURVE ( 'NONE', #12285, #13130, #25507, .T. ) ;
#16018=DIRECTION ( 'NONE',  ( 0.000000000000000000, -1.000000000000000000, 0.000000000000000000 ) ) ;
#16021=CARTESIAN_POINT ( 'NONE',  ( 158.0000000000010232, 108.1456246621830957, -45.00000000000000000 ) ) ;
#16024=ORIENTED_EDGE ( 'NONE', *, *, #25437, .F. ) ;
#16025=AXIS2_PLACEMENT_3D ( 'NONE', #11536, #461, #18130 ) ;
#16027=CARTESIAN_POINT ( 'NONE',  ( 157.4999999999997158, 258.8720626163585621, -45.00000000000000000 ) ) ;
#16032=EDGE_CURVE ( 'NONE', #21598, #695, #10287, .T. ) ;
#16036=CARTESIAN_POINT ( 'NONE',  ( 157.9999999999996589, 276.6811251726610976, 45.00000000000000000 ) ) ;
#16038=VERTEX_POINT ( 'NONE', #28069 ) ;
#16039=CARTESIAN_POINT ( 'NONE',  ( 157.9999999999996589, 279.1890001801680796, 45.00000000000000000 ) ) ;
#16040=ORIENTED_EDGE ( 'NONE', *, *, #16628, .T. ) ;
#16041=ORIENTED_EDGE ( 'NONE', *, *, #18403, .F. ) ;
#16042=ORIENTED_EDGE ( 'NONE', *, *, #9265, .T. ) ;
#16047=CARTESIAN_POINT ( 'NONE',  ( 157.9999999999998295, 224.0157500150140208, 45.00000000000000000 ) ) ;
#16050=CARTESIAN_POINT ( 'NONE',  ( 158.0000000000015348, 58.49599951954928656, 45.00000000000000000 ) ) ;
#16057=CARTESIAN_POINT ( 'NONE',  ( 158.0000000000017053, 43.44874947450702507, 45.00000000000000000 ) ) ;
#16065=EDGE_LOOP ( 'NONE', ( #27721, #20754, #10245, #14974 ) ) ;
#16066=EDGE_CURVE ( 'NONE', #15103, #27621, #10147, .T. ) ;
#16069=DIRECTION ( 'NONE',  ( -0.000000000000000000, -0.000000000000000000, -1.000000000000000000 ) ) ;
#16076=ORIENTED_EDGE ( 'NONE', *, *, #25247, .T. ) ;
#16080=CARTESIAN_POINT ( 'NONE',  ( 157.4999999999998579, 183.6358123911478799, 45.00000000000000000 ) ) ;
#16085=EDGE_CURVE ( 'NONE', #20337, #14862, #4090, .T. ) ;
#16087=DIRECTION ( 'NONE',  ( 0.000000000000000000, -1.000000000000000000, 0.000000000000000000 ) ) ;
#16089=AXIS2_PLACEMENT_3D ( 'NONE', #9286, #3231, #13753 ) ;
#16099=ORIENTED_EDGE ( 'NONE', *, *, #885, .F. ) ;
#16100=EDGE_LOOP ( 'NONE', ( #19521, #7913, #25341, #5975 ) ) ;
#16103=ORIENTED_EDGE ( 'NONE', *, *, #27328, .F. ) ;
#16107=VECTOR ( 'NONE', #20626, 1000.000000000000114 ) ;
#16111=CARTESIAN_POINT ( 'NONE',  ( 157.4999999999998579, 183.6358123911478799, -45.00000000000000000 ) ) ;
#16112=CARTESIAN_POINT ( 'NONE',  ( 157.4999999999997726, 243.8248125713165280, 45.00000000000000000 ) ) ;
#16114=DIRECTION ( 'NONE',  ( -0.8916010070294706491, -0.4528218681380501986, 0.000000000000000000 ) ) ;
#16116=CARTESIAN_POINT ( 'NONE',  ( 157.9999999999997442, 251.0945000900840398, -45.00000000000000000 ) ) ;
#16119=LINE ( 'NONE', #14380, #25007 ) ;
#16120=CARTESIAN_POINT ( 'NONE',  ( 157.4999999999998579, 120.9389372034718093, 45.00000000000000000 ) ) ;
#16125=CARTESIAN_POINT ( 'NONE',  ( 158.0000000000006537, 145.7637497747887210, -45.00000000000000000 ) ) ;
#16128=LINE ( 'NONE', #26743, #24287 ) ;
#16132=ORIENTED_EDGE ( 'NONE', *, *, #20151, .T. ) ;
#16135=CARTESIAN_POINT ( 'NONE',  ( 158.0000000000001990, 188.3976249024084666, 45.00000000000000000 ) ) ;
#16141=DIRECTION ( 'NONE',  ( -0.000000000000000000, 0.000000000000000000, -1.000000000000000000 ) ) ;
#16142=VERTEX_POINT ( 'NONE', #16615 ) ;
#16144=ORIENTED_EDGE ( 'NONE', *, *, #15329, .F. ) ;
#16146=CARTESIAN_POINT ( 'NONE',  ( 157.4999999999998295, 226.2696875187675118, -45.00000000000000000 ) ) ;
#16147=EDGE_CURVE ( 'NONE', #12751, #26586, #23216, .T. ) ;
#16150=CARTESIAN_POINT ( 'NONE',  ( 158.0000000000001137, 195.9212499249295831, -45.00000000000000000 ) ) ;
#16154=DIRECTION ( 'NONE',  ( -0.000000000000000000, -0.000000000000000000, -1.000000000000000000 ) ) ;
#16155=DIRECTION ( 'NONE',  ( -0.000000000000000000, -0.000000000000000000, -1.000000000000000000 ) ) ;
#16156=VERTEX_POINT ( 'NONE', #68 ) ;
#16164=VECTOR ( 'NONE', #5505, 1000.000000000000000 ) ;
#16165=CARTESIAN_POINT ( 'NONE',  ( 157.4999999999998010, 236.3011875487955251, 45.00000000000000000 ) ) ;
#16168=VERTEX_POINT ( 'NONE', #21768 ) ;
#16170=DIRECTION ( 'NONE',  ( -0.000000000000000000, -0.000000000000000000, -1.000000000000000000 ) ) ;
#16172=VERTEX_POINT ( 'NONE', #6391 ) ;
#16176=CARTESIAN_POINT ( 'NONE',  ( 158.0000000000001421, 193.4133749174225443, 45.00000000000000000 ) ) ;
#16177=EDGE_LOOP ( 'NONE', ( #14834, #4247, #22055, #4943 ) ) ;
#16179=ORIENTED_EDGE ( 'NONE', *, *, #28285, .F. ) ;
#16180=DIRECTION ( 'NONE',  ( 0.000000000000000000, -1.000000000000000000, 0.000000000000000000 ) ) ;
#16181=ORIENTED_EDGE ( 'NONE', *, *, #20355, .F. ) ;
#16182=ADVANCED_FACE ( 'NONE', ( #15591 ), #2492, .F. ) ;
#16183=ORIENTED_EDGE ( 'NONE', *, *, #12318, .F. ) ;
#16184=ORIENTED_EDGE ( 'NONE', *, *, #25586, .T. ) ;
#16186=LINE ( 'NONE', #5105, #14799 ) ;
#16188=EDGE_CURVE ( 'NONE', #9224, #21137, #4371, .T. ) ;
#16189=DIRECTION ( 'NONE',  ( 0.8916010070293584056, 0.4528218681382713551, 0.000000000000000000 ) ) ;
#16190=CARTESIAN_POINT ( 'NONE',  ( 157.9999999999996589, 273.6653751576470768, 45.00000000000000000 ) ) ;
#16194=CARTESIAN_POINT ( 'NONE',  ( 158.0000000000013927, 73.54324956459154805, 45.00000000000000000 ) ) ;
#16196=ADVANCED_FACE ( 'NONE', ( #24337 ), #23922, .F. ) ;
#16198=LINE ( 'NONE', #20631, #14474 ) ;
#16202=EDGE_LOOP ( 'NONE', ( #26828, #25131, #7265, #26362 ) ) ;
#16203=FACE_OUTER_BOUND ( 'NONE', #12382, .T. ) ;
#16206=ORIENTED_EDGE ( 'NONE', *, *, #9233, .T. ) ;
#16208=VECTOR ( 'NONE', #20619, 1000.000000000000000 ) ;
#16210=PLANE ( 'NONE',  #4721 ) ;
#16213=ORIENTED_EDGE ( 'NONE', *, *, #17927, .T. ) ;
#16215=ADVANCED_FACE ( 'NONE', ( #10851 ), #2208, .F. ) ;
#16216=ORIENTED_EDGE ( 'NONE', *, *, #22717, .F. ) ;
#16217=ORIENTED_EDGE ( 'NONE', *, *, #26940, .F. ) ;
#16220=DIRECTION ( 'NONE',  ( 0.4528218681374307497, -0.8916010070297853973, 0.000000000000000000 ) ) ;
#16224=VECTOR ( 'NONE', #21321, 1000.000000000000000 ) ;
#16227=DIRECTION ( 'NONE',  ( -0.000000000000000000, -0.000000000000000000, -1.000000000000000000 ) ) ;
#16228=ADVANCED_FACE ( 'NONE', ( #15314 ), #2349, .F. ) ;
#16229=EDGE_CURVE ( 'NONE', #1981, #7228, #17588, .T. ) ;
#16236=CARTESIAN_POINT ( 'NONE',  ( 157.9999999999996874, 266.1417501351260171, 45.00000000000000000 ) ) ;
#16241=EDGE_CURVE ( 'NONE', #22232, #17818, #26627, .T. ) ;
#16242=DIRECTION ( 'NONE',  ( -0.8916010070295309342, 0.4528218681379315713, 0.000000000000000000 ) ) ;
#16243=ORIENTED_EDGE ( 'NONE', *, *, #2678, .T. ) ;
#16244=VECTOR ( 'NONE', #21994, 1000.000000000000000 ) ;
#16245=ORIENTED_EDGE ( 'NONE', *, *, #16317, .F. ) ;
#16246=EDGE_CURVE ( 'NONE', #17150, #410, #28346, .T. ) ;
#16250=VERTEX_POINT ( 'NONE', #26345 ) ;
#16252=VECTOR ( 'NONE', #13432, 1000.000000000000000 ) ;
#16258=PLANE ( 'NONE',  #19955 ) ;
#16262=DIRECTION ( 'NONE',  ( -0.8916010070295011802, -0.4528218681379903021, 0.000000000000000000 ) ) ;
#16274=VERTEX_POINT ( 'NONE', #6675 ) ;
#16277=CARTESIAN_POINT ( 'NONE',  ( 157.4999999999996874, 268.9035626463865469, 45.00000000000000000 ) ) ;
#16278=FACE_OUTER_BOUND ( 'NONE', #25907, .T. ) ;
#16280=VECTOR ( 'NONE', #5216, 1000.000000000000000 ) ;
#16287=VERTEX_POINT ( 'NONE', #27334 ) ;
#16294=DIRECTION ( 'NONE',  ( -0.8916010070293783896, 0.4528218681382319422, 0.000000000000000000 ) ) ;
#16298=LINE ( 'NONE', #25052, #9570 ) ;
#16301=CARTESIAN_POINT ( 'NONE',  ( 157.9999999999998295, 226.5236250225210313, 45.00000000000000000 ) ) ;
#16305=VERTEX_POINT ( 'NONE', #9552 ) ;
#16310=LINE ( 'NONE', #20742, #7889 ) ;
#16313=ORIENTED_EDGE ( 'NONE', *, *, #1180, .T. ) ;
#16315=EDGE_CURVE ( 'NONE', #6262, #21673, #3206, .T. ) ;
#16317=EDGE_CURVE ( 'NONE', #12148, #24050, #4935, .T. ) ;
#16320=ORIENTED_EDGE ( 'NONE', *, *, #670, .F. ) ;
#16323=VECTOR ( 'NONE', #24189, 1000.000000000000000 ) ;
#16325=VERTEX_POINT ( 'NONE', #15886 ) ;
#16328=CARTESIAN_POINT ( 'NONE',  ( 158.0000000000009663, 113.6692496847042264, 45.00000000000000000 ) ) ;
#16329=LINE ( 'NONE', #7417, #7124 ) ;
#16333=DIRECTION ( 'NONE',  ( 0.000000000000000000, -1.000000000000000000, 0.000000000000000000 ) ) ;
#16334=CARTESIAN_POINT ( 'NONE',  ( 158.0000000000000853, 198.4291249324366504, 45.00000000000000000 ) ) ;
#16340=EDGE_CURVE ( 'NONE', #23830, #5272, #2933, .T. ) ;
#16348=VECTOR ( 'NONE', #2086, 1000.000000000000000 ) ;
#16354=ORIENTED_EDGE ( 'NONE', *, *, #5060, .F. ) ;
#16355=ORIENTED_EDGE ( 'NONE', *, *, #3116, .T. ) ;
#16356=ORIENTED_EDGE ( 'NONE', *, *, #14742, .T. ) ;
#16361=DIRECTION ( 'NONE',  ( 0.4528218681378515797, 0.8916010070295715684, -0.000000000000000000 ) ) ;
#16365=CARTESIAN_POINT ( 'NONE',  ( 158.0000000000008811, 121.1928747072253572, -45.00000000000000000 ) ) ;
#16366=CARTESIAN_POINT ( 'NONE',  ( 158.0000000000010232, 106.1456246621830957, 45.00000000000000000 ) ) ;
#16369=VECTOR ( 'NONE', #4365, 1000.000000000000114 ) ;
#16372=LINE ( 'NONE', #27538, #24438 ) ;
#16373=ORIENTED_EDGE ( 'NONE', *, *, #7934, .F. ) ;
#16377=FACE_OUTER_BOUND ( 'NONE', #2610, .T. ) ;
#16378=EDGE_LOOP ( 'NONE', ( #24998, #2747, #22670, #9254 ) ) ;
#16380=LINE ( 'NONE', #16655, #24893 ) ;
#16382=VERTEX_POINT ( 'NONE', #18025 ) ;
#16383=VECTOR ( 'NONE', #22643, 1000.000000000000227 ) ;
#16384=ORIENTED_EDGE ( 'NONE', *, *, #24281, .T. ) ;
#16387=VERTEX_POINT ( 'NONE', #9829 ) ;
#16388=EDGE_LOOP ( 'NONE', ( #22281, #11597, #23151, #4664 ) ) ;
#16389=DIRECTION ( 'NONE',  ( -0.8916010070299471568, 0.4528218681371123377, 0.000000000000000000 ) ) ;
#16393=EDGE_CURVE ( 'NONE', #1795, #26789, #11719, .T. ) ;
#16397=PLANE ( 'NONE',  #2631 ) ;
#16398=VECTOR ( 'NONE', #20544, 1000.000000000000114 ) ;
#16402=LINE ( 'NONE', #5611, #22988 ) ;
#16404=CARTESIAN_POINT ( 'NONE',  ( 157.4999999999998579, 158.5570623160774630, 45.00000000000000000 ) ) ;
#16405=ORIENTED_EDGE ( 'NONE', *, *, #15206, .F. ) ;
#16408=FACE_OUTER_BOUND ( 'NONE', #13375, .T. ) ;
#16419=DIRECTION ( 'NONE',  ( -0.000000000000000000, -0.000000000000000000, -1.000000000000000000 ) ) ;
#16425=LINE ( 'NONE', #906, #18039 ) ;
#16426=CARTESIAN_POINT ( 'NONE',  ( 158.0000000000000284, 203.9527499549551806, 45.00000000000000000 ) ) ;
#16427=CARTESIAN_POINT ( 'NONE',  ( 157.9999999999998010, 231.5393750375350237, 45.00000000000000000 ) ) ;
#16430=ADVANCED_FACE ( 'NONE', ( #8374 ), #12418, .F. ) ;
#16431=EDGE_CURVE ( 'NONE', #6317, #12327, #27891, .T. ) ;
#16432=CARTESIAN_POINT ( 'NONE',  ( 157.9999999999996305, 286.7126252026890256, -45.00000000000000000 ) ) ;
#16433=PLANE ( 'NONE',  #5127 ) ;
#16439=DIRECTION ( 'NONE',  ( 0.000000000000000000, -1.000000000000000000, 0.000000000000000000 ) ) ;
#16443=DIRECTION ( 'NONE',  ( -0.8916010070298868717, -0.4528218681372309651, 0.000000000000000000 ) ) ;
#16445=DIRECTION ( 'NONE',  ( -0.8916010070295616874, -0.4528218681378710642, 0.000000000000000000 ) ) ;
#16446=VERTEX_POINT ( 'NONE', #27753 ) ;
#16450=LINE ( 'NONE', #27073, #17516 ) ;
#16452=EDGE_LOOP ( 'NONE', ( #11325, #4796, #20247, #12502 ) ) ;
#16454=CARTESIAN_POINT ( 'NONE',  ( 158.0000000000012221, 90.59049960963380954, 45.00000000000000000 ) ) ;
#16455=ORIENTED_EDGE ( 'NONE', *, *, #14985, .F. ) ;
#16457=AXIS2_PLACEMENT_3D ( 'NONE', #20871, #9251, #25179 ) ;
#16458=VERTEX_POINT ( 'NONE', #19144 ) ;
#16460=FACE_OUTER_BOUND ( 'NONE', #18008, .T. ) ;
#16466=DIRECTION ( 'NONE',  ( 0.000000000000000000, 0.000000000000000000, 1.000000000000000000 ) ) ;
#16467=CARTESIAN_POINT ( 'NONE',  ( 157.4999999999996874, 266.3956876388795649, 45.00000000000000000 ) ) ;
#16473=DIRECTION ( 'NONE',  ( 1.000000000000000000, 0.000000000000000000, -0.000000000000000000 ) ) ;
#16480=CARTESIAN_POINT ( 'NONE',  ( 158.0000000000010232, 108.1456246621830957, -45.00000000000000000 ) ) ;
#16483=FACE_OUTER_BOUND ( 'NONE', #16100, .T. ) ;
#16487=VERTEX_POINT ( 'NONE', #17135 ) ;
#16495=EDGE_CURVE ( 'NONE', #15548, #13125, #16578, .T. ) ;
#16500=EDGE_CURVE ( 'NONE', #24747, #16964, #5792, .T. ) ;
#16501=DIRECTION ( 'NONE',  ( -0.000000000000000000, -0.000000000000000000, -1.000000000000000000 ) ) ;
#16503=FACE_OUTER_BOUND ( 'NONE', #5939, .T. ) ;
#16512=CARTESIAN_POINT ( 'NONE',  ( 158.0000000000013074, 83.06687458711267880, -45.00000000000000000 ) ) ;
#16513=LINE ( 'NONE', #21476, #11621 ) ;
#16516=AXIS2_PLACEMENT_3D ( 'NONE', #6851, #27099, #9728 ) ;
#16521=ORIENTED_EDGE ( 'NONE', *, *, #21821, .F. ) ;
#16523=EDGE_CURVE ( 'NONE', #18620, #2585, #21014, .T. ) ;
#16527=EDGE_CURVE ( 'NONE', #17634, #16387, #18725, .T. ) ;
#16530=CARTESIAN_POINT ( 'NONE',  ( 158.0000000000006537, 143.7637497747887210, -45.00000000000000000 ) ) ;
#16532=CARTESIAN_POINT ( 'NONE',  ( 158.0000000000006537, 141.2558747672816821, 45.00000000000000000 ) ) ;
#16534=DIRECTION ( 'NONE',  ( -0.8916010070296632728, -0.4528218681376712240, 0.000000000000000000 ) ) ;
#16535=CARTESIAN_POINT ( 'NONE',  ( 157.9999999999998579, 219.0000000000000284, 45.00000000000000000 ) ) ;
#16537=EDGE_CURVE ( 'NONE', #9050, #7851, #14564, .T. ) ;
#16543=VECTOR ( 'NONE', #7132, 1000.000000000000000 ) ;
#16545=ORIENTED_EDGE ( 'NONE', *, *, #24211, .F. ) ;
#16550=FACE_OUTER_BOUND ( 'NONE', #6053, .T. ) ;
#16553=ORIENTED_EDGE ( 'NONE', *, *, #14624, .T. ) ;
#16554=CARTESIAN_POINT ( 'NONE',  ( 158.0000000000006253, 148.2716247822957882, -45.00000000000000000 ) ) ;
#16556=DIRECTION ( 'NONE',  ( 0.4528218681372709331, -0.8916010070298664436, 0.000000000000000000 ) ) ;
#16560=ORIENTED_EDGE ( 'NONE', *, *, #9659, .F. ) ;
#16562=AXIS2_PLACEMENT_3D ( 'NONE', #21573, #15269, #7027 ) ;
#16566=CARTESIAN_POINT ( 'NONE',  ( 157.4999999999997726, 243.8248125713165280, 45.00000000000000000 ) ) ;
#16569=VECTOR ( 'NONE', #20416, 1000.000000000000000 ) ;
#16570=CARTESIAN_POINT ( 'NONE',  ( 158.0000000000017053, 45.44874947450702507, 45.00000000000000000 ) ) ;
#16571=ORIENTED_EDGE ( 'NONE', *, *, #23856, .F. ) ;
#16572=EDGE_CURVE ( 'NONE', #12431, #19970, #1894, .T. ) ;
#16574=CARTESIAN_POINT ( 'NONE',  ( 158.0000000000012506, 86.08262460212675649, 45.00000000000000000 ) ) ;
#16575=CARTESIAN_POINT ( 'NONE',  ( 158.0000000000012221, 90.59049960963380954, -45.00000000000000000 ) ) ;
#16576=CARTESIAN_POINT ( 'NONE',  ( 157.9999999999999432, 211.4763749774776045, -45.00000000000000000 ) ) ;
#16578=LINE ( 'NONE', #3913, #7321 ) ;
#16579=EDGE_LOOP ( 'NONE', ( #14511, #23353, #15823, #6862, #648, #14644, #25803, #25243, #6154, #14539, #18149, #15388, #6656, #22767, #27439, #4911, #12595, #9090, #19818, #26363, #12850, #11556, #5585, #18356, #17809, #26762, #3465, #15452, #21661, #4913, #8060, #49, #14540, #20067, #23312, #11040, #16657, #18727, #24506, #8215, #11975, #27543, #357, #12811, #25547, #27112, #25722, #934, #23341, #652, #6258, #13670, #8024, #8139, #8394, #22605, #4, #27379, #27382, #7413, #6211, #25329, #252, #24165, #14432, #5191, #17250, #15216, #14023, #10940, #9060, #18363, #16700, #5020, #16040, #11436, #85, #13027, #15286, #24676, #5899, #10934, #4754, #7672, #25619, #4556, #24725, #4987, #9394, #13665, #24025, #3788, #23363, #666, #1836, #23595, #28160, #24075, #21778, #33, #22202, #28081, #4640, #3570, #17701, #24988, #8033, #20640, #16213, #806, #21410, #3286, #10992, #25265, #18250, #26629, #13637, #9528, #20849, #19161, #18147, #22093, #12152, #1322, #28162, #26600, #13927, #8487, #10617, #12570, #27135, #4421, #23286, #19396, #5414, #10790, #12463, #5265, #9585, #17644, #12216, #27168, #10616, #19859, #5135, #11400, #2259, #2186, #5341, #20102, #3712, #21566, #8136, #15668, #20425, #13139, #14445, #20070, #15005, #28041, #110, #1857, #19449, #5966, #14789, #25408, #22977, #25018, #21283, #11737, #27647, #13276, #26179, #25072, #15718, #28068, #15904, #14197, #12919, #10442, #1562, #27869, #18249, #26396, #2350, #20025, #21060, #23173, #24342, #17243, #16899, #10251, #6578, #13956, #11988, #14466, #12072, #3181, #16042, #22897, #22207, #5386, #13629, #13923, #22412, #12574, #13777, #22194, #26559, #3320, #14785, #23474, #15926, #14782, #21382, #25101, #6476, #265, #10022, #27864, #14129, #6063, #21914, #15675, #25684, #23295, #27061, #5369, #2729, #5765, #15250, #2474, #8461, #19907, #27409, #26138, #5634, #27865, #18395, #6500, #22129, #17459, #17775, #10560, #15136, #5244, #5935, #15040, #6826, #20744, #1022, #3998, #14093, #14983, #3650, #2650, #17696, #18359, #23546, #23871, #24576, #229, #14633, #2300, #8569, #15067, #19750, #22642, #2215, #19709, #16132, #19259, #233, #12608, #11802, #27774, #21353, #4214, #20950, #19057, #22234, #10221, #5175, #15844, #12501, #4380, #26045, #12917, #1893, #8938, #10409, #19149, #11867, #8955, #7856, #6802, #24210, #28203, #24712, #25117 ) ) ;
#16584=LINE ( 'NONE', #7818, #18876 ) ;
#16585=CARTESIAN_POINT ( 'NONE',  ( 158.0000000000007958, 130.7164997297464595, 45.00000000000000000 ) ) ;
#16587=EDGE_CURVE ( 'NONE', #12172, #15969, #179, .T. ) ;
#16589=CARTESIAN_POINT ( 'NONE',  ( 157.4999999999997442, 251.3484375938375024, 45.00000000000000000 ) ) ;
#16590=DIRECTION ( 'NONE',  ( 0.000000000000000000, -1.000000000000000000, 0.000000000000000000 ) ) ;
#16591=ORIENTED_EDGE ( 'NONE', *, *, #16495, .F. ) ;
#16592=EDGE_CURVE ( 'NONE', #11585, #23433, #11244, .T. ) ;
#16597=ADVANCED_FACE ( 'NONE', ( #15279 ), #15700, .F. ) ;
#16604=LINE ( 'NONE', #23485, #10814 ) ;
#16605=CARTESIAN_POINT ( 'NONE',  ( 157.4999999999997726, 246.3326875788235384, 45.00000000000000000 ) ) ;
#16614=EDGE_LOOP ( 'NONE', ( #28298, #18113, #25791, #10919 ) ) ;
#16615=CARTESIAN_POINT ( 'NONE',  ( 157.4999999999998579, 201.1909374436971802, 45.00000000000000000 ) ) ;
#16618=LINE ( 'NONE', #27793, #27713 ) ;
#16621=ORIENTED_EDGE ( 'NONE', *, *, #16758, .F. ) ;
#16625=ORIENTED_EDGE ( 'NONE', *, *, #816, .T. ) ;
#16627=ORIENTED_EDGE ( 'NONE', *, *, #22981, .F. ) ;
#16628=EDGE_CURVE ( 'NONE', #12668, #5675, #10672, .T. ) ;
#16631=ORIENTED_EDGE ( 'NONE', *, *, #17505, .F. ) ;
#16637=DIRECTION ( 'NONE',  ( 1.000000000000000000, 0.000000000000000000, -0.000000000000000000 ) ) ;
#16642=FACE_OUTER_BOUND ( 'NONE', #16614, .T. ) ;
#16644=DIRECTION ( 'NONE',  ( 0.4528218681382319422, -0.8916010070293783896, 0.000000000000000000 ) ) ;
#16648=VECTOR ( 'NONE', #22696, 999.9999999999998863 ) ;
#16653=ORIENTED_EDGE ( 'NONE', *, *, #19514, .T. ) ;
#16655=CARTESIAN_POINT ( 'NONE',  ( 158.0000000000014495, 68.01962454207041731, -45.00000000000000000 ) ) ;
#16656=ORIENTED_EDGE ( 'NONE', *, *, #17829, .T. ) ;
#16657=ORIENTED_EDGE ( 'NONE', *, *, #14017, .T. ) ;
#16658=EDGE_CURVE ( 'NONE', #2371, #20337, #8521, .T. ) ;
#16659=EDGE_LOOP ( 'NONE', ( #14672, #10681, #26870, #10896 ) ) ;
#16660=EDGE_CURVE ( 'NONE', #4740, #7009, #6772, .T. ) ;
#16668=DIRECTION ( 'NONE',  ( 0.8916010070293584056, -0.4528218681382712996, 0.000000000000000000 ) ) ;
#16678=LINE ( 'NONE', #25432, #19835 ) ;
#16682=EDGE_CURVE ( 'NONE', #7082, #20397, #3167, .T. ) ;
#16683=AXIS2_PLACEMENT_3D ( 'NONE', #18567, #22455, #16002 ) ;
#16690=EDGE_LOOP ( 'NONE', ( #13999, #17038, #351, #12292 ) ) ;
#16695=ORIENTED_EDGE ( 'NONE', *, *, #18313, .T. ) ;
#16696=DIRECTION ( 'NONE',  ( 0.8916010070293384215, 0.4528218681383106015, 0.000000000000000000 ) ) ;
#16697=EDGE_CURVE ( 'NONE', #27297, #12778, #14675, .T. ) ;
#16698=LINE ( 'NONE', #1598, #8818 ) ;
#16700=ORIENTED_EDGE ( 'NONE', *, *, #4895, .T. ) ;
#16705=CARTESIAN_POINT ( 'NONE',  ( 158.0000000000012506, 86.08262460212675649, 45.00000000000000000 ) ) ;
#16707=DIRECTION ( 'NONE',  ( 0.4528218681383056610, -0.8916010070293409751, 0.000000000000000000 ) ) ;
#16708=VECTOR ( 'NONE', #12416, 999.9999999999998863 ) ;
#16712=ORIENTED_EDGE ( 'NONE', *, *, #19956, .F. ) ;
#16715=LINE ( 'NONE', #27888, #4672 ) ;
#16721=LINE ( 'NONE', #6215, #10696 ) ;
#16724=ORIENTED_EDGE ( 'NONE', *, *, #26195, .F. ) ;
#16728=VECTOR ( 'NONE', #13534, 1000.000000000000000 ) ;
#16729=LINE ( 'NONE', #1353, #15241 ) ;
#16731=ORIENTED_EDGE ( 'NONE', *, *, #19956, .T. ) ;
#16733=VERTEX_POINT ( 'NONE', #3031 ) ;
#16736=ADVANCED_FACE ( 'NONE', ( #20698 ), #22298, .F. ) ;
#16738=ORIENTED_EDGE ( 'NONE', *, *, #7431, .F. ) ;
#16740=DIRECTION ( 'NONE',  ( 0.4528218681382912836, -0.8916010070293483025, 0.000000000000000000 ) ) ;
#16743=VECTOR ( 'NONE', #20236, 1000.000000000000114 ) ;
#16746=CARTESIAN_POINT ( 'NONE',  ( 157.4999999999996589, 278.9350626764145318, -45.00000000000000000 ) ) ;
#16752=LINE ( 'NONE', #1232, #23336 ) ;
#16756=DIRECTION ( 'NONE',  ( 0.4528218681371111165, -0.8916010070299477119, 0.000000000000000000 ) ) ;
#16757=LINE ( 'NONE', #25509, #222 ) ;
#16758=EDGE_CURVE ( 'NONE', #18364, #9383, #9518, .T. ) ;
#16766=VECTOR ( 'NONE', #14728, 1000.000000000000000 ) ;
#16770=VERTEX_POINT ( 'NONE', #2607 ) ;
#16771=VECTOR ( 'NONE', #15247, 1000.000000000000000 ) ;
#16773=DIRECTION ( 'NONE',  ( -0.8916010070293584056, 0.4528218681382713551, 0.000000000000000000 ) ) ;
#16777=CARTESIAN_POINT ( 'NONE',  ( 157.9999999999996305, 288.7126252026890256, 45.00000000000000000 ) ) ;
#16780=CARTESIAN_POINT ( 'NONE',  ( 167.4999999999996589, 258.6181251126050711, 1.387778780781445676E-14 ) ) ;
#16781=VECTOR ( 'NONE', #11840, 1000.000000000000000 ) ;
#16784=DIRECTION ( 'NONE',  ( 1.000000000000000000, 0.000000000000000000, -0.000000000000000000 ) ) ;
#16787=ORIENTED_EDGE ( 'NONE', *, *, #20582, .F. ) ;
#16793=ORIENTED_EDGE ( 'NONE', *, *, #12017, .F. ) ;
#16795=DIRECTION ( 'NONE',  ( 0.4528218681379315713, 0.8916010070295309342, -0.000000000000000000 ) ) ;
#16796=VERTEX_POINT ( 'NONE', #18553 ) ;
#16797=ORIENTED_EDGE ( 'NONE', *, *, #21438, .T. ) ;
#16798=ORIENTED_EDGE ( 'NONE', *, *, #16975, .F. ) ;
#16801=ORIENTED_EDGE ( 'NONE', *, *, #18992, .F. ) ;
#16803=CARTESIAN_POINT ( 'NONE',  ( 158.0000000000011937, 93.09837461714084839, 45.00000000000000000 ) ) ;
#16805=CARTESIAN_POINT ( 'NONE',  ( 157.9999999999998295, 229.0315000300280417, 45.00000000000000000 ) ) ;
#16806=VECTOR ( 'NONE', #27504, 1000.000000000000000 ) ;
#16809=DIRECTION ( 'NONE',  ( -0.000000000000000000, -0.000000000000000000, -1.000000000000000000 ) ) ;
#16810=EDGE_CURVE ( 'NONE', #2468, #22232, #16128, .T. ) ;
#16811=CARTESIAN_POINT ( 'NONE',  ( 157.4999999999996874, 266.3956876388795649, 45.00000000000000000 ) ) ;
#16817=PLANE ( 'NONE',  #18761 ) ;
#16821=VECTOR ( 'NONE', #18739, 1000.000000000000000 ) ;
#16827=ORIENTED_EDGE ( 'NONE', *, *, #6489, .F. ) ;
#16832=CARTESIAN_POINT ( 'NONE',  ( 158.0000000000001990, 188.3976249024084666, 45.00000000000000000 ) ) ;
#16833=FACE_OUTER_BOUND ( 'NONE', #25207, .T. ) ;
#16834=CARTESIAN_POINT ( 'NONE',  ( 158.0000000000009663, 113.6692496847042264, 45.00000000000000000 ) ) ;
#16835=ORIENTED_EDGE ( 'NONE', *, *, #13101, .T. ) ;
#16836=CARTESIAN_POINT ( 'NONE',  ( 157.9999999999996874, 271.1575001501400379, 45.00000000000000000 ) ) ;
#16842=CARTESIAN_POINT ( 'NONE',  ( 157.9999999999998010, 236.0472500450420341, -45.00000000000000000 ) ) ;
#16845=CARTESIAN_POINT ( 'NONE',  ( 158.0000000000013074, 83.06687458711267880, 45.00000000000000000 ) ) ;
#16846=DIRECTION ( 'NONE',  ( 1.000000000000000000, 0.000000000000000000, -0.000000000000000000 ) ) ;
#16851=LINE ( 'NONE', #12135, #27987 ) ;
#16852=CARTESIAN_POINT ( 'NONE',  ( 157.4999999999998579, 188.6515624061619576, 45.00000000000000000 ) ) ;
#16854=VERTEX_POINT ( 'NONE', #14665 ) ;
#16858=CARTESIAN_POINT ( 'NONE',  ( 157.4999999999998579, 58.24206201579573872, 45.00000000000000000 ) ) ;
#16865=VECTOR ( 'NONE', #10476, 1000.000000000000000 ) ;
#16866=CARTESIAN_POINT ( 'NONE',  ( 157.4999999999997726, 243.8248125713165280, -45.00000000000000000 ) ) ;
#16871=ORIENTED_EDGE ( 'NONE', *, *, #514, .F. ) ;
#16872=ORIENTED_EDGE ( 'NONE', *, *, #24622, .T. ) ;
#16883=CARTESIAN_POINT ( 'NONE',  ( 157.4999999999998579, 223.7618125112605298, 45.00000000000000000 ) ) ;
#16885=CARTESIAN_POINT ( 'NONE',  ( 157.9999999999997158, 259.1260001201120531, 45.00000000000000000 ) ) ;
#16891=DIRECTION ( 'NONE',  ( 0.8916010070298049373, -0.4528218681373920584, 0.000000000000000000 ) ) ;
#16892=CARTESIAN_POINT ( 'NONE',  ( 158.0000000000012790, 83.57474959461971764, 45.00000000000000000 ) ) ;
#16895=CARTESIAN_POINT ( 'NONE',  ( 158.0000000000004547, 165.8267498348450886, 45.00000000000000000 ) ) ;
#16897=DIRECTION ( 'NONE',  ( 0.8916010070293483025, 0.4528218681382912836, 0.000000000000000000 ) ) ;
#16898=VECTOR ( 'NONE', #12272, 1000.000000000000000 ) ;
#16899=ORIENTED_EDGE ( 'NONE', *, *, #2219, .T. ) ;
#16902=VERTEX_POINT ( 'NONE', #27433 ) ;
#16903=DIRECTION ( 'NONE',  ( -0.000000000000000000, -0.000000000000000000, -1.000000000000000000 ) ) ;
#16904=EDGE_CURVE ( 'NONE', #15116, #1795, #25293, .T. ) ;
#16905=ORIENTED_EDGE ( 'NONE', *, *, #20673, .F. ) ;
#16907=LINE ( 'NONE', #27807, #5825 ) ;
#16921=LINE ( 'NONE', #14775, #13011 ) ;
#16922=ORIENTED_EDGE ( 'NONE', *, *, #26840, .F. ) ;
#16923=EDGE_CURVE ( 'NONE', #20027, #4329, #18971, .T. ) ;
#16927=CARTESIAN_POINT ( 'NONE',  ( 158.0000000000002842, 178.8739998798873216, 45.00000000000000000 ) ) ;
#16932=ORIENTED_EDGE ( 'NONE', *, *, #10979, .T. ) ;
#16935=ORIENTED_EDGE ( 'NONE', *, *, #18925, .F. ) ;
#16936=ORIENTED_EDGE ( 'NONE', *, *, #10331, .F. ) ;
#16940=CARTESIAN_POINT ( 'NONE',  ( 158.0000000000015916, 53.48024950453520177, 45.00000000000000000 ) ) ;
#16943=FACE_OUTER_BOUND ( 'NONE', #23332, .T. ) ;
#16948=VECTOR ( 'NONE', #14616, 999.9999999999998863 ) ;
#16955=EDGE_CURVE ( 'NONE', #25616, #19117, #13954, .T. ) ;
#16956=CARTESIAN_POINT ( 'NONE',  ( 157.4999999999998579, 138.4940622560211239, 45.00000000000000000 ) ) ;
#16957=DIRECTION ( 'NONE',  ( -0.000000000000000000, -0.000000000000000000, -1.000000000000000000 ) ) ;
#16958=VERTEX_POINT ( 'NONE', #11359 ) ;
#16964=VERTEX_POINT ( 'NONE', #17805 ) ;
#16967=CARTESIAN_POINT ( 'NONE',  ( 158.0000000000001137, 195.9212499249295831, 45.00000000000000000 ) ) ;
#16970=ADVANCED_FACE ( 'NONE', ( #24564 ), #22264, .F. ) ;
#16971=CARTESIAN_POINT ( 'NONE',  ( 157.9999999999996589, 279.1890001801680796, 45.00000000000000000 ) ) ;
#16972=EDGE_CURVE ( 'NONE', #5280, #5095, #4872, .T. ) ;
#16975=EDGE_CURVE ( 'NONE', #24347, #18723, #17954, .T. ) ;
#16984=ORIENTED_EDGE ( 'NONE', *, *, #54, .F. ) ;
#16988=CARTESIAN_POINT ( 'NONE',  ( 157.4999999999995737, 203.6988124512014338, 45.00000000000000000 ) ) ;
#16991=DIRECTION ( 'NONE',  ( -0.000000000000000000, -0.000000000000000000, -1.000000000000000000 ) ) ;
#16993=LINE ( 'NONE', #17137, #28126 ) ;
#16997=CARTESIAN_POINT ( 'NONE',  ( 158.0000000000001705, 188.9054999099155054, 45.00000000000000000 ) ) ;
#17000=CARTESIAN_POINT ( 'NONE',  ( 157.4999999999998579, 183.6358123911478799, 45.00000000000000000 ) ) ;
#17001=ORIENTED_EDGE ( 'NONE', *, *, #3413, .F. ) ;
#17006=VECTOR ( 'NONE', #5576, 1000.000000000000000 ) ;
#17007=ADVANCED_FACE ( 'NONE', ( #9343 ), #9627, .F. ) ;
#17008=VERTEX_POINT ( 'NONE', #20248 ) ;
#17011=VECTOR ( 'NONE', #19426, 1000.000000000000000 ) ;
#17013=PLANE ( 'NONE',  #15796 ) ;
#17019=DIRECTION ( 'NONE',  ( 0.000000000000000000, -1.000000000000000000, 0.000000000000000000 ) ) ;
#17021=CARTESIAN_POINT ( 'NONE',  ( 157.4999999999998579, 110.9074371734436255, 45.00000000000000000 ) ) ;
#17022=CARTESIAN_POINT ( 'NONE',  ( 157.4999999999998579, 45.70268697826052318, 45.00000000000000000 ) ) ;
#17025=DIRECTION ( 'NONE',  ( -0.000000000000000000, -0.000000000000000000, -1.000000000000000000 ) ) ;
#17027=LINE ( 'NONE', #20815, #27636 ) ;
#17032=ORIENTED_EDGE ( 'NONE', *, *, #26982, .T. ) ;
#17035=CARTESIAN_POINT ( 'NONE',  ( 157.9999999999996305, 286.2047501951820436, 45.00000000000000000 ) ) ;
#17037=FACE_OUTER_BOUND ( 'NONE', #11832, .T. ) ;
#17038=ORIENTED_EDGE ( 'NONE', *, *, #21618, .F. ) ;
#17043=ORIENTED_EDGE ( 'NONE', *, *, #21926, .F. ) ;
#17044=PLANE ( 'NONE',  #6745 ) ;
#17046=DIRECTION ( 'NONE',  ( -0.000000000000000000, -0.000000000000000000, -1.000000000000000000 ) ) ;
#17048=VECTOR ( 'NONE', #6245, 1000.000000000000000 ) ;
#17053=DIRECTION ( 'NONE',  ( -0.000000000000000000, -0.000000000000000000, -1.000000000000000000 ) ) ;
#17059=CARTESIAN_POINT ( 'NONE',  ( 158.0000000000012790, 85.57474959461971764, -45.00000000000000000 ) ) ;
#17061=EDGE_CURVE ( 'NONE', #12718, #9667, #17753, .T. ) ;
#17063=LINE ( 'NONE', #107, #15824 ) ;
#17064=CARTESIAN_POINT ( 'NONE',  ( 157.4999999999998579, 168.5885623461056184, 45.00000000000000000 ) ) ;
#17065=ORIENTED_EDGE ( 'NONE', *, *, #4352, .F. ) ;
#17066=ORIENTED_EDGE ( 'NONE', *, *, #17238, .F. ) ;
#17073=VERTEX_POINT ( 'NONE', #24225 ) ;
#17074=VECTOR ( 'NONE', #23223, 1000.000000000000000 ) ;
#17076=ORIENTED_EDGE ( 'NONE', *, *, #15799, .F. ) ;
#17077=EDGE_LOOP ( 'NONE', ( #17550, #15069, #2451, #22812 ) ) ;
#17080=ADVANCED_FACE ( 'NONE', ( #26369 ), #4397, .F. ) ;
#17085=AXIS2_PLACEMENT_3D ( 'NONE', #24739, #5330, #26739 ) ;
#17086=LINE ( 'NONE', #17227, #18586 ) ;
#17088=DIRECTION ( 'NONE',  ( -0.8916010070293485246, -0.4528218681382906730, 0.000000000000000000 ) ) ;
#17090=EDGE_CURVE ( 'NONE', #5655, #8321, #26505, .T. ) ;
#17095=DIRECTION ( 'NONE',  ( 0.000000000000000000, -1.000000000000000000, 0.000000000000000000 ) ) ;
#17106=VECTOR ( 'NONE', #5638, 1000.000000000000000 ) ;
#17108=AXIS2_PLACEMENT_3D ( 'NONE', #22973, #25927, #26067 ) ;
#17110=CARTESIAN_POINT ( 'NONE',  ( 157.9999999999997158, 256.6181251126050711, 45.00000000000000000 ) ) ;
#17115=VECTOR ( 'NONE', #26966, 1000.000000000000000 ) ;
#17122=DIRECTION ( 'NONE',  ( 1.000000000000000000, 0.000000000000000000, -0.000000000000000000 ) ) ;
#17123=DIRECTION ( 'NONE',  ( 0.000000000000000000, -1.000000000000000000, 0.000000000000000000 ) ) ;
#17124=VECTOR ( 'NONE', #25138, 1000.000000000000000 ) ;
#17128=DIRECTION ( 'NONE',  ( 0.8916010070296327417, -0.4528218681377311761, 0.000000000000000000 ) ) ;
#17131=VECTOR ( 'NONE', #8590, 1000.000000000000114 ) ;
#17132=ADVANCED_FACE ( 'NONE', ( #10874 ), #26087, .F. ) ;
#17135=CARTESIAN_POINT ( 'NONE',  ( 187.4999999999996305, 258.6181251126050711, 6.000000000000019540 ) ) ;
#17137=CARTESIAN_POINT ( 'NONE',  ( 158.0000000000013642, 76.05112457209858690, 45.00000000000000000 ) ) ;
#17141=LINE ( 'NONE', #21165, #28093 ) ;
#17145=VERTEX_POINT ( 'NONE', #13182 ) ;
#17149=ORIENTED_EDGE ( 'NONE', *, *, #14492, .F. ) ;
#17150=VERTEX_POINT ( 'NONE', #17903 ) ;
#17151=VERTEX_POINT ( 'NONE', #15193 ) ;
#17153=LINE ( 'NONE', #15152, #4711 ) ;
#17154=EDGE_CURVE ( 'NONE', #855, #19117, #9144, .T. ) ;
#17156=CARTESIAN_POINT ( 'NONE',  ( 187.4999999999996305, 288.9665627064425166, 45.00000000000000000 ) ) ;
#17157=CARTESIAN_POINT ( 'NONE',  ( 158.0000000000005116, 160.8109998198309825, 45.00000000000000000 ) ) ;
#17167=VERTEX_POINT ( 'NONE', #2516 ) ;
#17168=VECTOR ( 'NONE', #3478, 1000.000000000000000 ) ;
#17169=ADVANCED_FACE ( 'NONE', ( #11309 ), #23805, .F. ) ;
#17170=CARTESIAN_POINT ( 'NONE',  ( 157.4999999999998579, 171.0964373536126573, 45.00000000000000000 ) ) ;
#17184=VERTEX_POINT ( 'NONE', #20341 ) ;
#17187=ORIENTED_EDGE ( 'NONE', *, *, #19088, .T. ) ;
#17188=DIRECTION ( 'NONE',  ( 0.000000000000000000, -1.000000000000000000, 0.000000000000000000 ) ) ;
#17189=VECTOR ( 'NONE', #13501, 999.9999999999998863 ) ;
#17191=LINE ( 'NONE', #26085, #127 ) ;
#17195=CARTESIAN_POINT ( 'NONE',  ( 158.0000000000007674, 131.2243747372535267, -45.00000000000000000 ) ) ;
#17204=ORIENTED_EDGE ( 'NONE', *, *, #19199, .F. ) ;
#17205=EDGE_CURVE ( 'NONE', #15878, #23120, #25080, .T. ) ;
#17210=ORIENTED_EDGE ( 'NONE', *, *, #7519, .F. ) ;
#17221=DIRECTION ( 'NONE',  ( -0.000000000000000000, -0.000000000000000000, -1.000000000000000000 ) ) ;
#17222=CARTESIAN_POINT ( 'NONE',  ( 157.4999999999998579, 223.7618125112605298, -45.00000000000000000 ) ) ;
#17223=VECTOR ( 'NONE', #20487, 1000.000000000000000 ) ;
#17225=LINE ( 'NONE', #6450, #2776 ) ;
#17226=ADVANCED_FACE ( 'NONE', ( #18475 ), #26650, .F. ) ;
#17227=CARTESIAN_POINT ( 'NONE',  ( 158.0000000000007958, 128.7164997297464595, 45.00000000000000000 ) ) ;
#17238=EDGE_CURVE ( 'NONE', #26259, #14934, #15767, .T. ) ;
#17243=ORIENTED_EDGE ( 'NONE', *, *, #15722, .T. ) ;
#17244=AXIS2_PLACEMENT_3D ( 'NONE', #22488, #369, #2653 ) ;
#17246=DIRECTION ( 'NONE',  ( 0.8916010070293783896, 0.4528218681382319422, 0.000000000000000000 ) ) ;
#17247=DIRECTION ( 'NONE',  ( 1.000000000000000000, 0.000000000000000000, -0.000000000000000000 ) ) ;
#17249=VECTOR ( 'NONE', #3411, 1000.000000000000000 ) ;
#17250=ORIENTED_EDGE ( 'NONE', *, *, #24154, .T. ) ;
#17251=EDGE_CURVE ( 'NONE', #4042, #13806, #22504, .T. ) ;
#17253=EDGE_CURVE ( 'NONE', #12700, #19742, #18338, .T. ) ;
#17254=DIRECTION ( 'NONE',  ( 0.8916010070295005141, -0.4528218681379915789, 0.000000000000000000 ) ) ;
#17255=DIRECTION ( 'NONE',  ( 0.000000000000000000, -1.000000000000000000, 0.000000000000000000 ) ) ;
#17265=CARTESIAN_POINT ( 'NONE',  ( 157.4999999999998579, 113.4153121809506786, -45.00000000000000000 ) ) ;
#17267=CARTESIAN_POINT ( 'NONE',  ( 157.4999999999996305, 286.4586876989355915, -45.00000000000000000 ) ) ;
#17269=CARTESIAN_POINT ( 'NONE',  ( 157.4999999999998579, 115.9231871884577174, 45.00000000000000000 ) ) ;
#17272=ADVANCED_FACE ( 'NONE', ( #15910 ), #7130, .F. ) ;
#17280=DIRECTION ( 'NONE',  ( -0.000000000000000000, -0.000000000000000000, -1.000000000000000000 ) ) ;
#17285=CARTESIAN_POINT ( 'NONE',  ( 157.4999999999998579, 115.9231871884577174, -45.00000000000000000 ) ) ;
#17289=EDGE_CURVE ( 'NONE', #17818, #27311, #7275, .T. ) ;
#17293=DIRECTION ( 'NONE',  ( 0.000000000000000000, -1.000000000000000000, 0.000000000000000000 ) ) ;
#17294=CARTESIAN_POINT ( 'NONE',  ( 157.4999999999998579, 161.0649373235845019, 45.00000000000000000 ) ) ;
#17295=DIRECTION ( 'NONE',  ( 0.000000000000000000, -1.000000000000000000, 0.000000000000000000 ) ) ;
#17296=DIRECTION ( 'NONE',  ( -0.8916010070298868717, -0.4528218681372309651, 0.000000000000000000 ) ) ;
#17301=CARTESIAN_POINT ( 'NONE',  ( 157.9999999999997726, 248.5866250825770294, 45.00000000000000000 ) ) ;
#17303=VECTOR ( 'NONE', #15715, 1000.000000000000000 ) ;
#17304=VERTEX_POINT ( 'NONE', #22788 ) ;
#17306=VECTOR ( 'NONE', #27113, 1000.000000000000000 ) ;
#17307=PLANE ( 'NONE',  #17108 ) ;
#17309=DIRECTION ( 'NONE',  ( 0.8916010070297751833, 0.4528218681374507892, 0.000000000000000000 ) ) ;
#17311=DIRECTION ( 'NONE',  ( -0.8916010070298766577, -0.4528218681372509491, 0.000000000000000000 ) ) ;
#17313=CARTESIAN_POINT ( 'NONE',  ( 158.0000000000001421, 193.4133749174225443, 45.00000000000000000 ) ) ;
#17314=VERTEX_POINT ( 'NONE', #9713 ) ;
#17319=AXIS2_PLACEMENT_3D ( 'NONE', #16845, #27600, #4039 ) ;
#17321=EDGE_CURVE ( 'NONE', #9638, #26421, #14877, .T. ) ;
#17324=VECTOR ( 'NONE', #19235, 1000.000000000000114 ) ;
#17328=EDGE_CURVE ( 'NONE', #5281, #800, #1505, .T. ) ;
#17331=DIRECTION ( 'NONE',  ( 0.4528218681382907285, -0.8916010070293486356, 0.000000000000000000 ) ) ;
#17334=FACE_OUTER_BOUND ( 'NONE', #25273, .T. ) ;
#17336=CARTESIAN_POINT ( 'NONE',  ( 157.4999999999998010, 241.3169375638095460, 45.00000000000000000 ) ) ;
#17339=EDGE_LOOP ( 'NONE', ( #11008, #16827, #10318, #18412 ) ) ;
#17340=LINE ( 'NONE', #13472, #10583 ) ;
#17350=VERTEX_POINT ( 'NONE', #20905 ) ;
#17353=STYLED_ITEM('',(#28427),#28013);
#17357=DIRECTION ( 'NONE',  ( 1.000000000000000000, 0.000000000000000000, -0.000000000000000000 ) ) ;
#17361=VECTOR ( 'NONE', #16087, 1000.000000000000000 ) ;
#17363=CARTESIAN_POINT ( 'NONE',  ( 157.4999999999998579, 58.24206201579573872, -45.00000000000000000 ) ) ;
#17368=CARTESIAN_POINT ( 'NONE',  ( 157.9999999999996589, 281.1890001801680796, 45.00000000000000000 ) ) ;
#17374=DIRECTION ( 'NONE',  ( 0.000000000000000000, -1.000000000000000000, 0.000000000000000000 ) ) ;
#17380=AXIS2_PLACEMENT_3D ( 'NONE', #10343, #10484, #19103 ) ;
#17382=ORIENTED_EDGE ( 'NONE', *, *, #15147, .F. ) ;
#17386=AXIS2_PLACEMENT_3D ( 'NONE', #5633, #23300, #27314 ) ;
#17387=ORIENTED_EDGE ( 'NONE', *, *, #22638, .F. ) ;
#17391=ORIENTED_EDGE ( 'NONE', *, *, #24179, .T. ) ;
#17393=VECTOR ( 'NONE', #2459, 1000.000000000000000 ) ;
#17395=CARTESIAN_POINT ( 'NONE',  ( 158.0000000000010232, 108.1456246621830957, 45.00000000000000000 ) ) ;
#17396=VECTOR ( 'NONE', #11557, 1000.000000000000000 ) ;
#17400=FACE_OUTER_BOUND ( 'NONE', #8306, .T. ) ;
#17402=EDGE_CURVE ( 'NONE', #20915, #16382, #27779, .T. ) ;
#17406=CARTESIAN_POINT ( 'NONE',  ( 158.0000000000009948, 110.6534996696901345, 45.00000000000000000 ) ) ;
#17409=CARTESIAN_POINT ( 'NONE',  ( 158.0000000000010516, 103.6377496546760568, -45.00000000000000000 ) ) ;
#17412=VERTEX_POINT ( 'NONE', #14588 ) ;
#17414=DIRECTION ( 'NONE',  ( 0.4528218681369524101, 0.8916010070300282031, -0.000000000000000000 ) ) ;
#17416=LINE ( 'NONE', #13401, #19871 ) ;
#17424=VERTEX_POINT ( 'NONE', #5535 ) ;
#17427=CARTESIAN_POINT ( 'NONE',  ( 158.0000000000011937, 93.09837461714084839, -45.00000000000000000 ) ) ;
#17429=VERTEX_POINT ( 'NONE', #5955 ) ;
#17431=EDGE_CURVE ( 'NONE', #19692, #27184, #21040, .T. ) ;
#17435=DIRECTION ( 'NONE',  ( -0.000000000000000000, -0.000000000000000000, -1.000000000000000000 ) ) ;
#17436=DIRECTION ( 'NONE',  ( -0.000000000000000000, -0.000000000000000000, -1.000000000000000000 ) ) ;
#17438=CIRCLE ( 'NONE', #2755, 6.000000000000005329 ) ;
#17440=EDGE_LOOP ( 'NONE', ( #13159, #20856, #14142, #3102 ) ) ;
#17441=DIRECTION ( 'NONE',  ( 1.000000000000000000, 0.000000000000000000, -0.000000000000000000 ) ) ;
#17443=CARTESIAN_POINT ( 'NONE',  ( 158.0000000000005400, 155.7952498048169048, 45.00000000000000000 ) ) ;
#17444=DIRECTION ( 'NONE',  ( -0.8916010070297142320, -0.4528218681375706933, 0.000000000000000000 ) ) ;
#17448=CARTESIAN_POINT ( 'NONE',  ( 158.0000000000009663, 113.6692496847042264, -45.00000000000000000 ) ) ;
#17454=ADVANCED_FACE ( 'NONE', ( #19168 ), #1776, .F. ) ;
#17455=VECTOR ( 'NONE', #12164, 1000.000000000000227 ) ;
#17456=FACE_OUTER_BOUND ( 'NONE', #14758, .T. ) ;
#17458=PLANE ( 'NONE',  #23201 ) ;
#17459=ORIENTED_EDGE ( 'NONE', *, *, #9909, .T. ) ;
#17460=EDGE_CURVE ( 'NONE', #14958, #2723, #6275, .T. ) ;
#17461=VERTEX_POINT ( 'NONE', #15049 ) ;
#17462=DIRECTION ( 'NONE',  ( -0.000000000000000000, -0.000000000000000000, -1.000000000000000000 ) ) ;
#17466=CARTESIAN_POINT ( 'NONE',  ( 157.9999999999999147, 215.9842499849850697, 45.00000000000000000 ) ) ;
#17470=CARTESIAN_POINT ( 'NONE',  ( 157.4999999999998579, 90.84443711338730054, 45.00000000000000000 ) ) ;
#17472=DIRECTION ( 'NONE',  ( -0.8916010070296429557, 0.4528218681377111920, 0.000000000000000000 ) ) ;
#17474=VECTOR ( 'NONE', #8224, 999.9999999999998863 ) ;
#17475=CARTESIAN_POINT ( 'NONE',  ( 158.0000000000008811, 123.1928747072253572, 45.00000000000000000 ) ) ;
#17476=LINE ( 'NONE', #8722, #9433 ) ;
#17480=ORIENTED_EDGE ( 'NONE', *, *, #4780, .T. ) ;
#17481=CARTESIAN_POINT ( 'NONE',  ( 158.0000000000013927, 75.54324956459154805, -45.00000000000000000 ) ) ;
#17484=CARTESIAN_POINT ( 'NONE',  ( 158.0000000000010232, 108.1456246621830957, 45.00000000000000000 ) ) ;
#17487=EDGE_CURVE ( 'NONE', #14163, #27184, #14486, .T. ) ;
#17489=VERTEX_POINT ( 'NONE', #12622 ) ;
#17496=AXIS2_PLACEMENT_3D ( 'NONE', #26635, #24921, #18319 ) ;
#17497=CARTESIAN_POINT ( 'NONE',  ( 158.0000000000000000, 208.4606249624626457, 45.00000000000000000 ) ) ;
#17499=EDGE_CURVE ( 'NONE', #16958, #21312, #8150, .T. ) ;
#17500=DIRECTION ( 'NONE',  ( 1.000000000000000000, 0.000000000000000000, -0.000000000000000000 ) ) ;
#17503=CARTESIAN_POINT ( 'NONE',  ( 187.4999999999996305, 40.68693696324645970, 45.00000000000000000 ) ) ;
#17505=EDGE_CURVE ( 'NONE', #13208, #19162, #1398, .T. ) ;
#17507=DIRECTION ( 'NONE',  ( 0.000000000000000000, -1.000000000000000000, 0.000000000000000000 ) ) ;
#17508=LINE ( 'NONE', #26276, #10460 ) ;
#17509=DIRECTION ( 'NONE',  ( -0.000000000000000000, 0.000000000000000000, -1.000000000000000000 ) ) ;
#17513=DIRECTION ( 'NONE',  ( 0.4528218681373720744, 0.8916010070298151513, -0.000000000000000000 ) ) ;
#17515=LINE ( 'NONE', #24139, #26271 ) ;
#17516=VECTOR ( 'NONE', #7406, 1000.000000000000000 ) ;
#17518=EDGE_LOOP ( 'NONE', ( #22411, #18804, #28255, #27043 ) ) ;
#17525=ORIENTED_EDGE ( 'NONE', *, *, #10004, .F. ) ;
#17526=ORIENTED_EDGE ( 'NONE', *, *, #10935, .F. ) ;
#17529=LINE ( 'NONE', #15396, #27349 ) ;
#17530=ORIENTED_EDGE ( 'NONE', *, *, #12258, .F. ) ;
#17533=CARTESIAN_POINT ( 'NONE',  ( 157.4999999999998579, 55.73418700828869277, -45.00000000000000000 ) ) ;
#17540=VECTOR ( 'NONE', #3280, 1000.000000000000000 ) ;
#17541=CARTESIAN_POINT ( 'NONE',  ( 157.9999999999996874, 264.1417501351260171, 45.00000000000000000 ) ) ;
#17547=CARTESIAN_POINT ( 'NONE',  ( 157.9999999999996874, 266.1417501351260171, 45.00000000000000000 ) ) ;
#17550=ORIENTED_EDGE ( 'NONE', *, *, #6181, .T. ) ;
#17556=LINE ( 'NONE', #24599, #28206 ) ;
#17560=ORIENTED_EDGE ( 'NONE', *, *, #27083, .F. ) ;
#17561=VECTOR ( 'NONE', #7296, 1000.000000000000000 ) ;
#17568=CARTESIAN_POINT ( 'NONE',  ( 157.9999999999999716, 208.9684999699701393, -45.00000000000000000 ) ) ;
#17571=VECTOR ( 'NONE', #1043, 999.9999999999998863 ) ;
#17574=CARTESIAN_POINT ( 'NONE',  ( 157.9999999999997442, 253.6023750975910502, 45.00000000000000000 ) ) ;
#17575=DIRECTION ( 'NONE',  ( -0.8916010070295511403, 0.4528218681378916033, 0.000000000000000000 ) ) ;
#17580=CARTESIAN_POINT ( 'NONE',  ( 157.4999999999998579, 113.4153121809506786, 45.00000000000000000 ) ) ;
#17584=CARTESIAN_POINT ( 'NONE',  ( 157.4999999999997442, 256.3641876088515232, 45.00000000000000000 ) ) ;
#17585=PLANE ( 'NONE',  #21053 ) ;
#17587=VERTEX_POINT ( 'NONE', #19634 ) ;
#17588=LINE ( 'NONE', #358, #10510 ) ;
#17594=CARTESIAN_POINT ( 'NONE',  ( 157.9999999999997158, 261.6338751276190351, 45.00000000000000000 ) ) ;
#17597=EDGE_CURVE ( 'NONE', #4287, #24562, #21794, .T. ) ;
#17602=CARTESIAN_POINT ( 'NONE',  ( 157.9999999999997726, 241.5708750675630370, 45.00000000000000000 ) ) ;
#17604=AXIS2_PLACEMENT_3D ( 'NONE', #25055, #18722, #22896 ) ;
#17605=EDGE_LOOP ( 'NONE', ( #28018, #3276, #19862, #28191 ) ) ;
#17608=ORIENTED_EDGE ( 'NONE', *, *, #3921, .F. ) ;
#17614=LINE ( 'NONE', #26649, #24083 ) ;
#17616=VECTOR ( 'NONE', #13419, 1000.000000000000000 ) ;
#17618=CARTESIAN_POINT ( 'NONE',  ( 157.9999999999996589, 273.6653751576470768, 45.00000000000000000 ) ) ;
#17619=DIRECTION ( 'NONE',  ( 0.8916010070293384215, 0.4528218681383106015, 0.000000000000000000 ) ) ;
#17620=PRODUCT_DEFINITION_SHAPE ( 'NONE', 'NONE',  #8432 ) ;
#17621=DIRECTION ( 'NONE',  ( 1.000000000000000000, -0.000000000000000000, -0.000000000000000000 ) ) ;
#17624=ADVANCED_FACE ( 'NONE', ( #11020 ), #24226, .F. ) ;
#17625=VECTOR ( 'NONE', #28173, 1000.000000000000000 ) ;
#17626=LINE ( 'NONE', #24520, #5566 ) ;
#17627=LINE ( 'NONE', #23673, #1744 ) ;
#17634=VERTEX_POINT ( 'NONE', #9289 ) ;
#17636=CARTESIAN_POINT ( 'NONE',  ( 158.0000000000001990, 186.3976249024084666, -45.00000000000000000 ) ) ;
#17637=EDGE_LOOP ( 'NONE', ( #19482, #13598, #6580, #11838 ) ) ;
#17638=FACE_OUTER_BOUND ( 'NONE', #6809, .T. ) ;
#17639=VERTEX_POINT ( 'NONE', #26371 ) ;
#17641=ORIENTED_EDGE ( 'NONE', *, *, #16758, .T. ) ;
#17642=ORIENTED_EDGE ( 'NONE', *, *, #15960, .F. ) ;
#17644=ORIENTED_EDGE ( 'NONE', *, *, #602, .T. ) ;
#17648=EDGE_CURVE ( 'NONE', #3887, #9114, #96, .T. ) ;
#17650=EDGE_CURVE ( 'NONE', #17988, #22350, #8858, .T. ) ;
#17654=CARTESIAN_POINT ( 'NONE',  ( 158.0000000000013927, 75.54324956459154805, 45.00000000000000000 ) ) ;
#17655=DIRECTION ( 'NONE',  ( -0.8916010070293384215, 0.4528218681383106015, 0.000000000000000000 ) ) ;
#17657=LINE ( 'NONE', #1850, #4022 ) ;
#17659=FACE_OUTER_BOUND ( 'NONE', #6821, .T. ) ;
#17661=CARTESIAN_POINT ( 'NONE',  ( 158.0000000000013927, 75.54324956459154805, 45.00000000000000000 ) ) ;
#17662=DIRECTION ( 'NONE',  ( 0.8916010070298056034, 0.4528218681373908372, 0.000000000000000000 ) ) ;
#17668=ORIENTED_EDGE ( 'NONE', *, *, #25864, .T. ) ;
#17669=ORIENTED_EDGE ( 'NONE', *, *, #2047, .F. ) ;
#17670=ORIENTED_EDGE ( 'NONE', *, *, #27551, .F. ) ;
#17672=LINE ( 'NONE', #6324, #24889 ) ;
#17677=VECTOR ( 'NONE', #15915, 1000.000000000000000 ) ;
#17679=CARTESIAN_POINT ( 'NONE',  ( 157.4999999999998579, 85.82868709837320864, -45.00000000000000000 ) ) ;
#17681=EDGE_CURVE ( 'NONE', #1943, #5089, #23951, .T. ) ;
#17686=ADVANCED_FACE ( 'NONE', ( #17904 ), #2099, .F. ) ;
#17687=EDGE_CURVE ( 'NONE', #5281, #28009, #22505, .T. ) ;
#17690=VERTEX_POINT ( 'NONE', #2810 ) ;
#17692=VECTOR ( 'NONE', #16227, 1000.000000000000000 ) ;
#17694=CARTESIAN_POINT ( 'NONE',  ( 158.0000000000000853, 200.9369999399436892, -45.00000000000000000 ) ) ;
#17696=ORIENTED_EDGE ( 'NONE', *, *, #20800, .T. ) ;
#17698=CARTESIAN_POINT ( 'NONE',  ( 157.4999999999998295, 228.7775625262745223, 45.00000000000000000 ) ) ;
#17701=ORIENTED_EDGE ( 'NONE', *, *, #7953, .T. ) ;
#17706=ORIENTED_EDGE ( 'NONE', *, *, #16527, .T. ) ;
#17707=ORIENTED_EDGE ( 'NONE', *, *, #5523, .F. ) ;
#17709=EDGE_CURVE ( 'NONE', #1480, #26626, #7701, .T. ) ;
#17710=EDGE_CURVE ( 'NONE', #4413, #11964, #3232, .T. ) ;
#17711=DIRECTION ( 'NONE',  ( -0.000000000000000000, -0.000000000000000000, -1.000000000000000000 ) ) ;
#17713=ORIENTED_EDGE ( 'NONE', *, *, #18656, .T. ) ;
#17714=VECTOR ( 'NONE', #15331, 1000.000000000000000 ) ;
#17715=CARTESIAN_POINT ( 'NONE',  ( 157.4999999999998579, 168.5885623461056184, -45.00000000000000000 ) ) ;
#17718=CARTESIAN_POINT ( 'NONE',  ( 157.9999999999997726, 241.5708750675630370, -45.00000000000000000 ) ) ;
#17719=CARTESIAN_POINT ( 'NONE',  ( 158.0000000000013358, 78.55899957960562574, 45.00000000000000000 ) ) ;
#17721=VECTOR ( 'NONE', #17019, 1000.000000000000000 ) ;
#17722=DIRECTION ( 'NONE',  ( 0.8916010070297846202, -0.4528218681374320265, 0.000000000000000000 ) ) ;
#17726=CARTESIAN_POINT ( 'NONE',  ( 187.4999999999996305, 258.6181251126050711, 1.387778780781445676E-14 ) ) ;
#17728=FACE_OUTER_BOUND ( 'NONE', #7110, .T. ) ;
#17730=ORIENTED_EDGE ( 'NONE', *, *, #14945, .T. ) ;
#17733=CARTESIAN_POINT ( 'NONE',  ( 158.0000000000003411, 175.8582498648732440, 45.00000000000000000 ) ) ;
#17736=ORIENTED_EDGE ( 'NONE', *, *, #21182, .F. ) ;
#17738=ORIENTED_EDGE ( 'NONE', *, *, #16431, .T. ) ;
#17739=VECTOR ( 'NONE', #4625, 1000.000000000000114 ) ;
#17740=LINE ( 'NONE', #24212, #4256 ) ;
#17741=ORIENTED_EDGE ( 'NONE', *, *, #4838, .T. ) ;
#17743=ORIENTED_EDGE ( 'NONE', *, *, #11957, .F. ) ;
#17752=DIRECTION ( 'NONE',  ( -0.8916010070297338830, 0.4528218681375318910, 0.000000000000000000 ) ) ;
#17753=LINE ( 'NONE', #4674, #2253 ) ;
#17759=EDGE_CURVE ( 'NONE', #27097, #19656, #13903, .T. ) ;
#17760=LINE ( 'NONE', #6422, #24133 ) ;
#17762=LINE ( 'NONE', #8863, #10614 ) ;
#17765=ORIENTED_EDGE ( 'NONE', *, *, #26523, .F. ) ;
#17766=DIRECTION ( 'NONE',  ( 1.000000000000000000, 0.000000000000000000, -0.000000000000000000 ) ) ;
#17770=VERTEX_POINT ( 'NONE', #24658 ) ;
#17771=EDGE_CURVE ( 'NONE', #15393, #12920, #2957, .T. ) ;
#17772=PLANE ( 'NONE',  #6098 ) ;
#17775=ORIENTED_EDGE ( 'NONE', *, *, #8287, .T. ) ;
#17777=ORIENTED_EDGE ( 'NONE', *, *, #10517, .T. ) ;
#17778=EDGE_CURVE ( 'NONE', #2965, #21780, #5536, .T. ) ;
#17780=VERTEX_POINT ( 'NONE', #27089 ) ;
#17781=ORIENTED_EDGE ( 'NONE', *, *, #10956, .F. ) ;
#17782=DIRECTION ( 'NONE',  ( 0.8916010070295614653, -0.4528218681378716193, 0.000000000000000000 ) ) ;
#17785=DIRECTION ( 'NONE',  ( -0.8916010070296022105, 0.4528218681377911281, 0.000000000000000000 ) ) ;
#17787=EDGE_CURVE ( 'NONE', #14580, #13671, #7419, .T. ) ;
#17791=PLANE ( 'NONE',  #10356 ) ;
#17801=LINE ( 'NONE', #21693, #12509 ) ;
#17804=EDGE_CURVE ( 'NONE', #14369, #15187, #9714, .T. ) ;
#17805=CARTESIAN_POINT ( 'NONE',  ( 157.4999999999996305, 286.4586876989355915, -45.00000000000000000 ) ) ;
#17806=VECTOR ( 'NONE', #11477, 1000.000000000000000 ) ;
#17807=DIRECTION ( 'NONE',  ( 0.000000000000000000, -1.000000000000000000, 0.000000000000000000 ) ) ;
#17809=ORIENTED_EDGE ( 'NONE', *, *, #21387, .T. ) ;
#17810=ORIENTED_EDGE ( 'NONE', *, *, #14673, .F. ) ;
#17812=VERTEX_POINT ( 'NONE', #27499 ) ;
#17813=EDGE_CURVE ( 'NONE', #1568, #7082, #12725, .T. ) ;
#17816=LINE ( 'NONE', #22416, #24147 ) ;
#17817=VECTOR ( 'NONE', #17722, 1000.000000000000114 ) ;
#17818=VERTEX_POINT ( 'NONE', #12305 ) ;
#17820=ORIENTED_EDGE ( 'NONE', *, *, #3997, .F. ) ;
#17822=CARTESIAN_POINT ( 'NONE',  ( 157.4999999999998579, 80.81293708335913095, 45.00000000000000000 ) ) ;
#17825=LINE ( 'NONE', #20266, #12372 ) ;
#17826=DIRECTION ( 'NONE',  ( 0.000000000000000000, -1.000000000000000000, 0.000000000000000000 ) ) ;
#17827=VECTOR ( 'NONE', #23497, 1000.000000000000000 ) ;
#17828=CARTESIAN_POINT ( 'NONE',  ( 158.0000000000007958, 130.7164997297464595, -45.00000000000000000 ) ) ;
#17829=EDGE_CURVE ( 'NONE', #9601, #6438, #19033, .T. ) ;
#17840=VECTOR ( 'NONE', #27042, 1000.000000000000000 ) ;
#17841=DIRECTION ( 'NONE',  ( 0.000000000000000000, -1.000000000000000000, 0.000000000000000000 ) ) ;
#17843=ORIENTED_EDGE ( 'NONE', *, *, #6434, .F. ) ;
#17849=FACE_OUTER_BOUND ( 'NONE', #22276, .T. ) ;
#17853=DIRECTION ( 'NONE',  ( -0.000000000000000000, -0.000000000000000000, -1.000000000000000000 ) ) ;
#17859=VECTOR ( 'NONE', #25982, 1000.000000000000227 ) ;
#17862=FACE_OUTER_BOUND ( 'NONE', #18194, .T. ) ;
#17864=CARTESIAN_POINT ( 'NONE',  ( 157.4999999999998579, 110.9074371734436255, -45.00000000000000000 ) ) ;
#17869=EDGE_CURVE ( 'NONE', #21761, #1908, #19314, .T. ) ;
#17870=CARTESIAN_POINT ( 'NONE',  ( 157.4999999999998579, 163.5728123310915407, -45.00000000000000000 ) ) ;
#17874=LINE ( 'NONE', #9113, #16252 ) ;
#17875=ORIENTED_EDGE ( 'NONE', *, *, #24214, .F. ) ;
#17876=DIRECTION ( 'NONE',  ( 0.000000000000000000, -1.000000000000000000, 0.000000000000000000 ) ) ;
#17878=ORIENTED_EDGE ( 'NONE', *, *, #19865, .F. ) ;
#17879=LINE ( 'NONE', #22334, #23063 ) ;
#17883=PLANE ( 'NONE',  #17496 ) ;
#17888=EDGE_CURVE ( 'NONE', #3327, #12285, #25361, .T. ) ;
#17890=ORIENTED_EDGE ( 'NONE', *, *, #25355, .F. ) ;
#17892=DIRECTION ( 'NONE',  ( -0.000000000000000000, -0.000000000000000000, -1.000000000000000000 ) ) ;
#17895=DIRECTION ( 'NONE',  ( 1.000000000000000000, 0.000000000000000000, -0.000000000000000000 ) ) ;
#17896=ORIENTED_EDGE ( 'NONE', *, *, #7075, .F. ) ;
#17899=ORIENTED_EDGE ( 'NONE', *, *, #20281, .T. ) ;
#17903=CARTESIAN_POINT ( 'NONE',  ( 158.0000000000007105, 136.2401247522676044, -45.00000000000000000 ) ) ;
#17904=FACE_OUTER_BOUND ( 'NONE', #22086, .T. ) ;
#17909=FACE_OUTER_BOUND ( 'NONE', #11089, .T. ) ;
#17912=ORIENTED_EDGE ( 'NONE', *, *, #3642, .F. ) ;
#17916=CARTESIAN_POINT ( 'NONE',  ( 158.0000000000005969, 150.7794997898028271, 45.00000000000000000 ) ) ;
#17922=ORIENTED_EDGE ( 'NONE', *, *, #10548, .F. ) ;
#17923=EDGE_CURVE ( 'NONE', #24347, #372, #23208, .T. ) ;
#17925=ORIENTED_EDGE ( 'NONE', *, *, #54, .T. ) ;
#17926=ORIENTED_EDGE ( 'NONE', *, *, #15714, .F. ) ;
#17927=EDGE_CURVE ( 'NONE', #19893, #2965, #25916, .T. ) ;
#17929=ORIENTED_EDGE ( 'NONE', *, *, #3209, .T. ) ;
#17932=CARTESIAN_POINT ( 'NONE',  ( 158.0000000000007674, 131.2243747372535267, 45.00000000000000000 ) ) ;
#17940=CARTESIAN_POINT ( 'NONE',  ( 157.9999999999996305, 288.7126252026890256, -45.00000000000000000 ) ) ;
#17941=CARTESIAN_POINT ( 'NONE',  ( 158.0000000000003695, 173.3503748573662051, -45.00000000000000000 ) ) ;
#17942=CARTESIAN_POINT ( 'NONE',  ( 158.0000000000017337, 40.94087446699997912, 45.00000000000000000 ) ) ;
#17943=PLANE ( 'NONE',  #9411 ) ;
#17952=ORIENTED_EDGE ( 'NONE', *, *, #111, .T. ) ;
#17953=VERTEX_POINT ( 'NONE', #12863 ) ;
#17954=LINE ( 'NONE', #18105, #22923 ) ;
#17955=VECTOR ( 'NONE', #23491, 1000.000000000000114 ) ;
#17959=VERTEX_POINT ( 'NONE', #4221 ) ;
#17960=AXIS2_PLACEMENT_3D ( 'NONE', #507, #4941, #18457 ) ;
#17961=VERTEX_POINT ( 'NONE', #22179 ) ;
#17962=VECTOR ( 'NONE', #15815, 1000.000000000000000 ) ;
#17965=ADVANCED_FACE ( 'NONE', ( #8683 ), #2483, .F. ) ;
#17967=ORIENTED_EDGE ( 'NONE', *, *, #4979, .T. ) ;
#17969=LINE ( 'NONE', #16112, #15480 ) ;
#17970=DIRECTION ( 'NONE',  ( 0.000000000000000000, -1.000000000000000000, 0.000000000000000000 ) ) ;
#17975=EDGE_CURVE ( 'NONE', #13270, #21808, #23911, .T. ) ;
#17976=AXIS2_PLACEMENT_3D ( 'NONE', #8089, #3767, #8370 ) ;
#17981=AXIS2_PLACEMENT_3D ( 'NONE', #7259, #18179, #9560 ) ;
#17985=CARTESIAN_POINT ( 'NONE',  ( 158.0000000000005400, 156.3031248123239436, 45.00000000000000000 ) ) ;
#17988=VERTEX_POINT ( 'NONE', #13286 ) ;
#17992=ORIENTED_EDGE ( 'NONE', *, *, #5776, .T. ) ;
#17995=ORIENTED_EDGE ( 'NONE', *, *, #22962, .T. ) ;
#17996=AXIS2_PLACEMENT_3D ( 'NONE', #13978, #11953, #5043 ) ;
#17998=DIRECTION ( 'NONE',  ( -0.000000000000000000, -0.000000000000000000, -1.000000000000000000 ) ) ;
#18004=VECTOR ( 'NONE', #5442, 1000.000000000000000 ) ;
#18005=CARTESIAN_POINT ( 'NONE',  ( 158.0000000000015348, 58.49599951954928656, 45.00000000000000000 ) ) ;
#18006=EDGE_LOOP ( 'NONE', ( #4048, #26078, #20887, #22352 ) ) ;
#18008=EDGE_LOOP ( 'NONE', ( #6548, #11859, #21752, #3355 ) ) ;
#18011=LINE ( 'NONE', #22319, #4308 ) ;
#18014=VECTOR ( 'NONE', #9469, 1000.000000000000000 ) ;
#18017=CARTESIAN_POINT ( 'NONE',  ( 158.0000000000000568, 203.4448749474510407, -45.00000000000000000 ) ) ;
#18023=DIRECTION ( 'NONE',  ( -0.000000000000000000, -0.000000000000000000, -1.000000000000000000 ) ) ;
#18024=ORIENTED_EDGE ( 'NONE', *, *, #8179, .F. ) ;
#18025=CARTESIAN_POINT ( 'NONE',  ( 158.0000000000009663, 111.1613746771971876, 45.00000000000000000 ) ) ;
#18029=DIRECTION ( 'NONE',  ( -0.000000000000000000, -0.000000000000000000, -1.000000000000000000 ) ) ;
#18034=EDGE_LOOP ( 'NONE', ( #17929, #1137, #24443, #21210 ) ) ;
#18037=CARTESIAN_POINT ( 'NONE',  ( 158.0000000000011937, 91.09837461714084839, -45.00000000000000000 ) ) ;
#18038=ORIENTED_EDGE ( 'NONE', *, *, #10351, .T. ) ;
#18039=VECTOR ( 'NONE', #9535, 1000.000000000000114 ) ;
#18041=CARTESIAN_POINT ( 'NONE',  ( 158.0000000000012506, 88.08262460212675649, -45.00000000000000000 ) ) ;
#18050=EDGE_CURVE ( 'NONE', #8166, #7477, #6521, .T. ) ;
#18053=EDGE_CURVE ( 'NONE', #26626, #14606, #26337, .T. ) ;
#18054=CARTESIAN_POINT ( 'NONE',  ( 158.0000000000006537, 141.2558747672816821, -45.00000000000000000 ) ) ;
#18055=LINE ( 'NONE', #20908, #25047 ) ;
#18058=CARTESIAN_POINT ( 'NONE',  ( 157.4999999999998579, 201.1909374436971802, -45.00000000000000000 ) ) ;
#18060=DIRECTION ( 'NONE',  ( 0.000000000000000000, -1.000000000000000000, 0.000000000000000000 ) ) ;
#18065=LINE ( 'NONE', #537, #36 ) ;
#18071=ORIENTED_EDGE ( 'NONE', *, *, #10004, .T. ) ;
#18074=PLANE ( 'NONE',  #8171 ) ;
#18075=ORIENTED_EDGE ( 'NONE', *, *, #8817, .T. ) ;
#18078=ORIENTED_EDGE ( 'NONE', *, *, #6111, .F. ) ;
#18081=LINE ( 'NONE', #20372, #24678 ) ;
#18083=EDGE_CURVE ( 'NONE', #14664, #21625, #14006, .T. ) ;
#18091=LINE ( 'NONE', #13357, #19072 ) ;
#18093=LINE ( 'NONE', #423, #5766 ) ;
#18094=PLANE ( 'NONE',  #12638 ) ;
#18096=DIRECTION ( 'NONE',  ( -0.8916010070297244461, -0.4528218681375507093, 0.000000000000000000 ) ) ;
#18100=PLANE ( 'NONE',  #23448 ) ;
#18104=VECTOR ( 'NONE', #26733, 1000.000000000000000 ) ;
#18105=CARTESIAN_POINT ( 'NONE',  ( 157.4999999999998579, 105.8916871584295478, 45.00000000000000000 ) ) ;
#18107=VERTEX_POINT ( 'NONE', #20305 ) ;
#18111=DIRECTION ( 'NONE',  ( -0.000000000000000000, -0.000000000000000000, -1.000000000000000000 ) ) ;
#18113=ORIENTED_EDGE ( 'NONE', *, *, #1880, .F. ) ;
#18114=ORIENTED_EDGE ( 'NONE', *, *, #1539, .F. ) ;
#18115=DIRECTION ( 'NONE',  ( -0.000000000000000000, -0.000000000000000000, -1.000000000000000000 ) ) ;
#18117=EDGE_CURVE ( 'NONE', #14502, #21206, #7095, .T. ) ;
#18119=EDGE_LOOP ( 'NONE', ( #16184, #7848, #1477, #19831 ) ) ;
#18122=CARTESIAN_POINT ( 'NONE',  ( 167.4999999999996589, 258.6181251126050711, -5.999999999999991118 ) ) ;
#18123=LINE ( 'NONE', #7767, #4342 ) ;
#18130=DIRECTION ( 'NONE',  ( -0.000000000000000000, 0.000000000000000000, -1.000000000000000000 ) ) ;
#18134=VERTEX_POINT ( 'NONE', #3058 ) ;
#18135=CARTESIAN_POINT ( 'NONE',  ( 167.4999999999996589, 258.6181251126050711, 1.387778780781445676E-14 ) ) ;
#18138=ORIENTED_EDGE ( 'NONE', *, *, #5237, .T. ) ;
#18143=EDGE_CURVE ( 'NONE', #25694, #27854, #26917, .T. ) ;
#18144=EDGE_CURVE ( 'NONE', #28076, #16964, #7666, .T. ) ;
#18147=ORIENTED_EDGE ( 'NONE', *, *, #26969, .T. ) ;
#18148=VECTOR ( 'NONE', #27167, 1000.000000000000000 ) ;
#18149=ORIENTED_EDGE ( 'NONE', *, *, #22019, .T. ) ;
#18151=ORIENTED_EDGE ( 'NONE', *, *, #4425, .F. ) ;
#18154=FACE_OUTER_BOUND ( 'NONE', #28060, .T. ) ;
#18156=VECTOR ( 'NONE', #7527, 1000.000000000000000 ) ;
#18160=DIRECTION ( 'NONE',  ( -0.8916010070295213863, -0.4528218681379502786, 0.000000000000000000 ) ) ;
#18162=EDGE_CURVE ( 'NONE', #14089, #8924, #2629, .T. ) ;
#18164=CARTESIAN_POINT ( 'NONE',  ( 158.0000000000006253, 148.2716247822957882, 45.00000000000000000 ) ) ;
#18166=ADVANCED_FACE ( 'NONE', ( #1052 ), #9542, .F. ) ;
#18168=VECTOR ( 'NONE', #14414, 1000.000000000000000 ) ;
#18170=FACE_OUTER_BOUND ( 'NONE', #27719, .T. ) ;
#18176=DIRECTION ( 'NONE',  ( -0.8916010070298563406, -0.4528218681372909171, 0.000000000000000000 ) ) ;
#18178=ORIENTED_EDGE ( 'NONE', *, *, #1268, .T. ) ;
#18179=DIRECTION ( 'NONE',  ( 0.4528218681382856770, 0.8916010070293511891, -0.000000000000000000 ) ) ;
#18180=ORIENTED_EDGE ( 'NONE', *, *, #16500, .T. ) ;
#18182=DIRECTION ( 'NONE',  ( 0.4528218681382319422, 0.8916010070293783896, -0.000000000000000000 ) ) ;
#18184=LINE ( 'NONE', #18037, #5317 ) ;
#18185=ORIENTED_EDGE ( 'NONE', *, *, #6489, .T. ) ;
#18187=VECTOR ( 'NONE', #19972, 999.9999999999998863 ) ;
#18190=EDGE_CURVE ( 'NONE', #2723, #24747, #24907, .T. ) ;
#18194=EDGE_LOOP ( 'NONE', ( #6462, #11596, #11152, #18906 ) ) ;
#18196=VERTEX_POINT ( 'NONE', #5644 ) ;
#18198=DIRECTION ( 'NONE',  ( 0.000000000000000000, -1.000000000000000000, 0.000000000000000000 ) ) ;
#18201=DIRECTION ( 'NONE',  ( 0.4528218681383056610, -0.8916010070293409751, 0.000000000000000000 ) ) ;
#18202=CARTESIAN_POINT ( 'NONE',  ( 157.9999999999998295, 229.0315000300280417, 45.00000000000000000 ) ) ;
#18204=CARTESIAN_POINT ( 'NONE',  ( 157.4999999999998579, 43.19481197075347723, 45.00000000000000000 ) ) ;
#18206=CARTESIAN_POINT ( 'NONE',  ( 158.0000000000006821, 138.7479997597746433, 45.00000000000000000 ) ) ;
#18207=CARTESIAN_POINT ( 'NONE',  ( 158.0000000000003411, 175.8582498648732440, -45.00000000000000000 ) ) ;
#18208=VECTOR ( 'NONE', #21451, 1000.000000000000000 ) ;
#18209=ORIENTED_EDGE ( 'NONE', *, *, #9554, .F. ) ;
#18210=DIRECTION ( 'NONE',  ( -0.000000000000000000, 0.000000000000000000, -1.000000000000000000 ) ) ;
#18211=CARTESIAN_POINT ( 'NONE',  ( 157.9999999999998010, 231.5393750375350237, -45.00000000000000000 ) ) ;
#18221=ADVANCED_FACE ( 'NONE', ( #19135 ), #12550, .F. ) ;
#18233=CARTESIAN_POINT ( 'NONE',  ( 158.0000000000004832, 161.3188748273380213, 45.00000000000000000 ) ) ;
#18234=CARTESIAN_POINT ( 'NONE',  ( 158.0000000000009948, 108.6534996696901345, 45.00000000000000000 ) ) ;
#18235=CARTESIAN_POINT ( 'NONE',  ( 157.9999999999998579, 221.5078750075070104, 45.00000000000000000 ) ) ;
#18237=DIRECTION ( 'NONE',  ( 0.000000000000000000, -1.000000000000000000, 0.000000000000000000 ) ) ;
#18240=DIRECTION ( 'NONE',  ( 0.5150380749100565980, 1.049727191138616847E-16, 0.8571673007021108903 ) ) ;
#18243=ORIENTED_EDGE ( 'NONE', *, *, #7934, .T. ) ;
#18247=EDGE_CURVE ( 'NONE', #6570, #16387, #27744, .T. ) ;
#18248=CARTESIAN_POINT ( 'NONE',  ( 157.4999999999996589, 278.9350626764145318, 45.00000000000000000 ) ) ;
#18249=ORIENTED_EDGE ( 'NONE', *, *, #19704, .T. ) ;
#18250=ORIENTED_EDGE ( 'NONE', *, *, #4178, .T. ) ;
#18257=LINE ( 'NONE', #7621, #26604 ) ;
#18258=DIRECTION ( 'NONE',  ( -0.000000000000000000, 0.000000000000000000, -1.000000000000000000 ) ) ;
#18263=CARTESIAN_POINT ( 'NONE',  ( 157.4999999999998579, 58.24206201579573872, -45.00000000000000000 ) ) ;
#18264=CARTESIAN_POINT ( 'NONE',  ( 157.4999999999998579, 173.6043123611196961, 45.00000000000000000 ) ) ;
#18267=CARTESIAN_POINT ( 'NONE',  ( 157.9999999999997158, 261.1260001201120531, 45.00000000000000000 ) ) ;
#18269=DIRECTION ( 'NONE',  ( 0.8916010070294904111, -0.4528218681380115074, 0.000000000000000000 ) ) ;
#18274=AXIS2_PLACEMENT_3D ( 'NONE', #4719, #13503, #9187 ) ;
#18277=VECTOR ( 'NONE', #16018, 1000.000000000000000 ) ;
#18279=ORIENTED_EDGE ( 'NONE', *, *, #1779, .F. ) ;
#18281=APPLICATION_CONTEXT ( 'automotive_design' ) ;
#18284=EDGE_CURVE ( 'NONE', #15498, #24050, #25460, .T. ) ;
#18285=EDGE_LOOP ( 'NONE', ( #7360, #24614, #26620, #25441 ) ) ;
#18288=ADVANCED_FACE ( 'NONE', ( #23593 ), #3902, .F. ) ;
#18289=DIRECTION ( 'NONE',  ( -0.8916010070300181001, 0.4528218681369723386, 0.000000000000000000 ) ) ;
#18291=LINE ( 'NONE', #10090, #21510 ) ;
#18292=ORIENTED_EDGE ( 'NONE', *, *, #2369, .F. ) ;
#18293=CARTESIAN_POINT ( 'NONE',  ( 157.4999999999998579, 191.1594374136689964, 45.00000000000000000 ) ) ;
#18298=LINE ( 'NONE', #27048, #16781 ) ;
#18299=CARTESIAN_POINT ( 'NONE',  ( 157.4999999999998579, 80.81293708335913095, -45.00000000000000000 ) ) ;
#18306=DIRECTION ( 'NONE',  ( -0.8916010070293283185, -0.4528218681383305855, 0.000000000000000000 ) ) ;
#18308=CARTESIAN_POINT ( 'NONE',  ( 158.0000000000007674, 131.2243747372535267, 45.00000000000000000 ) ) ;
#18309=CARTESIAN_POINT ( 'NONE',  ( 158.0000000000014211, 73.03537455708450921, -45.00000000000000000 ) ) ;
#18310=ORIENTED_EDGE ( 'NONE', *, *, #13982, .F. ) ;
#18312=ORIENTED_EDGE ( 'NONE', *, *, #24814, .T. ) ;
#18313=EDGE_CURVE ( 'NONE', #23832, #12148, #14278, .T. ) ;
#18314=VECTOR ( 'NONE', #16991, 1000.000000000000000 ) ;
#18315=DIRECTION ( 'NONE',  ( -0.000000000000000000, -0.000000000000000000, -1.000000000000000000 ) ) ;
#18318=ORIENTED_EDGE ( 'NONE', *, *, #11095, .F. ) ;
#18319=DIRECTION ( 'NONE',  ( 0.8916010070299781320, 0.4528218681370510534, 0.000000000000000000 ) ) ;
#18321=VERTEX_POINT ( 'NONE', #3337 ) ;
#18323=CARTESIAN_POINT ( 'NONE',  ( 158.0000000000005969, 148.7794997898028271, -45.00000000000000000 ) ) ;
#18330=VERTEX_POINT ( 'NONE', #1191 ) ;
#18331=EDGE_CURVE ( 'NONE', #22237, #8556, #3761, .T. ) ;
#18333=EDGE_LOOP ( 'NONE', ( #25652, #9213, #6831, #15325 ) ) ;
#18336=DIRECTION ( 'NONE',  ( 0.000000000000000000, -1.000000000000000000, 0.000000000000000000 ) ) ;
#18338=LINE ( 'NONE', #7565, #15153 ) ;
#18342=PLANE ( 'NONE',  #12653 ) ;
#18343=DIRECTION ( 'NONE',  ( 1.000000000000000000, 0.000000000000000000, -0.000000000000000000 ) ) ;
#18344=DIRECTION ( 'NONE',  ( -0.000000000000000000, -0.000000000000000000, -1.000000000000000000 ) ) ;
#18346=LINE ( 'NONE', #7572, #19793 ) ;
#18350=AXIS2_PLACEMENT_3D ( 'NONE', #21957, #24544, #6872 ) ;
#18353=DIRECTION ( 'NONE',  ( 0.4528218681382463751, 0.8916010070293711731, -0.000000000000000000 ) ) ;
#18354=EDGE_CURVE ( 'NONE', #13425, #8035, #15947, .T. ) ;
#18355=CARTESIAN_POINT ( 'NONE',  ( 158.0000000000000853, 200.9369999399436892, 45.00000000000000000 ) ) ;
#18356=ORIENTED_EDGE ( 'NONE', *, *, #18726, .T. ) ;
#18359=ORIENTED_EDGE ( 'NONE', *, *, #9598, .T. ) ;
#18362=ORIENTED_EDGE ( 'NONE', *, *, #2367, .F. ) ;
#18363=ORIENTED_EDGE ( 'NONE', *, *, #11513, .T. ) ;
#18364=VERTEX_POINT ( 'NONE', #12975 ) ;
#18368=UNCERTAINTY_MEASURE_WITH_UNIT (LENGTH_MEASURE( 1.000000000000000082E-05 ), #8943, 'distance_accuracy_value', 'NONE');
#18380=ADVANCED_FACE ( 'NONE', ( #26695 ), #19566, .F. ) ;
#18381=VECTOR ( 'NONE', #27893, 1000.000000000000000 ) ;
#18383=DIRECTION ( 'NONE',  ( -0.000000000000000000, -0.000000000000000000, -1.000000000000000000 ) ) ;
#18387=FACE_OUTER_BOUND ( 'NONE', #2766, .T. ) ;
#18388=VERTEX_POINT ( 'NONE', #6487 ) ;
#18389=VERTEX_POINT ( 'NONE', #7175 ) ;
#18394=ORIENTED_EDGE ( 'NONE', *, *, #7241, .T. ) ;
#18395=ORIENTED_EDGE ( 'NONE', *, *, #24657, .T. ) ;
#18398=VECTOR ( 'NONE', #2134, 1000.000000000000000 ) ;
#18400=DIRECTION ( 'NONE',  ( -0.000000000000000000, -0.000000000000000000, -1.000000000000000000 ) ) ;
#18403=EDGE_CURVE ( 'NONE', #23120, #8173, #28168, .T. ) ;
#18407=CARTESIAN_POINT ( 'NONE',  ( 157.9999999999997442, 254.1102501050980322, 45.00000000000000000 ) ) ;
#18409=PLANE ( 'NONE',  #22537 ) ;
#18410=DIRECTION ( 'NONE',  ( -0.8916010070296124246, -0.4528218681377710886, 0.000000000000000000 ) ) ;
#18412=ORIENTED_EDGE ( 'NONE', *, *, #17487, .T. ) ;
#18416=LINE ( 'NONE', #27030, #18148 ) ;
#18419=ORIENTED_EDGE ( 'NONE', *, *, #1975, .T. ) ;
#18423=ORIENTED_EDGE ( 'NONE', *, *, #13077, .F. ) ;
#18427=DIRECTION ( 'NONE',  ( -0.000000000000000000, -0.000000000000000000, -1.000000000000000000 ) ) ;
#18428=VERTEX_POINT ( 'NONE', #26849 ) ;
#18429=PLANE ( 'NONE',  #21523 ) ;
#18430=ORIENTED_EDGE ( 'NONE', *, *, #20641, .T. ) ;
#18433=CARTESIAN_POINT ( 'NONE',  ( 158.0000000000012790, 85.57474959461971764, -45.00000000000000000 ) ) ;
#18434=EDGE_CURVE ( 'NONE', #27491, #583, #24697, .T. ) ;
#18436=EDGE_CURVE ( 'NONE', #17770, #18330, #9186, .T. ) ;
#18440=PLANE ( 'NONE',  #27905 ) ;
#18443=ORIENTED_EDGE ( 'NONE', *, *, #20641, .F. ) ;
#18444=FACE_OUTER_BOUND ( 'NONE', #24436, .T. ) ;
#18446=LINE ( 'NONE', #14146, #13407 ) ;
#18447=DIRECTION ( 'NONE',  ( -0.8916010070293409751, -0.4528218681383056610, 0.000000000000000000 ) ) ;
#18449=DIRECTION ( 'NONE',  ( -0.8916010070293483025, -0.4528218681382912281, 0.000000000000000000 ) ) ;
#18450=VERTEX_POINT ( 'NONE', #9333 ) ;
#18454=LINE ( 'NONE', #9969, #18814 ) ;
#18455=CARTESIAN_POINT ( 'NONE',  ( 217.4999999999996305, 258.6181251126050711, 6.000000000000019540 ) ) ;
#18457=DIRECTION ( 'NONE',  ( -0.000000000000000000, 0.000000000000000000, -1.000000000000000000 ) ) ;
#18463=ORIENTED_EDGE ( 'NONE', *, *, #16587, .F. ) ;
#18466=ORIENTED_EDGE ( 'NONE', *, *, #19, .F. ) ;
#18467=ORIENTED_EDGE ( 'NONE', *, *, #1210, .F. ) ;
#18469=AXIS2_PLACEMENT_3D ( 'NONE', #942, #22648, #2953 ) ;
#18470=CARTESIAN_POINT ( 'NONE',  ( 158.0000000000009663, 113.6692496847042264, 45.00000000000000000 ) ) ;
#18472=EDGE_CURVE ( 'NONE', #26566, #3490, #4863, .T. ) ;
#18473=VECTOR ( 'NONE', #9929, 1000.000000000000114 ) ;
#18475=FACE_OUTER_BOUND ( 'NONE', #10693, .T. ) ;
#18478=DIRECTION ( 'NONE',  ( -0.8916010070296327417, -0.4528218681377311761, 0.000000000000000000 ) ) ;
#18480=FACE_OUTER_BOUND ( 'NONE', #6634, .T. ) ;
#18481=LINE ( 'NONE', #22930, #14515 ) ;
#18485=ORIENTED_EDGE ( 'NONE', *, *, #24404, .F. ) ;
#18486=ADVANCED_FACE ( 'NONE', ( #11497 ), #15124, .F. ) ;
#18488=DIRECTION ( 'NONE',  ( -0.8916010070293483025, -0.4528218681382912281, 0.000000000000000000 ) ) ;
#18489=CARTESIAN_POINT ( 'NONE',  ( 157.4999999999998579, 100.8759371434154701, 45.00000000000000000 ) ) ;
#18492=VECTOR ( 'NONE', #7972, 1000.000000000000227 ) ;
#18496=DIRECTION ( 'NONE',  ( 0.8916010070293995948, 0.4528218681381900312, 0.000000000000000000 ) ) ;
#18497=VECTOR ( 'NONE', #9044, 1000.000000000000000 ) ;
#18498=EDGE_CURVE ( 'NONE', #9774, #23905, #20383, .T. ) ;
#18499=ORIENTED_EDGE ( 'NONE', *, *, #2297, .T. ) ;
#18505=VERTEX_POINT ( 'NONE', #7601 ) ;
#18507=CARTESIAN_POINT ( 'NONE',  ( 158.0000000000000853, 196.4291249324366504, -45.00000000000000000 ) ) ;
#18511=VECTOR ( 'NONE', #10768, 1000.000000000000000 ) ;
#18514=LINE ( 'NONE', #22687, #12223 ) ;
#18518=VECTOR ( 'NONE', #19776, 1000.000000000000000 ) ;
#18519=FACE_OUTER_BOUND ( 'NONE', #12191, .T. ) ;
#18527=ORIENTED_EDGE ( 'NONE', *, *, #11660, .T. ) ;
#18529=ORIENTED_EDGE ( 'NONE', *, *, #28285, .T. ) ;
#18530=VECTOR ( 'NONE', #12655, 1000.000000000000000 ) ;
#18534=VERTEX_POINT ( 'NONE', #11786 ) ;
#18537=DIRECTION ( 'NONE',  ( 1.000000000000000000, 0.000000000000000000, -0.000000000000000000 ) ) ;
#18541=LINE ( 'NONE', #18122, #27235 ) ;
#18544=CARTESIAN_POINT ( 'NONE',  ( 157.9999999999996874, 266.1417501351260171, -45.00000000000000000 ) ) ;
#18546=VECTOR ( 'NONE', #7455, 1000.000000000000114 ) ;
#18551=FACE_OUTER_BOUND ( 'NONE', #19757, .T. ) ;
#18553=CARTESIAN_POINT ( 'NONE',  ( 157.4999999999996589, 278.9350626764145318, -45.00000000000000000 ) ) ;
#18558=VERTEX_POINT ( 'NONE', #23248 ) ;
#18562=EDGE_CURVE ( 'NONE', #4740, #21445, #27129, .T. ) ;
#18564=ORIENTED_EDGE ( 'NONE', *, *, #25247, .F. ) ;
#18565=EDGE_CURVE ( 'NONE', #2405, #12219, #1405, .T. ) ;
#18566=ADVANCED_FACE ( 'NONE', ( #26986 ), #18791, .F. ) ;
#18567=CARTESIAN_POINT ( 'NONE',  ( 158.0000000000009379, 116.1771246922112653, 45.00000000000000000 ) ) ;
#18569=FACE_OUTER_BOUND ( 'NONE', #15461, .T. ) ;
#18572=VERTEX_POINT ( 'NONE', #22690 ) ;
#18575=LINE ( 'NONE', #25455, #22732 ) ;
#18578=CARTESIAN_POINT ( 'NONE',  ( 157.9999999999996305, 286.2047501951820436, 45.00000000000000000 ) ) ;
#18579=CARTESIAN_POINT ( 'NONE',  ( 158.0000000000008811, 121.1928747072253572, 45.00000000000000000 ) ) ;
#18582=CARTESIAN_POINT ( 'NONE',  ( 158.0000000000004832, 161.3188748273380213, -45.00000000000000000 ) ) ;
#18586=VECTOR ( 'NONE', #16809, 1000.000000000000000 ) ;
#18591=ORIENTED_EDGE ( 'NONE', *, *, #1400, .F. ) ;
#18592=CARTESIAN_POINT ( 'NONE',  ( 158.0000000000008811, 123.1928747072253572, -45.00000000000000000 ) ) ;
#18594=ORIENTED_EDGE ( 'NONE', *, *, #5323, .F. ) ;
#18596=ADVANCED_FACE ( 'NONE', ( #18519 ), #22829, .F. ) ;
#18599=ORIENTED_EDGE ( 'NONE', *, *, #21294, .F. ) ;
#18601=CARTESIAN_POINT ( 'NONE',  ( 158.0000000000006821, 140.7479997597746433, 45.00000000000000000 ) ) ;
#18605=ORIENTED_EDGE ( 'NONE', *, *, #23272, .T. ) ;
#18609=DIRECTION ( 'NONE',  ( -0.8916010070293483025, -0.4528218681382912281, 0.000000000000000000 ) ) ;
#18611=DIRECTION ( 'NONE',  ( -0.000000000000000000, -0.000000000000000000, -1.000000000000000000 ) ) ;
#18615=CARTESIAN_POINT ( 'NONE',  ( 158.0000000000001705, 188.9054999099155054, -45.00000000000000000 ) ) ;
#18620=VERTEX_POINT ( 'NONE', #23527 ) ;
#18623=VECTOR ( 'NONE', #15375, 1000.000000000000000 ) ;
#18626=ADVANCED_FACE ( 'NONE', ( #21652 ), #3842, .F. ) ;
#18631=CARTESIAN_POINT ( 'NONE',  ( 157.4999999999998579, 198.6830624361901414, 45.00000000000000000 ) ) ;
#18632=ORIENTED_EDGE ( 'NONE', *, *, #20375, .F. ) ;
#18648=LINE ( 'NONE', #27391, #10478 ) ;
#18652=VECTOR ( 'NONE', #23211, 1000.000000000000114 ) ;
#18654=DIRECTION ( 'NONE',  ( -0.8916010070294605461, -0.4528218681380702382, 0.000000000000000000 ) ) ;
#18656=EDGE_CURVE ( 'NONE', #4479, #21343, #25816, .T. ) ;
#18659=CARTESIAN_POINT ( 'NONE',  ( 158.0000000000004547, 165.8267498348450886, -45.00000000000000000 ) ) ;
#18660=ORIENTED_EDGE ( 'NONE', *, *, #14481, .F. ) ;
#18661=ORIENTED_EDGE ( 'NONE', *, *, #18436, .F. ) ;
#18662=EDGE_CURVE ( 'NONE', #5675, #13193, #10597, .T. ) ;
#18663=CARTESIAN_POINT ( 'NONE',  ( 158.0000000000008527, 125.7007497147323818, 45.00000000000000000 ) ) ;
#18665=ORIENTED_EDGE ( 'NONE', *, *, #376, .T. ) ;
#18666=AXIS2_PLACEMENT_3D ( 'NONE', #25904, #6226, #10828 ) ;
#18667=EDGE_LOOP ( 'NONE', ( #2806, #3823, #16724, #81 ) ) ;
#18669=ORIENTED_EDGE ( 'NONE', *, *, #418, .F. ) ;
#18672=EDGE_CURVE ( 'NONE', #14862, #11476, #25675, .T. ) ;
#18678=DIRECTION ( 'NONE',  ( 1.000000000000000000, 0.000000000000000000, -0.000000000000000000 ) ) ;
#18684=DIRECTION ( 'NONE',  ( 0.8916010070296023216, -0.4528218681377911281, 0.000000000000000000 ) ) ;
#18686=EDGE_LOOP ( 'NONE', ( #24917, #3810, #22603, #26344 ) ) ;
#18687=EDGE_CURVE ( 'NONE', #8486, #1213, #19215, .T. ) ;
#18690=CARTESIAN_POINT ( 'NONE',  ( 157.4999999999996874, 268.9035626463865469, 45.00000000000000000 ) ) ;
#18696=VECTOR ( 'NONE', #27157, 1000.000000000000000 ) ;
#18697=DIRECTION ( 'NONE',  ( 0.000000000000000000, -1.000000000000000000, 0.000000000000000000 ) ) ;
#18698=CARTESIAN_POINT ( 'NONE',  ( 157.4999999999998579, 156.0491873085704242, -45.00000000000000000 ) ) ;
#18702=DIRECTION ( 'NONE',  ( -0.000000000000000000, 0.000000000000000000, -1.000000000000000000 ) ) ;
#18713=CARTESIAN_POINT ( 'NONE',  ( 157.4999999999998579, 125.9546872184859012, 45.00000000000000000 ) ) ;
#18716=AXIS2_PLACEMENT_3D ( 'NONE', #27130, #6881, #7176 ) ;
#18717=ORIENTED_EDGE ( 'NONE', *, *, #11274, .F. ) ;
#18719=AXIS2_PLACEMENT_3D ( 'NONE', #6344, #8653, #4330 ) ;
#18720=LINE ( 'NONE', #16574, #15185 ) ;
#18722=DIRECTION ( 'NONE',  ( 0.4528218681383106015, 0.8916010070293384215, -0.000000000000000000 ) ) ;
#18723=VERTEX_POINT ( 'NONE', #532 ) ;
#18725=LINE ( 'NONE', #1200, #9600 ) ;
#18726=EDGE_CURVE ( 'NONE', #15277, #27632, #4540, .T. ) ;
#18727=ORIENTED_EDGE ( 'NONE', *, *, #11968, .T. ) ;
#18729=CARTESIAN_POINT ( 'NONE',  ( 157.9999999999999147, 213.9842499849850697, 45.00000000000000000 ) ) ;
#18732=DIRECTION ( 'NONE',  ( 0.4528218681381301347, -0.8916010070294301260, 0.000000000000000000 ) ) ;
#18733=EDGE_LOOP ( 'NONE', ( #22313, #12460, #4207, #15826 ) ) ;
#18734=LINE ( 'NONE', #18323, #20788 ) ;
#18739=DIRECTION ( 'NONE',  ( 0.000000000000000000, -1.000000000000000000, 0.000000000000000000 ) ) ;
#18741=AXIS2_PLACEMENT_3D ( 'NONE', #2243, #15487, #4120 ) ;
#18742=ADVANCED_FACE ( 'NONE', ( #17909 ), #15486, .F. ) ;
#18744=ORIENTED_EDGE ( 'NONE', *, *, #20699, .F. ) ;
#18751=PLANE ( 'NONE',  #8826 ) ;
#18752=VECTOR ( 'NONE', #11384, 1000.000000000000000 ) ;
#18754=EDGE_CURVE ( 'NONE', #12868, #18572, #17626, .T. ) ;
#18759=ADVANCED_FACE ( 'NONE', ( #8723 ), #4403, .F. ) ;
#18761=AXIS2_PLACEMENT_3D ( 'NONE', #3446, #3725, #25562 ) ;
#18762=ADVANCED_FACE ( 'NONE', ( #6989 ), #4827, .F. ) ;
#18767=FACE_OUTER_BOUND ( 'NONE', #18686, .T. ) ;
#18770=LINE ( 'NONE', #25232, #17115 ) ;
#18771=ORIENTED_EDGE ( 'NONE', *, *, #9594, .T. ) ;
#18773=ORIENTED_EDGE ( 'NONE', *, *, #24507, .F. ) ;
#18775=AXIS2_PLACEMENT_3D ( 'NONE', #15171, #21903, #9115 ) ;
#18791=PLANE ( 'NONE',  #957 ) ;
#18796=EDGE_CURVE ( 'NONE', #9114, #9224, #11025, .T. ) ;
#18804=ORIENTED_EDGE ( 'NONE', *, *, #23231, .F. ) ;
#18808=ORIENTED_EDGE ( 'NONE', *, *, #21111, .F. ) ;
#18811=AXIS2_PLACEMENT_3D ( 'NONE', #4114, #21644, #1956 ) ;
#18814=VECTOR ( 'NONE', #1483, 1000.000000000000000 ) ;
#18816=EDGE_CURVE ( 'NONE', #3560, #4902, #249, .T. ) ;
#18818=LINE ( 'NONE', #8184, #15099 ) ;
#18820=CARTESIAN_POINT ( 'NONE',  ( 157.9999999999998010, 236.5551250525490161, 45.00000000000000000 ) ) ;
#18822=DIRECTION ( 'NONE',  ( -0.000000000000000000, -0.000000000000000000, -1.000000000000000000 ) ) ;
#18826=EDGE_CURVE ( 'NONE', #11076, #17424, #17762, .T. ) ;
#18832=ORIENTED_EDGE ( 'NONE', *, *, #10100, .F. ) ;
#18834=AXIS2_PLACEMENT_3D ( 'NONE', #9156, #15778, #2111 ) ;
#18835=LINE ( 'NONE', #14965, #9722 ) ;
#18838=VERTEX_POINT ( 'NONE', #24663 ) ;
#18840=LINE ( 'NONE', #14541, #14103 ) ;
#18841=EDGE_CURVE ( 'NONE', #26462, #12700, #2383, .T. ) ;
#18849=LINE ( 'NONE', #27319, #2553 ) ;
#18851=CARTESIAN_POINT ( 'NONE',  ( 157.9999999999997442, 251.0945000900840398, 45.00000000000000000 ) ) ;
#18852=LINE ( 'NONE', #7800, #4861 ) ;
#18853=FACE_OUTER_BOUND ( 'NONE', #2432, .T. ) ;
#18857=ORIENTED_EDGE ( 'NONE', *, *, #28176, .T. ) ;
#18859=DIRECTION ( 'NONE',  ( 1.000000000000000000, 0.000000000000000000, -0.000000000000000000 ) ) ;
#18860=CARTESIAN_POINT ( 'NONE',  ( 158.0000000000005400, 158.3031248123239436, -45.00000000000000000 ) ) ;
#18868=ORIENTED_EDGE ( 'NONE', *, *, #8314, .F. ) ;
#18869=CARTESIAN_POINT ( 'NONE',  ( 158.0000000000012221, 90.59049960963380954, -45.00000000000000000 ) ) ;
#18873=LINE ( 'NONE', #23328, #21645 ) ;
#18876=VECTOR ( 'NONE', #14155, 1000.000000000000114 ) ;
#18877=ORIENTED_EDGE ( 'NONE', *, *, #18162, .F. ) ;
#18879=ORIENTED_EDGE ( 'NONE', *, *, #15463, .T. ) ;
#18880=AXIS2_PLACEMENT_3D ( 'NONE', #5125, #25230, #12036 ) ;
#18884=DIRECTION ( 'NONE',  ( 0.000000000000000000, -1.000000000000000000, 0.000000000000000000 ) ) ;
#18894=DIRECTION ( 'NONE',  ( -0.8916010070298868717, -0.4528218681372309651, 0.000000000000000000 ) ) ;
#18895=DIRECTION ( 'NONE',  ( 0.4528218681377311206, 0.8916010070296327417, -0.000000000000000000 ) ) ;
#18900=CARTESIAN_POINT ( 'NONE',  ( 158.0000000000009379, 118.1771246922112653, 45.00000000000000000 ) ) ;
#18901=VECTOR ( 'NONE', #15030, 1000.000000000000000 ) ;
#18903=LINE ( 'NONE', #27370, #14910 ) ;
#18905=LINE ( 'NONE', #3814, #17074 ) ;
#18906=ORIENTED_EDGE ( 'NONE', *, *, #16066, .T. ) ;
#18907=DIRECTION ( 'NONE',  ( 0.000000000000000000, -1.000000000000000000, 0.000000000000000000 ) ) ;
#18910=FACE_OUTER_BOUND ( 'NONE', #513, .T. ) ;
#18913=ORIENTED_EDGE ( 'NONE', *, *, #17253, .F. ) ;
#18916=ORIENTED_EDGE ( 'NONE', *, *, #3310, .T. ) ;
#18917=EDGE_CURVE ( 'NONE', #25403, #21137, #1231, .T. ) ;
#18925=EDGE_CURVE ( 'NONE', #12219, #5230, #18346, .T. ) ;
#18931=CARTESIAN_POINT ( 'NONE',  ( 157.4999999999998295, 226.2696875187675118, 45.00000000000000000 ) ) ;
#18939=DIRECTION ( 'NONE',  ( -0.8916010070294301260, -0.4528218681381301347, 0.000000000000000000 ) ) ;
#18943=ORIENTED_EDGE ( 'NONE', *, *, #6435, .T. ) ;
#18947=VERTEX_POINT ( 'NONE', #5686 ) ;
#18952=ORIENTED_EDGE ( 'NONE', *, *, #22325, .F. ) ;
#18954=VECTOR ( 'NONE', #25454, 1000.000000000000000 ) ;
#18958=CARTESIAN_POINT ( 'NONE',  ( 157.4999999999998579, 113.4153121809506786, 45.00000000000000000 ) ) ;
#18963=CARTESIAN_POINT ( 'NONE',  ( 158.0000000000013642, 78.05112457209858690, 45.00000000000000000 ) ) ;
#18964=LINE ( 'NONE', #27707, #13430 ) ;
#18969=ORIENTED_EDGE ( 'NONE', *, *, #23480, .T. ) ;
#18971=LINE ( 'NONE', #12666, #9163 ) ;
#18973=CARTESIAN_POINT ( 'NONE',  ( 157.9999999999998295, 224.0157500150140208, -45.00000000000000000 ) ) ;
#18979=EDGE_CURVE ( 'NONE', #800, #20034, #5262, .T. ) ;
#18980=LINE ( 'NONE', #3459, #996 ) ;
#18981=DIRECTION ( 'NONE',  ( 0.000000000000000000, -1.000000000000000000, 0.000000000000000000 ) ) ;
#18984=PLANE ( 'NONE',  #1700 ) ;
#18986=PLANE ( 'NONE',  #26543 ) ;
#18992=EDGE_CURVE ( 'NONE', #21166, #10546, #21470, .T. ) ;
#18993=EDGE_CURVE ( 'NONE', #8245, #9774, #25922, .T. ) ;
#18994=DIRECTION ( 'NONE',  ( 0.8916010070300078860, -0.4528218681369923782, 0.000000000000000000 ) ) ;
#19000=LINE ( 'NONE', #8225, #22502 ) ;
#19001=VERTEX_POINT ( 'NONE', #27921 ) ;
#19004=DIRECTION ( 'NONE',  ( -0.000000000000000000, -0.000000000000000000, -1.000000000000000000 ) ) ;
#19005=CARTESIAN_POINT ( 'NONE',  ( 157.9999999999997442, 256.1102501050980322, -45.00000000000000000 ) ) ;
#19007=ADVANCED_FACE ( 'NONE', ( #28207 ), #19038, .F. ) ;
#19010=ADVANCED_FACE ( 'NONE', ( #7981 ), #14594, .F. ) ;
#19012=DIRECTION ( 'NONE',  ( -0.000000000000000000, 0.000000000000000000, -1.000000000000000000 ) ) ;
#19014=ORIENTED_EDGE ( 'NONE', *, *, #3921, .T. ) ;
#19016=DIRECTION ( 'NONE',  ( -0.000000000000000000, 0.000000000000000000, -1.000000000000000000 ) ) ;
#19028=EDGE_CURVE ( 'NONE', #14759, #83, #12309, .T. ) ;
#19029=EDGE_CURVE ( 'NONE', #6262, #18388, #23350, .T. ) ;
#19033=LINE ( 'NONE', #14880, #14253 ) ;
#19038=PLANE ( 'NONE',  #21619 ) ;
#19042=EDGE_CURVE ( 'NONE', #19942, #19398, #1512, .T. ) ;
#19047=VERTEX_POINT ( 'NONE', #21047 ) ;
#19051=ORIENTED_EDGE ( 'NONE', *, *, #25300, .T. ) ;
#19052=CARTESIAN_POINT ( 'NONE',  ( 157.4999999999998579, 68.27356204582390831, 45.00000000000000000 ) ) ;
#19053=VERTEX_POINT ( 'NONE', #16883 ) ;
#19057=ORIENTED_EDGE ( 'NONE', *, *, #18050, .T. ) ;
#19060=VECTOR ( 'NONE', #150, 1000.000000000000000 ) ;
#19061=VERTEX_POINT ( 'NONE', #10282 ) ;
#19064=CARTESIAN_POINT ( 'NONE',  ( 157.9999999999996305, 283.6968751876750616, -45.00000000000000000 ) ) ;
#19068=DIRECTION ( 'NONE',  ( 0.000000000000000000, -1.000000000000000000, 0.000000000000000000 ) ) ;
#19072=VECTOR ( 'NONE', #26692, 1000.000000000000000 ) ;
#19073=LINE ( 'NONE', #25674, #1169 ) ;
#19074=CARTESIAN_POINT ( 'NONE',  ( 158.0000000000005684, 153.2873747973098659, 45.00000000000000000 ) ) ;
#19076=VECTOR ( 'NONE', #7568, 1000.000000000000000 ) ;
#19077=CARTESIAN_POINT ( 'NONE',  ( 158.0000000000016200, 52.97237449702815582, 45.00000000000000000 ) ) ;
#19085=ADVANCED_FACE ( 'NONE', ( #8553 ), #23772, .F. ) ;
#19086=EDGE_CURVE ( 'NONE', #16305, #17073, #3660, .T. ) ;
#19088=EDGE_CURVE ( 'NONE', #26586, #17489, #27644, .T. ) ;
#19090=ORIENTED_EDGE ( 'NONE', *, *, #12489, .F. ) ;
#19094=ORIENTED_EDGE ( 'NONE', *, *, #23272, .F. ) ;
#19100=DIRECTION ( 'NONE',  ( 0.4528218681377311206, -0.8916010070296327417, 0.000000000000000000 ) ) ;
#19103=DIRECTION ( 'NONE',  ( 0.8916010070298867607, 0.4528218681372308541, 0.000000000000000000 ) ) ;
#19104=CARTESIAN_POINT ( 'NONE',  ( 187.4999999999996305, 40.68693696324645970, -45.00000000000000000 ) ) ;
#19107=CARTESIAN_POINT ( 'NONE',  ( 157.4999999999995737, 203.6988124512014338, 45.00000000000000000 ) ) ;
#19108=DIRECTION ( 'NONE',  ( 0.8916010070293783896, -0.4528218681382319422, 0.000000000000000000 ) ) ;
#19112=EDGE_CURVE ( 'NONE', #21343, #7910, #25637, .T. ) ;
#19113=EDGE_CURVE ( 'NONE', #10576, #2123, #6804, .T. ) ;
#19115=ORIENTED_EDGE ( 'NONE', *, *, #2323, .T. ) ;
#19117=VERTEX_POINT ( 'NONE', #28342 ) ;
#19118=EDGE_LOOP ( 'NONE', ( #19339, #7780, #21390, #16553 ) ) ;
#19120=DIRECTION ( 'NONE',  ( -0.8916010070297852863, -0.4528218681374307497, 0.000000000000000000 ) ) ;
#19121=ORIENTED_EDGE ( 'NONE', *, *, #7556, .T. ) ;
#19122=VERTEX_POINT ( 'NONE', #2636 ) ;
#19123=DIRECTION ( 'NONE',  ( 0.8916010070294395629, -0.4528218681381114274, 0.000000000000000000 ) ) ;
#19125=DIRECTION ( 'NONE',  ( -0.8916010070299577039, -0.4528218681370910215, 0.000000000000000000 ) ) ;
#19130=CARTESIAN_POINT ( 'NONE',  ( 157.9999999999996305, 284.2047501951820436, -45.00000000000000000 ) ) ;
#19132=PLANE ( 'NONE',  #20393 ) ;
#19134=DIRECTION ( 'NONE',  ( 0.8916010070296429557, 0.4528218681377111920, 0.000000000000000000 ) ) ;
#19135=FACE_OUTER_BOUND ( 'NONE', #3537, .T. ) ;
#19137=EDGE_CURVE ( 'NONE', #22238, #17429, #15586, .T. ) ;
#19141=DIRECTION ( 'NONE',  ( 0.000000000000000000, -1.000000000000000000, 0.000000000000000000 ) ) ;
#19142=CARTESIAN_POINT ( 'NONE',  ( 157.4999999999998579, 53.22631200078164682, 45.00000000000000000 ) ) ;
#19144=CARTESIAN_POINT ( 'NONE',  ( 157.4999999999998579, 70.78143705333094715, 45.00000000000000000 ) ) ;
#19145=ADVANCED_FACE ( 'NONE', ( #26201 ), #10989, .F. ) ;
#19146=FACE_OUTER_BOUND ( 'NONE', #6532, .T. ) ;
#19147=LINE ( 'NONE', #10819, #13338 ) ;
#19148=DIRECTION ( 'NONE',  ( -0.000000000000000000, -0.000000000000000000, -1.000000000000000000 ) ) ;
#19149=ORIENTED_EDGE ( 'NONE', *, *, #2643, .T. ) ;
#19151=CARTESIAN_POINT ( 'NONE',  ( 157.4999999999998579, 53.22631200078164682, 45.00000000000000000 ) ) ;
#19152=VERTEX_POINT ( 'NONE', #24333 ) ;
#19156=CARTESIAN_POINT ( 'NONE',  ( 158.0000000000002274, 185.8897498949014278, -45.00000000000000000 ) ) ;
#19157=ORIENTED_EDGE ( 'NONE', *, *, #21887, .T. ) ;
#19159=CARTESIAN_POINT ( 'NONE',  ( 157.4999999999998579, 70.78143705333094715, 45.00000000000000000 ) ) ;
#19160=ORIENTED_EDGE ( 'NONE', *, *, #9358, .F. ) ;
#19161=ORIENTED_EDGE ( 'NONE', *, *, #3620, .T. ) ;
#19162=VERTEX_POINT ( 'NONE', #6527 ) ;
#19164=LINE ( 'NONE', #8540, #19400 ) ;
#19166=CARTESIAN_POINT ( 'NONE',  ( 158.0000000000000853, 196.4291249324366504, 45.00000000000000000 ) ) ;
#19168=FACE_OUTER_BOUND ( 'NONE', #1127, .T. ) ;
#19169=CARTESIAN_POINT ( 'NONE',  ( 157.9999999999998010, 239.0630000600560550, -45.00000000000000000 ) ) ;
#19172=ORIENTED_EDGE ( 'NONE', *, *, #4838, .F. ) ;
#19175=DIRECTION ( 'NONE',  ( -0.000000000000000000, -0.000000000000000000, -1.000000000000000000 ) ) ;
#19178=CARTESIAN_POINT ( 'NONE',  ( 157.9999999999996589, 281.1890001801680796, 45.00000000000000000 ) ) ;
#19180=CARTESIAN_POINT ( 'NONE',  ( 158.0000000000001137, 193.9212499249295831, -45.00000000000000000 ) ) ;
#19182=PLANE ( 'NONE',  #19473 ) ;
#19184=LINE ( 'NONE', #27931, #5142 ) ;
#19185=ORIENTED_EDGE ( 'NONE', *, *, #17328, .T. ) ;
#19187=EDGE_CURVE ( 'NONE', #7590, #1943, #11279, .T. ) ;
#19190=EDGE_CURVE ( 'NONE', #2326, #27871, #22183, .T. ) ;
#19191=DIRECTION ( 'NONE',  ( 0.4528218681382912836, -0.8916010070293483025, 0.000000000000000000 ) ) ;
#19195=CARTESIAN_POINT ( 'NONE',  ( 158.0000000000015348, 60.49599951954928656, 45.00000000000000000 ) ) ;
#19199=EDGE_CURVE ( 'NONE', #16733, #9066, #353, .T. ) ;
#19200=DIRECTION ( 'NONE',  ( -0.000000000000000000, -0.000000000000000000, -1.000000000000000000 ) ) ;
#19203=DIRECTION ( 'NONE',  ( -0.000000000000000000, 0.000000000000000000, -1.000000000000000000 ) ) ;
#19205=CARTESIAN_POINT ( 'NONE',  ( 158.0000000000005116, 160.8109998198309825, 45.00000000000000000 ) ) ;
#19210=PRODUCT ( 'Gear Rack', 'Gear Rack', '', ( #26145 ) ) ;
#19213=DIRECTION ( 'NONE',  ( 0.000000000000000000, -1.000000000000000000, 0.000000000000000000 ) ) ;
#19214=EDGE_CURVE ( 'NONE', #25157, #15447, #26623, .T. ) ;
#19215=LINE ( 'NONE', #8447, #1881 ) ;
#19219=VECTOR ( 'NONE', #17255, 1000.000000000000000 ) ;
#19220=DIRECTION ( 'NONE',  ( 0.000000000000000000, -1.000000000000000000, 0.000000000000000000 ) ) ;
#19221=CARTESIAN_POINT ( 'NONE',  ( 167.4999999999996589, 258.6181251126050711, -5.999999999999991118 ) ) ;
#19222=CARTESIAN_POINT ( 'NONE',  ( 158.0000000000005969, 148.7794997898028271, 45.00000000000000000 ) ) ;
#19229=AXIS2_PLACEMENT_3D ( 'NONE', #4417, #22089, #19933 ) ;
#19230=ORIENTED_EDGE ( 'NONE', *, *, #17888, .F. ) ;
#19235=DIRECTION ( 'NONE',  ( -0.8916010070293409751, -0.4528218681383056610, 0.000000000000000000 ) ) ;
#19240=ADVANCED_FACE ( 'NONE', ( #24197 ), #19739, .F. ) ;
#19242=VECTOR ( 'NONE', #579, 1000.000000000000000 ) ;
#19243=VECTOR ( 'NONE', #12458, 1000.000000000000000 ) ;
#19245=LINE ( 'NONE', #16535, #28375 ) ;
#19247=AXIS2_PLACEMENT_3D ( 'NONE', #21770, #23641, #2077 ) ;
#19252=ORIENTED_EDGE ( 'NONE', *, *, #15652, .F. ) ;
#19254=AXIS2_PLACEMENT_3D ( 'NONE', #12336, #8293, #17752 ) ;
#19255=PLANE ( 'NONE',  #8969 ) ;
#19258=ORIENTED_EDGE ( 'NONE', *, *, #20375, .T. ) ;
#19259=ORIENTED_EDGE ( 'NONE', *, *, #25914, .T. ) ;
#19261=EDGE_CURVE ( 'NONE', #26578, #855, #24483, .T. ) ;
#19262=CARTESIAN_POINT ( 'NONE',  ( 157.9999999999996589, 274.1732501651540588, -45.00000000000000000 ) ) ;
#19269=LINE ( 'NONE', #15258, #4997 ) ;
#19270=ORIENTED_EDGE ( 'NONE', *, *, #23888, .T. ) ;
#19277=ADVANCED_FACE ( 'NONE', ( #26921 ), #9686, .F. ) ;
#19282=VECTOR ( 'NONE', #7977, 999.9999999999998863 ) ;
#19283=DIRECTION ( 'NONE',  ( 0.000000000000000000, -1.000000000000000000, 0.000000000000000000 ) ) ;
#19285=PLANE ( 'NONE',  #19811 ) ;
#19287=ORIENTED_EDGE ( 'NONE', *, *, #7211, .T. ) ;
#19290=LINE ( 'NONE', #19432, #13006 ) ;
#19300=LINE ( 'NONE', #16454, #16821 ) ;
#19302=VERTEX_POINT ( 'NONE', #643 ) ;
#19305=EDGE_CURVE ( 'NONE', #12668, #7560, #27331, .T. ) ;
#19307=VERTEX_POINT ( 'NONE', #3344 ) ;
#19308=PLANE ( 'NONE',  #20778 ) ;
#19310=EDGE_CURVE ( 'NONE', #25194, #477, #11714, .T. ) ;
#19314=LINE ( 'NONE', #10138, #3690 ) ;
#19317=LINE ( 'NONE', #3518, #17721 ) ;
#19318=DIRECTION ( 'NONE',  ( -0.8916010070293584056, 0.4528218681382713551, 0.000000000000000000 ) ) ;
#19320=LINE ( 'NONE', #25924, #25860 ) ;
#19321=ORIENTED_EDGE ( 'NONE', *, *, #20957, .F. ) ;
#19323=VECTOR ( 'NONE', #27957, 1000.000000000000000 ) ;
#19328=CARTESIAN_POINT ( 'NONE',  ( 157.4999999999997726, 248.8405625863305204, 45.00000000000000000 ) ) ;
#19332=ORIENTED_EDGE ( 'NONE', *, *, #4030, .F. ) ;
#19333=LINE ( 'NONE', #25936, #19527 ) ;
#19336=DIRECTION ( 'NONE',  ( -0.000000000000000000, 0.000000000000000000, -1.000000000000000000 ) ) ;
#19337=EDGE_CURVE ( 'NONE', #8321, #18107, #18446, .T. ) ;
#19339=ORIENTED_EDGE ( 'NONE', *, *, #22325, .T. ) ;
#19344=VECTOR ( 'NONE', #20142, 1000.000000000000000 ) ;
#19346=VECTOR ( 'NONE', #2970, 1000.000000000000000 ) ;
#19355=FACE_OUTER_BOUND ( 'NONE', #25692, .T. ) ;
#19356=CARTESIAN_POINT ( 'NONE',  ( 157.4999999999998579, 166.0806873385985796, 45.00000000000000000 ) ) ;
#19359=LINE ( 'NONE', #6431, #28187 ) ;
#19362=EDGE_LOOP ( 'NONE', ( #10802, #3826, #8283, #4364 ) ) ;
#19365=VECTOR ( 'NONE', #16957, 1000.000000000000000 ) ;
#19373=VECTOR ( 'NONE', #21199, 1000.000000000000000 ) ;
#19382=EDGE_CURVE ( 'NONE', #5381, #16287, #3062, .T. ) ;
#19383=VECTOR ( 'NONE', #7181, 1000.000000000000000 ) ;
#19390=CARTESIAN_POINT ( 'NONE',  ( 157.9999999999998295, 228.5236250225210313, 45.00000000000000000 ) ) ;
#19392=CARTESIAN_POINT ( 'NONE',  ( 158.0000000000013074, 81.06687458711267880, 45.00000000000000000 ) ) ;
#19396=ORIENTED_EDGE ( 'NONE', *, *, #23138, .T. ) ;
#19398=VERTEX_POINT ( 'NONE', #9547 ) ;
#19400=VECTOR ( 'NONE', #23906, 1000.000000000000000 ) ;
#19403=VECTOR ( 'NONE', #13731, 1000.000000000000000 ) ;
#19404=DIRECTION ( 'NONE',  ( -0.000000000000000000, -0.000000000000000000, -1.000000000000000000 ) ) ;
#19407=EDGE_CURVE ( 'NONE', #17314, #12327, #16715, .T. ) ;
#19408=VECTOR ( 'NONE', #28103, 1000.000000000000000 ) ;
#19409=VERTEX_POINT ( 'NONE', #1336 ) ;
#19414=ORIENTED_EDGE ( 'NONE', *, *, #22913, .F. ) ;
#19421=AXIS2_PLACEMENT_3D ( 'NONE', #3576, #27840, #4003 ) ;
#19423=VERTEX_POINT ( 'NONE', #16575 ) ;
#19426=DIRECTION ( 'NONE',  ( -0.000000000000000000, -0.000000000000000000, -1.000000000000000000 ) ) ;
#19428=VECTOR ( 'NONE', #13725, 1000.000000000000000 ) ;
#19429=CARTESIAN_POINT ( 'NONE',  ( 158.0000000000010232, 106.1456246621830957, 45.00000000000000000 ) ) ;
#19430=VERTEX_POINT ( 'NONE', #7808 ) ;
#19432=CARTESIAN_POINT ( 'NONE',  ( 157.4999999999996589, 273.9193126614005678, 45.00000000000000000 ) ) ;
#19435=ORIENTED_EDGE ( 'NONE', *, *, #22707, .F. ) ;
#19437=EDGE_CURVE ( 'NONE', #1905, #7826, #12415, .T. ) ;
#19439=ADVANCED_FACE ( 'NONE', ( #25467 ), #12274, .F. ) ;
#19441=ADVANCED_FACE ( 'NONE', ( #5789 ), #12698, .F. ) ;
#19444=VECTOR ( 'NONE', #21826, 1000.000000000000000 ) ;
#19446=LINE ( 'NONE', #8952, #17739 ) ;
#19449=ORIENTED_EDGE ( 'NONE', *, *, #17687, .T. ) ;
#19451=VECTOR ( 'NONE', #15209, 1000.000000000000000 ) ;
#19452=LINE ( 'NONE', #8398, #12549 ) ;
#19453=LINE ( 'NONE', #28195, #16323 ) ;
#19454=DIRECTION ( 'NONE',  ( 1.000000000000000000, 0.000000000000000000, -0.000000000000000000 ) ) ;
#19456=DIRECTION ( 'NONE',  ( 0.8916010070295719014, 0.4528218681378510801, 0.000000000000000000 ) ) ;
#19457=CARTESIAN_POINT ( 'NONE',  ( 158.0000000000014211, 68.52749954957745615, 45.00000000000000000 ) ) ;
#19459=VERTEX_POINT ( 'NONE', #18860 ) ;
#19460=DIRECTION ( 'NONE',  ( 0.000000000000000000, -1.000000000000000000, 0.000000000000000000 ) ) ;
#19463=LINE ( 'NONE', #3809, #9820 ) ;
#19467=ADVANCED_FACE ( 'NONE', ( #27608 ), #25327, .F. ) ;
#19468=LINE ( 'NONE', #18659, #131 ) ;
#19469=CARTESIAN_POINT ( 'NONE',  ( 157.4999999999994600, 213.7303124812313513, -45.00000000000000000 ) ) ;
#19470=PLANE ( 'NONE',  #12168 ) ;
#19473=AXIS2_PLACEMENT_3D ( 'NONE', #6537, #25929, #2078 ) ;
#19475=ADVANCED_FACE ( 'NONE', ( #10528 ), #19285, .F. ) ;
#19477=ORIENTED_EDGE ( 'NONE', *, *, #16431, .F. ) ;
#19478=ADVANCED_FACE ( 'NONE', ( #3623 ), #25888, .F. ) ;
#19482=ORIENTED_EDGE ( 'NONE', *, *, #10406, .T. ) ;
#19483=FACE_OUTER_BOUND ( 'NONE', #14408, .T. ) ;
#19485=ORIENTED_EDGE ( 'NONE', *, *, #21315, .F. ) ;
#19490=CARTESIAN_POINT ( 'NONE',  ( 157.4999999999998579, 83.32081209086616980, 45.00000000000000000 ) ) ;
#19491=DIRECTION ( 'NONE',  ( 0.000000000000000000, -1.000000000000000000, 0.000000000000000000 ) ) ;
#19492=DIRECTION ( 'NONE',  ( 0.4528218681383106015, 0.8916010070293384215, -0.000000000000000000 ) ) ;
#19499=ADVANCED_FACE ( 'NONE', ( #12556 ), #1614, .F. ) ;
#19506=CARTESIAN_POINT ( 'NONE',  ( 157.9999999999996305, 281.6968751876750616, -45.00000000000000000 ) ) ;
#19507=AXIS2_PLACEMENT_3D ( 'NONE', #23205, #21322, #1642 ) ;
#19514=EDGE_CURVE ( 'NONE', #21211, #8565, #12834, .T. ) ;
#19517=VECTOR ( 'NONE', #20138, 1000.000000000000000 ) ;
#19520=VERTEX_POINT ( 'NONE', #21579 ) ;
#19521=ORIENTED_EDGE ( 'NONE', *, *, #3785, .T. ) ;
#19524=DIRECTION ( 'NONE',  ( 0.4528218681374719945, 0.8916010070297644141, -0.000000000000000000 ) ) ;
#19527=VECTOR ( 'NONE', #8841, 1000.000000000000000 ) ;
#19528=LINE ( 'NONE', #17363, #6119 ) ;
#19530=PLANE ( 'NONE',  #12420 ) ;
#19532=DIRECTION ( 'NONE',  ( -0.000000000000000000, -0.000000000000000000, -1.000000000000000000 ) ) ;
#19533=VECTOR ( 'NONE', #24056, 1000.000000000000000 ) ;
#19534=CARTESIAN_POINT ( 'NONE',  ( 157.4999999999996589, 281.4429376839215138, 45.00000000000000000 ) ) ;
#19536=EDGE_CURVE ( 'NONE', #18330, #4657, #1891, .T. ) ;
#19537=PLANE ( 'NONE',  #21496 ) ;
#19538=DIRECTION ( 'NONE',  ( -0.000000000000000000, -0.000000000000000000, -1.000000000000000000 ) ) ;
#19539=DIRECTION ( 'NONE',  ( 0.4528218681373109011, -0.8916010070298462376, 0.000000000000000000 ) ) ;
#19544=SHAPE_DEFINITION_REPRESENTATION ( #17620, #10277 ) ;
#19546=ORIENTED_EDGE ( 'NONE', *, *, #23405, .F. ) ;
#19547=AXIS2_PLACEMENT_3D ( 'NONE', #5344, #17247, #28152 ) ;
#19550=EDGE_CURVE ( 'NONE', #24175, #15078, #2455, .T. ) ;
#19552=DIRECTION ( 'NONE',  ( -0.8916010070295411483, 0.4528218681379115873, 0.000000000000000000 ) ) ;
#19553=ORIENTED_EDGE ( 'NONE', *, *, #8706, .T. ) ;
#19554=AXIS2_PLACEMENT_3D ( 'NONE', #25673, #1684, #25397 ) ;
#19561=EDGE_CURVE ( 'NONE', #9422, #14501, #15275, .T. ) ;
#19562=FACE_OUTER_BOUND ( 'NONE', #19362, .T. ) ;
#19563=DIRECTION ( 'NONE',  ( -0.8916010070298353574, 0.4528218681373319954, 0.000000000000000000 ) ) ;
#19566=PLANE ( 'NONE',  #16562 ) ;
#19567=ORIENTED_EDGE ( 'NONE', *, *, #14204, .F. ) ;
#19570=AXIS2_PLACEMENT_3D ( 'NONE', #13187, #8861, #11023 ) ;
#19572=FACE_OUTER_BOUND ( 'NONE', #27366, .T. ) ;
#19573=DIRECTION ( 'NONE',  ( -0.8916010070297548662, -0.4528218681374907573, 0.000000000000000000 ) ) ;
#19578=ORIENTED_EDGE ( 'NONE', *, *, #9523, .T. ) ;
#19581=CARTESIAN_POINT ( 'NONE',  ( 157.9999999999996589, 276.1732501651540588, 45.00000000000000000 ) ) ;
#19591=ORIENTED_EDGE ( 'NONE', *, *, #19596, .F. ) ;
#19596=EDGE_CURVE ( 'NONE', #7880, #18534, #4333, .T. ) ;
#19597=EDGE_CURVE ( 'NONE', #20740, #17150, #19847, .T. ) ;
#19599=CARTESIAN_POINT ( 'NONE',  ( 157.9999999999999716, 208.9684999699701393, 45.00000000000000000 ) ) ;
#19603=CARTESIAN_POINT ( 'NONE',  ( 157.9999999999996589, 274.1732501651540588, 45.00000000000000000 ) ) ;
#19604=LINE ( 'NONE', #28343, #21975 ) ;
#19607=ORIENTED_EDGE ( 'NONE', *, *, #983, .F. ) ;
#19608=CARTESIAN_POINT ( 'NONE',  ( 158.0000000000008242, 128.2086247222394206, 45.00000000000000000 ) ) ;
#19611=CARTESIAN_POINT ( 'NONE',  ( 158.0000000000001421, 191.4133749174225443, -45.00000000000000000 ) ) ;
#19612=CARTESIAN_POINT ( 'NONE',  ( 158.0000000000015348, 58.49599951954928656, 45.00000000000000000 ) ) ;
#19617=EDGE_CURVE ( 'NONE', #24242, #12999, #26025, .T. ) ;
#19620=ORIENTED_EDGE ( 'NONE', *, *, #7862, .T. ) ;
#19622=AXIS2_PLACEMENT_3D ( 'NONE', #8365, #23446, #19134 ) ;
#19625=ORIENTED_EDGE ( 'NONE', *, *, #16246, .F. ) ;
#19629=CARTESIAN_POINT ( 'NONE',  ( 157.9999999999998579, 223.5078750075070104, 45.00000000000000000 ) ) ;
#19632=DIRECTION ( 'NONE',  ( -0.8916010070298556744, 0.4528218681372921939, 0.000000000000000000 ) ) ;
#19633=EDGE_CURVE ( 'NONE', #9022, #19307, #31, .T. ) ;
#19634=CARTESIAN_POINT ( 'NONE',  ( 158.0000000000013074, 81.06687458711267880, 45.00000000000000000 ) ) ;
#19637=ADVANCED_FACE ( 'NONE', ( #19572 ), #8790, .F. ) ;
#19643=PLANE ( 'NONE',  #10133 ) ;
#19654=ORIENTED_EDGE ( 'NONE', *, *, #3438, .F. ) ;
#19656=VERTEX_POINT ( 'NONE', #2312 ) ;
#19659=CARTESIAN_POINT ( 'NONE',  ( 158.0000000000011653, 95.60624962464788723, -45.00000000000000000 ) ) ;
#19660=ADVANCED_FACE ( 'NONE', ( #15128 ), #13258, .F. ) ;
#19664=LINE ( 'NONE', #15370, #21549 ) ;
#19665=LINE ( 'NONE', #9037, #1986 ) ;
#19667=DIRECTION ( 'NONE',  ( 0.4528218681380115629, 0.8916010070294903000, -0.000000000000000000 ) ) ;
#19671=CARTESIAN_POINT ( 'NONE',  ( 157.9999999999998010, 236.0472500450420341, 45.00000000000000000 ) ) ;
#19674=EDGE_CURVE ( 'NONE', #17424, #9868, #2604, .T. ) ;
#19676=VECTOR ( 'NONE', #20276, 1000.000000000000114 ) ;
#19679=DIRECTION ( 'NONE',  ( 0.000000000000000000, -1.000000000000000000, 0.000000000000000000 ) ) ;
#19681=ORIENTED_EDGE ( 'NONE', *, *, #4030, .T. ) ;
#19692=VERTEX_POINT ( 'NONE', #22725 ) ;
#19694=EDGE_CURVE ( 'NONE', #12920, #22238, #747, .T. ) ;
#19695=AXIS2_PLACEMENT_3D ( 'NONE', #3771, #23601, #21300 ) ;
#19697=ORIENTED_EDGE ( 'NONE', *, *, #16904, .F. ) ;
#19699=VERTEX_POINT ( 'NONE', #16125 ) ;
#19704=EDGE_CURVE ( 'NONE', #21239, #991, #7213, .T. ) ;
#19709=ORIENTED_EDGE ( 'NONE', *, *, #20357, .T. ) ;
#19714=ORIENTED_EDGE ( 'NONE', *, *, #10651, .F. ) ;
#19719=CARTESIAN_POINT ( 'NONE',  ( 157.9999999999998863, 216.4921249924925348, 45.00000000000000000 ) ) ;
#19722=ORIENTED_EDGE ( 'NONE', *, *, #24148, .T. ) ;
#19739=PLANE ( 'NONE',  #6503 ) ;
#19740=DIRECTION ( 'NONE',  ( 0.8916010070293682865, 0.4528218681382519262, 0.000000000000000000 ) ) ;
#19741=LINE ( 'NONE', #26343, #19428 ) ;
#19742=VERTEX_POINT ( 'NONE', #15986 ) ;
#19745=DIRECTION ( 'NONE',  ( 0.000000000000000000, -1.000000000000000000, 0.000000000000000000 ) ) ;
#19750=ORIENTED_EDGE ( 'NONE', *, *, #24823, .T. ) ;
#19751=VECTOR ( 'NONE', #2775, 1000.000000000000227 ) ;
#19752=CARTESIAN_POINT ( 'NONE',  ( 158.0000000000002274, 185.8897498949014278, 45.00000000000000000 ) ) ;
#19757=EDGE_LOOP ( 'NONE', ( #25751, #15204, #21242, #25945 ) ) ;
#19758=ADVANCED_FACE ( 'NONE', ( #5467 ), #11817, .F. ) ;
#19759=DIRECTION ( 'NONE',  ( 0.4528218681371909971, -0.8916010070299070778, 0.000000000000000000 ) ) ;
#19761=ADVANCED_FACE ( 'NONE', ( #24875 ), #20417, .F. ) ;
#19768=DIRECTION ( 'NONE',  ( -0.000000000000000000, 0.000000000000000000, -1.000000000000000000 ) ) ;
#19769=DIRECTION ( 'NONE',  ( 0.8916010070296429557, -0.4528218681377111920, 0.000000000000000000 ) ) ;
#19770=FACE_OUTER_BOUND ( 'NONE', #9975, .T. ) ;
#19771=VECTOR ( 'NONE', #4040, 999.9999999999998863 ) ;
#19776=DIRECTION ( 'NONE',  ( -0.000000000000000000, -0.000000000000000000, -1.000000000000000000 ) ) ;
#19778=DIRECTION ( 'NONE',  ( 1.000000000000000000, 0.000000000000000000, -0.000000000000000000 ) ) ;
#19779=VECTOR ( 'NONE', #22404, 1000.000000000000000 ) ;
#19781=DIRECTION ( 'NONE',  ( 0.4528218681383305855, -0.8916010070293283185, 0.000000000000000000 ) ) ;
#19785=CARTESIAN_POINT ( 'NONE',  ( 157.4999999999994600, 216.2381874887387880, 45.00000000000000000 ) ) ;
#19792=EDGE_CURVE ( 'NONE', #8705, #5655, #22583, .T. ) ;
#19793=VECTOR ( 'NONE', #23074, 1000.000000000000000 ) ;
#19794=EDGE_CURVE ( 'NONE', #23572, #7620, #25016, .T. ) ;
#19797=CARTESIAN_POINT ( 'NONE',  ( 158.0000000000011653, 95.60624962464788723, -45.00000000000000000 ) ) ;
#19805=CARTESIAN_POINT ( 'NONE',  ( 157.4999999999998579, 55.73418700828869277, 45.00000000000000000 ) ) ;
#19806=PLANE ( 'NONE',  #19989 ) ;
#19811=AXIS2_PLACEMENT_3D ( 'NONE', #5926, #23453, #14700 ) ;
#19815=CARTESIAN_POINT ( 'NONE',  ( 158.0000000000014211, 70.52749954957745615, -45.00000000000000000 ) ) ;
#19818=ORIENTED_EDGE ( 'NONE', *, *, #10209, .T. ) ;
#19827=EDGE_CURVE ( 'NONE', #2081, #6570, #14954, .T. ) ;
#19830=EDGE_CURVE ( 'NONE', #13130, #26005, #1436, .T. ) ;
#19831=ORIENTED_EDGE ( 'NONE', *, *, #25718, .T. ) ;
#19835=VECTOR ( 'NONE', #19108, 1000.000000000000000 ) ;
#19847=LINE ( 'NONE', #4190, #15257 ) ;
#19849=ORIENTED_EDGE ( 'NONE', *, *, #3116, .F. ) ;
#19851=CARTESIAN_POINT ( 'NONE',  ( 157.4999999999998579, 178.6200623761337738, 45.00000000000000000 ) ) ;
#19856=ORIENTED_EDGE ( 'NONE', *, *, #11305, .T. ) ;
#19859=ORIENTED_EDGE ( 'NONE', *, *, #20508, .T. ) ;
#19860=CARTESIAN_POINT ( 'NONE',  ( 158.0000000000010800, 101.1298746471690038, 45.00000000000000000 ) ) ;
#19862=ORIENTED_EDGE ( 'NONE', *, *, #25795, .F. ) ;
#19865=EDGE_CURVE ( 'NONE', #25224, #22406, #25290, .T. ) ;
#19868=ORIENTED_EDGE ( 'NONE', *, *, #25013, .F. ) ;
#19871=VECTOR ( 'NONE', #13128, 1000.000000000000114 ) ;
#19872=LINE ( 'NONE', #11265, #4834 ) ;
#19874=DIRECTION ( 'NONE',  ( 0.000000000000000000, -1.000000000000000000, 0.000000000000000000 ) ) ;
#19876=CARTESIAN_POINT ( 'NONE',  ( 158.0000000000013358, 80.55899957960563995, -45.00000000000000000 ) ) ;
#19877=EDGE_CURVE ( 'NONE', #17145, #14062, #23418, .T. ) ;
#19878=CARTESIAN_POINT ( 'NONE',  ( 158.0000000000015632, 57.98812451204224061, 45.00000000000000000 ) ) ;
#19883=CARTESIAN_POINT ( 'NONE',  ( 157.9999999999997726, 244.0787500750700474, 45.00000000000000000 ) ) ;
#19885=DIRECTION ( 'NONE',  ( -0.8916010070293383105, -0.4528218681383106015, 0.000000000000000000 ) ) ;
#19887=DIRECTION ( 'NONE',  ( 1.000000000000000000, 0.000000000000000000, -0.000000000000000000 ) ) ;
#19889=EDGE_CURVE ( 'NONE', #5660, #15498, #23282, .T. ) ;
#19890=DIRECTION ( 'NONE',  ( 0.4528218681382319422, 0.8916010070293783896, -0.000000000000000000 ) ) ;
#19892=CARTESIAN_POINT ( 'NONE',  ( 158.0000000000014211, 70.52749954957745615, -45.00000000000000000 ) ) ;
#19893=VERTEX_POINT ( 'NONE', #25709 ) ;
#19895=VERTEX_POINT ( 'NONE', #20840 ) ;
#19897=DIRECTION ( 'NONE',  ( -0.000000000000000000, -0.000000000000000000, -1.000000000000000000 ) ) ;
#19898=ORIENTED_EDGE ( 'NONE', *, *, #27186, .F. ) ;
#19899=DIRECTION ( 'NONE',  ( -0.000000000000000000, 0.000000000000000000, -1.000000000000000000 ) ) ;
#19900=EDGE_LOOP ( 'NONE', ( #10048, #21455, #897, #12643 ) ) ;
#19901=VECTOR ( 'NONE', #5543, 1000.000000000000000 ) ;
#19903=EDGE_CURVE ( 'NONE', #9517, #1905, #3727, .T. ) ;
#19904=DIRECTION ( 'NONE',  ( 0.8916010070296834789, -0.4528218681376312005, 0.000000000000000000 ) ) ;
#19906=ORIENTED_EDGE ( 'NONE', *, *, #1180, .F. ) ;
#19907=ORIENTED_EDGE ( 'NONE', *, *, #15561, .T. ) ;
#19912=VECTOR ( 'NONE', #6726, 1000.000000000000000 ) ;
#19920=CARTESIAN_POINT ( 'NONE',  ( 158.0000000000015064, 61.00387452705632541, 45.00000000000000000 ) ) ;
#19921=CARTESIAN_POINT ( 'NONE',  ( 158.0000000000017337, 40.94087446699997912, -45.00000000000000000 ) ) ;
#19924=CARTESIAN_POINT ( 'NONE',  ( 157.9999999999997726, 243.5708750675630370, 45.00000000000000000 ) ) ;
#19930=ORIENTED_EDGE ( 'NONE', *, *, #12419, .F. ) ;
#19931=FACE_OUTER_BOUND ( 'NONE', #6718, .T. ) ;
#19932=VERTEX_POINT ( 'NONE', #10348 ) ;
#19933=DIRECTION ( 'NONE',  ( 0.8916010070298360235, 0.4528218681373308296, 0.000000000000000000 ) ) ;
#19934=ORIENTED_EDGE ( 'NONE', *, *, #16315, .F. ) ;
#19938=EDGE_CURVE ( 'NONE', #7676, #2950, #16678, .T. ) ;
#19939=EDGE_LOOP ( 'NONE', ( #27972, #6409, #3510, #16797 ) ) ;
#19942=VERTEX_POINT ( 'NONE', #5753 ) ;
#19943=LINE ( 'NONE', #15506, #21900 ) ;
#19944=DIRECTION ( 'NONE',  ( -0.000000000000000000, -0.000000000000000000, -1.000000000000000000 ) ) ;
#19952=LINE ( 'NONE', #26409, #17189 ) ;
#19955=AXIS2_PLACEMENT_3D ( 'NONE', #25009, #5325, #14101 ) ;
#19956=EDGE_CURVE ( 'NONE', #14934, #20505, #3305, .T. ) ;
#19957=EDGE_CURVE ( 'NONE', #4647, #12815, #17801, .T. ) ;
#19960=CARTESIAN_POINT ( 'NONE',  ( 157.4999999999998579, 100.8759371434154701, 45.00000000000000000 ) ) ;
#19961=VECTOR ( 'NONE', #16445, 1000.000000000000114 ) ;
#19965=DIRECTION ( 'NONE',  ( -0.000000000000000000, -0.000000000000000000, -1.000000000000000000 ) ) ;
#19967=ORIENTED_EDGE ( 'NONE', *, *, #28176, .F. ) ;
#19970=VERTEX_POINT ( 'NONE', #15092 ) ;
#19972=DIRECTION ( 'NONE',  ( -0.8916010070293584056, -0.4528218681382712996, 0.000000000000000000 ) ) ;
#19976=AXIS2_PLACEMENT_3D ( 'NONE', #1246, #19191, #16897 ) ;
#19977=PLANE ( 'NONE',  #1253 ) ;
#19979=ORIENTED_EDGE ( 'NONE', *, *, #16587, .T. ) ;
#19983=CARTESIAN_POINT ( 'NONE',  ( 157.9999999999999432, 213.4763749774776045, -45.00000000000000000 ) ) ;
#19987=DIRECTION ( 'NONE',  ( 0.8916010070293384215, 0.4528218681383106015, 0.000000000000000000 ) ) ;
#19989=AXIS2_PLACEMENT_3D ( 'NONE', #2559, #26407, #22107 ) ;
#19990=CARTESIAN_POINT ( 'NONE',  ( 158.0000000000003411, 173.8582498648732440, -45.00000000000000000 ) ) ;
#19992=CARTESIAN_POINT ( 'NONE',  ( 158.0000000000009948, 108.6534996696901345, -45.00000000000000000 ) ) ;
#19993=EDGE_LOOP ( 'NONE', ( #11836, #26042, #21547, #17706 ) ) ;
#20000=VERTEX_POINT ( 'NONE', #13367 ) ;
#20001=CARTESIAN_POINT ( 'NONE',  ( 157.4999999999998579, 181.1279373836408411, 45.00000000000000000 ) ) ;
#20006=CARTESIAN_POINT ( 'NONE',  ( 157.4999999999998579, 138.4940622560211239, 45.00000000000000000 ) ) ;
#20007=ORIENTED_EDGE ( 'NONE', *, *, #23454, .F. ) ;
#20011=ADVANCED_FACE ( 'NONE', ( #24272 ), #10634, .F. ) ;
#20013=FACE_OUTER_BOUND ( 'NONE', #24195, .T. ) ;
#20017=DIRECTION ( 'NONE',  ( 0.4528218681378510801, -0.8916010070295719014, 0.000000000000000000 ) ) ;
#20018=DIRECTION ( 'NONE',  ( 0.8916010070293283185, 0.4528218681383305855, 0.000000000000000000 ) ) ;
#20019=ORIENTED_EDGE ( 'NONE', *, *, #12091, .F. ) ;
#20021=ADVANCED_FACE ( 'NONE', ( #6313 ), #8480, .F. ) ;
#20025=ORIENTED_EDGE ( 'NONE', *, *, #12034, .T. ) ;
#20026=DIRECTION ( 'NONE',  ( 0.4528218681372909171, -0.8916010070298563406, 0.000000000000000000 ) ) ;
#20027=VERTEX_POINT ( 'NONE', #21971 ) ;
#20032=VERTEX_POINT ( 'NONE', #28140 ) ;
#20034=VERTEX_POINT ( 'NONE', #21839 ) ;
#20035=AXIS2_PLACEMENT_3D ( 'NONE', #18601, #27351, #7267 ) ;
#20036=DIRECTION ( 'NONE',  ( 0.000000000000000000, -1.000000000000000000, 0.000000000000000000 ) ) ;
#20038=DIRECTION ( 'NONE',  ( -0.8916010070293711731, 0.4528218681382463751, 0.000000000000000000 ) ) ;
#20043=ORIENTED_EDGE ( 'NONE', *, *, #3085, .F. ) ;
#20047=EDGE_CURVE ( 'NONE', #27897, #7159, #17515, .T. ) ;
#20052=DIRECTION ( 'NONE',  ( 0.000000000000000000, -1.000000000000000000, 0.000000000000000000 ) ) ;
#20055=CARTESIAN_POINT ( 'NONE',  ( 158.0000000000008811, 123.1928747072253572, -45.00000000000000000 ) ) ;
#20059=LINE ( 'NONE', #13762, #11644 ) ;
#20060=ORIENTED_EDGE ( 'NONE', *, *, #18434, .T. ) ;
#20061=CARTESIAN_POINT ( 'NONE',  ( 157.4999999999998010, 233.7933125412885147, 45.00000000000000000 ) ) ;
#20065=LINE ( 'NONE', #22084, #27277 ) ;
#20067=ORIENTED_EDGE ( 'NONE', *, *, #26151, .T. ) ;
#20068=AXIS2_PLACEMENT_3D ( 'NONE', #5642, #21002, #3901 ) ;
#20070=ORIENTED_EDGE ( 'NONE', *, *, #15206, .T. ) ;
#20071=VERTEX_POINT ( 'NONE', #8624 ) ;
#20072=AXIS2_PLACEMENT_3D ( 'NONE', #22845, #10904, #6587 ) ;
#20073=EDGE_CURVE ( 'NONE', #23817, #11039, #143, .T. ) ;
#20075=VECTOR ( 'NONE', #17188, 1000.000000000000000 ) ;
#20076=ADVANCED_FACE ( 'NONE', ( #26137 ), #6461, .F. ) ;
#20078=ORIENTED_EDGE ( 'NONE', *, *, #26079, .F. ) ;
#20081=LINE ( 'NONE', #2407, #22837 ) ;
#20083=CARTESIAN_POINT ( 'NONE',  ( 157.4999999999998579, 43.19481197075347723, -45.00000000000000000 ) ) ;
#20084=EDGE_CURVE ( 'NONE', #13314, #9427, #2283, .T. ) ;
#20085=PRODUCT_DEFINITION_CONTEXT ( 'detailed design', #8551, 'design' ) ;
#20086=LINE ( 'NONE', #24835, #28142 ) ;
#20088=VECTOR ( 'NONE', #21965, 1000.000000000000000 ) ;
#20089=DIRECTION ( 'NONE',  ( -0.000000000000000000, -0.000000000000000000, -1.000000000000000000 ) ) ;
#20093=LINE ( 'NONE', #15378, #21787 ) ;
#20094=CARTESIAN_POINT ( 'NONE',  ( 157.4999999999998010, 233.7933125412885147, 45.00000000000000000 ) ) ;
#20099=DIRECTION ( 'NONE',  ( 0.8916010070295817824, -0.4528218681378317623, 0.000000000000000000 ) ) ;
#20101=ORIENTED_EDGE ( 'NONE', *, *, #25586, .F. ) ;
#20102=ORIENTED_EDGE ( 'NONE', *, *, #11520, .T. ) ;
#20103=CARTESIAN_POINT ( 'NONE',  ( 158.0000000000015632, 57.98812451204224061, 45.00000000000000000 ) ) ;
#20105=CARTESIAN_POINT ( 'NONE',  ( 157.9999999999998295, 226.0157500150140208, -45.00000000000000000 ) ) ;
#20106=LINE ( 'NONE', #21843, #1175 ) ;
#20110=ORIENTED_EDGE ( 'NONE', *, *, #26768, .T. ) ;
#20112=DIRECTION ( 'NONE',  ( -0.8916010070293682865, -0.4528218681382519262, 0.000000000000000000 ) ) ;
#20115=ORIENTED_EDGE ( 'NONE', *, *, #14390, .T. ) ;
#20116=ORIENTED_EDGE ( 'NONE', *, *, #18687, .F. ) ;
#20117=DIRECTION ( 'NONE',  ( 0.4528218681372122578, 0.8916010070298964196, -0.000000000000000000 ) ) ;
#20118=EDGE_CURVE ( 'NONE', #905, #3644, #24847, .T. ) ;
#20122=CARTESIAN_POINT ( 'NONE',  ( 158.0000000000012790, 85.57474959461971764, 45.00000000000000000 ) ) ;
#20123=VECTOR ( 'NONE', #4898, 1000.000000000000000 ) ;
#20130=LINE ( 'NONE', #19990, #12461 ) ;
#20133=ORIENTED_EDGE ( 'NONE', *, *, #9537, .F. ) ;
#20136=EDGE_CURVE ( 'NONE', #6606, #23450, #20245, .T. ) ;
#20138=DIRECTION ( 'NONE',  ( -0.000000000000000000, -0.000000000000000000, -1.000000000000000000 ) ) ;
#20142=DIRECTION ( 'NONE',  ( 0.000000000000000000, -1.000000000000000000, 0.000000000000000000 ) ) ;
#20143=VECTOR ( 'NONE', #13582, 999.9999999999998863 ) ;
#20148=ORIENTED_EDGE ( 'NONE', *, *, #25566, .T. ) ;
#20149=EDGE_CURVE ( 'NONE', #19942, #9066, #11792, .T. ) ;
#20151=EDGE_CURVE ( 'NONE', #10576, #19932, #13657, .T. ) ;
#20153=PLANE ( 'NONE',  #27674 ) ;
#20156=PLANE ( 'NONE',  #4557 ) ;
#20160=CARTESIAN_POINT ( 'NONE',  ( 157.4999999999998579, 100.8759371434154701, 45.00000000000000000 ) ) ;
#20167=DIRECTION ( 'NONE',  ( 0.8916010070293384215, 0.4528218681383106015, 0.000000000000000000 ) ) ;
#20168=DIRECTION ( 'NONE',  ( 0.8916010070293384215, 0.4528218681383106015, 0.000000000000000000 ) ) ;
#20181=ORIENTED_EDGE ( 'NONE', *, *, #34, .F. ) ;
#20186=DIRECTION ( 'NONE',  ( 0.4528218681379503896, -0.8916010070295214973, 0.000000000000000000 ) ) ;
#20187=ORIENTED_EDGE ( 'NONE', *, *, #5112, .F. ) ;
#20193=ORIENTED_EDGE ( 'NONE', *, *, #18053, .T. ) ;
#20196=VECTOR ( 'NONE', #27616, 1000.000000000000114 ) ;
#20198=CARTESIAN_POINT ( 'NONE',  ( 158.0000000000000568, 201.4448749474510407, -45.00000000000000000 ) ) ;
#20199=CARTESIAN_POINT ( 'NONE',  ( 158.0000000000008242, 126.2086247222394206, 45.00000000000000000 ) ) ;
#20202=FACE_OUTER_BOUND ( 'NONE', #15749, .T. ) ;
#20204=DIRECTION ( 'NONE',  ( 0.000000000000000000, -1.000000000000000000, 0.000000000000000000 ) ) ;
#20205=DIRECTION ( 'NONE',  ( 0.8916010070293384215, 0.4528218681383106015, 0.000000000000000000 ) ) ;
#20211=DIRECTION ( 'NONE',  ( 0.8916010070295820045, -0.4528218681378310406, 0.000000000000000000 ) ) ;
#20214=ORIENTED_EDGE ( 'NONE', *, *, #18354, .F. ) ;
#20216=EDGE_CURVE ( 'NONE', #20740, #9697, #13951, .T. ) ;
#20217=PLANE ( 'NONE',  #11604 ) ;
#20221=ORIENTED_EDGE ( 'NONE', *, *, #27086, .F. ) ;
#20225=CARTESIAN_POINT ( 'NONE',  ( 158.0000000000004832, 163.3188748273380213, 45.00000000000000000 ) ) ;
#20230=LINE ( 'NONE', #4854, #18546 ) ;
#20236=DIRECTION ( 'NONE',  ( 0.8916010070298759915, -0.4528218681372521703, 0.000000000000000000 ) ) ;
#20237=DIRECTION ( 'NONE',  ( -0.8916010070294801970, 0.4528218681380314914, 0.000000000000000000 ) ) ;
#20245=LINE ( 'NONE', #2861, #2880 ) ;
#20246=ORIENTED_EDGE ( 'NONE', *, *, #17154, .T. ) ;
#20247=ORIENTED_EDGE ( 'NONE', *, *, #12288, .F. ) ;
#20248=CARTESIAN_POINT ( 'NONE',  ( 158.0000000000004547, 163.8267498348450886, 45.00000000000000000 ) ) ;
#20250=FACE_OUTER_BOUND ( 'NONE', #14792, .T. ) ;
#20259=ORIENTED_EDGE ( 'NONE', *, *, #18144, .T. ) ;
#20261=FACE_OUTER_BOUND ( 'NONE', #24855, .T. ) ;
#20265=ORIENTED_EDGE ( 'NONE', *, *, #16188, .T. ) ;
#20266=CARTESIAN_POINT ( 'NONE',  ( 158.0000000000013358, 80.55899957960563995, -45.00000000000000000 ) ) ;
#20267=LINE ( 'NONE', #22715, #17124 ) ;
#20268=VECTOR ( 'NONE', #26473, 1000.000000000000000 ) ;
#20269=DIRECTION ( 'NONE',  ( 0.4528218681372509491, -0.8916010070298766577, 0.000000000000000000 ) ) ;
#20271=CARTESIAN_POINT ( 'NONE',  ( 158.0000000000015632, 57.98812451204224061, -45.00000000000000000 ) ) ;
#20276=DIRECTION ( 'NONE',  ( 0.8916010070295410372, -0.4528218681379115873, 0.000000000000000000 ) ) ;
#20281=EDGE_CURVE ( 'NONE', #26421, #23616, #19468, .T. ) ;
#20288=EDGE_LOOP ( 'NONE', ( #21015, #19967, #20007, #10547 ) ) ;
#20300=CARTESIAN_POINT ( 'NONE',  ( 157.9999999999998010, 231.5393750375350237, 45.00000000000000000 ) ) ;
#20304=VECTOR ( 'NONE', #22681, 1000.000000000000000 ) ;
#20305=CARTESIAN_POINT ( 'NONE',  ( 158.0000000000004263, 168.3346248423521274, 45.00000000000000000 ) ) ;
#20312=CARTESIAN_POINT ( 'NONE',  ( 158.0000000000003126, 178.3661248723802828, 45.00000000000000000 ) ) ;
#20316=VECTOR ( 'NONE', #20036, 1000.000000000000000 ) ;
#20318=ORIENTED_EDGE ( 'NONE', *, *, #27526, .F. ) ;
#20330=VERTEX_POINT ( 'NONE', #6250 ) ;
#20332=ORIENTED_EDGE ( 'NONE', *, *, #9061, .T. ) ;
#20336=ORIENTED_EDGE ( 'NONE', *, *, #3021, .F. ) ;
#20337=VERTEX_POINT ( 'NONE', #12737 ) ;
#20341=CARTESIAN_POINT ( 'NONE',  ( 157.4999999999996874, 266.3956876388795649, -45.00000000000000000 ) ) ;
#20351=LINE ( 'NONE', #19921, #8876 ) ;
#20353=VECTOR ( 'NONE', #23698, 1000.000000000000227 ) ;
#20354=PLANE ( 'NONE',  #12890 ) ;
#20355=EDGE_CURVE ( 'NONE', #14898, #14664, #10568, .T. ) ;
#20357=EDGE_CURVE ( 'NONE', #21673, #10576, #10854, .T. ) ;
#20362=ORIENTED_EDGE ( 'NONE', *, *, #19597, .T. ) ;
#20367=ORIENTED_EDGE ( 'NONE', *, *, #735, .T. ) ;
#20368=EDGE_LOOP ( 'NONE', ( #13369, #21637, #21050, #646 ) ) ;
#20369=ORIENTED_EDGE ( 'NONE', *, *, #25821, .T. ) ;
#20372=CARTESIAN_POINT ( 'NONE',  ( 157.4999999999998579, 196.1751874286831026, 45.00000000000000000 ) ) ;
#20375=EDGE_CURVE ( 'NONE', #21445, #25157, #7745, .T. ) ;
#20376=CARTESIAN_POINT ( 'NONE',  ( 157.4999999999998010, 233.7933125412885147, 45.00000000000000000 ) ) ;
#20383=LINE ( 'NONE', #17406, #17006 ) ;
#20384=LINE ( 'NONE', #9334, #14604 ) ;
#20387=EDGE_CURVE ( 'NONE', #4329, #1247, #16513, .T. ) ;
#20392=ORIENTED_EDGE ( 'NONE', *, *, #16147, .T. ) ;
#20393=AXIS2_PLACEMENT_3D ( 'NONE', #10661, #17122, #28165 ) ;
#20396=DIRECTION ( 'NONE',  ( -0.000000000000000000, -0.000000000000000000, -1.000000000000000000 ) ) ;
#20397=VERTEX_POINT ( 'NONE', #20953 ) ;
#20398=ORIENTED_EDGE ( 'NONE', *, *, #14170, .F. ) ;
#20399=CARTESIAN_POINT ( 'NONE',  ( 158.0000000000009379, 116.1771246922112653, 45.00000000000000000 ) ) ;
#20402=ORIENTED_EDGE ( 'NONE', *, *, #1365, .T. ) ;
#20403=PLANE ( 'NONE',  #23436 ) ;
#20404=EDGE_CURVE ( 'NONE', #1347, #26566, #12069, .T. ) ;
#20405=DIRECTION ( 'NONE',  ( 1.000000000000000000, 0.000000000000000000, -0.000000000000000000 ) ) ;
#20406=LINE ( 'NONE', #736, #15123 ) ;
#20408=VECTOR ( 'NONE', #7350, 1000.000000000000000 ) ;
#20409=LINE ( 'NONE', #5182, #14867 ) ;
#20412=AXIS2_PLACEMENT_3D ( 'NONE', #28179, #14995, #8524 ) ;
#20415=LINE ( 'NONE', #13976, #24728 ) ;
#20416=DIRECTION ( 'NONE',  ( -0.000000000000000000, -0.000000000000000000, -1.000000000000000000 ) ) ;
#20417=PLANE ( 'NONE',  #17996 ) ;
#20421=ADVANCED_FACE ( 'NONE', ( #16377 ), #17307, .F. ) ;
#20422=EDGE_CURVE ( 'NONE', #14865, #7880, #17027, .T. ) ;
#20425=ORIENTED_EDGE ( 'NONE', *, *, #13350, .T. ) ;
#20428=EDGE_LOOP ( 'NONE', ( #7340, #11143, #20116, #3417 ) ) ;
#20431=CARTESIAN_POINT ( 'NONE',  ( 158.0000000000017053, 43.44874947450702507, -45.00000000000000000 ) ) ;
#20433=ORIENTED_EDGE ( 'NONE', *, *, #18284, .T. ) ;
#20443=DIRECTION ( 'NONE',  ( 1.000000000000000000, 0.000000000000000000, -0.000000000000000000 ) ) ;
#20445=CARTESIAN_POINT ( 'NONE',  ( 158.0000000000005116, 158.8109998198309825, -45.00000000000000000 ) ) ;
#20447=EDGE_CURVE ( 'NONE', #15242, #20027, #17879, .T. ) ;
#20451=PLANE ( 'NONE',  #20584 ) ;
#20453=CARTESIAN_POINT ( 'NONE',  ( 158.0000000000007390, 135.7322497447605656, 45.00000000000000000 ) ) ;
#20454=LINE ( 'NONE', #18017, #26757 ) ;
#20457=VECTOR ( 'NONE', #25590, 1000.000000000000000 ) ;
#20459=DIRECTION ( 'NONE',  ( 1.000000000000000000, 0.000000000000000000, -0.000000000000000000 ) ) ;
#20460=CARTESIAN_POINT ( 'NONE',  ( 157.4999999999998579, 65.76568703831686946, -45.00000000000000000 ) ) ;
#20463=ORIENTED_EDGE ( 'NONE', *, *, #25620, .F. ) ;
#20465=CARTESIAN_POINT ( 'NONE',  ( 157.4999999999998579, 130.9704372334999789, 45.00000000000000000 ) ) ;
#20470=ORIENTED_EDGE ( 'NONE', *, *, #16393, .T. ) ;
#20472=DIRECTION ( 'NONE',  ( 0.4528218681382463751, 0.8916010070293711731, -0.000000000000000000 ) ) ;
#20474=VECTOR ( 'NONE', #12531, 1000.000000000000000 ) ;
#20480=ORIENTED_EDGE ( 'NONE', *, *, #20675, .F. ) ;
#20484=CARTESIAN_POINT ( 'NONE',  ( 157.9999999999997158, 258.6181251126050711, -45.00000000000000000 ) ) ;
#20486=CARTESIAN_POINT ( 'NONE',  ( 157.9999999999997726, 246.0787500750700474, 45.00000000000000000 ) ) ;
#20487=DIRECTION ( 'NONE',  ( -0.000000000000000000, -0.000000000000000000, -1.000000000000000000 ) ) ;
#20489=LINE ( 'NONE', #814, #25983 ) ;
#20492=CARTESIAN_POINT ( 'NONE',  ( 157.4999999999995168, 208.7145624662163925, 45.00000000000000000 ) ) ;
#20495=ORIENTED_EDGE ( 'NONE', *, *, #5523, .T. ) ;
#20496=EDGE_CURVE ( 'NONE', #23733, #24388, #15455, .T. ) ;
#20499=LINE ( 'NONE', #18355, #19346 ) ;
#20500=ORIENTED_EDGE ( 'NONE', *, *, #7862, .F. ) ;
#20502=ORIENTED_EDGE ( 'NONE', *, *, #20404, .T. ) ;
#20503=EDGE_CURVE ( 'NONE', #9458, #11526, #26786, .T. ) ;
#20504=CARTESIAN_POINT ( 'NONE',  ( 157.4999999999998295, 40.68693696324645970, 45.00000000000000000 ) ) ;
#20505=VERTEX_POINT ( 'NONE', #17448 ) ;
#20506=VERTEX_POINT ( 'NONE', #24339 ) ;
#20508=EDGE_CURVE ( 'NONE', #15103, #8705, #8695, .T. ) ;
#20510=DIRECTION ( 'NONE',  ( 0.8916010070297439860, -0.4528218681375119070, 0.000000000000000000 ) ) ;
#20513=CARTESIAN_POINT ( 'NONE',  ( 157.4999999999998579, 181.1279373836408411, 45.00000000000000000 ) ) ;
#20514=ADVANCED_FACE ( 'NONE', ( #15742 ), #2352, .F. ) ;
#20515=AXIS2_PLACEMENT_3D ( 'NONE', #3399, #14480, #16773 ) ;
#20524=DIRECTION ( 'NONE',  ( 0.8916010070299672519, -0.4528218681370723142, 0.000000000000000000 ) ) ;
#20525=FACE_OUTER_BOUND ( 'NONE', #23198, .T. ) ;
#20531=ORIENTED_EDGE ( 'NONE', *, *, #15962, .F. ) ;
#20534=DIRECTION ( 'NONE',  ( 0.000000000000000000, -1.000000000000000000, 0.000000000000000000 ) ) ;
#20539=DIRECTION ( 'NONE',  ( -0.000000000000000000, 0.000000000000000000, -1.000000000000000000 ) ) ;
#20544=DIRECTION ( 'NONE',  ( 0.8916010070293383105, -0.4528218681383106015, 0.000000000000000000 ) ) ;
#20547=DIRECTION ( 'NONE',  ( 0.4528218681370723142, 0.8916010070299673629, -0.000000000000000000 ) ) ;
#20555=LINE ( 'NONE', #27711, #20700 ) ;
#20557=DIRECTION ( 'NONE',  ( -0.000000000000000000, 0.000000000000000000, -1.000000000000000000 ) ) ;
#20559=DIRECTION ( 'NONE',  ( -0.8916010070297749612, -0.4528218681374510668, 0.000000000000000000 ) ) ;
#20560=VECTOR ( 'NONE', #11611, 1000.000000000000114 ) ;
#20562=AXIS2_PLACEMENT_3D ( 'NONE', #5785, #25596, #27884 ) ;
#20563=LINE ( 'NONE', #1025, #13577 ) ;
#20567=EDGE_CURVE ( 'NONE', #15393, #12113, #360, .T. ) ;
#20573=CARTESIAN_POINT ( 'NONE',  ( 157.4999999999998579, 103.3838121509225090, 45.00000000000000000 ) ) ;
#20576=CARTESIAN_POINT ( 'NONE',  ( 157.4999999999998579, 135.9861872485140850, 45.00000000000000000 ) ) ;
#20582=EDGE_CURVE ( 'NONE', #10648, #27544, #24634, .T. ) ;
#20584=AXIS2_PLACEMENT_3D ( 'NONE', #24905, #5219, #9541 ) ;
#20585=DIRECTION ( 'NONE',  ( 0.8916010070293584056, -0.4528218681382712996, 0.000000000000000000 ) ) ;
#20586=DIRECTION ( 'NONE',  ( -0.000000000000000000, -0.000000000000000000, -1.000000000000000000 ) ) ;
#20588=DIRECTION ( 'NONE',  ( 0.000000000000000000, -1.000000000000000000, 0.000000000000000000 ) ) ;
#20595=CARTESIAN_POINT ( 'NONE',  ( 158.0000000000012506, 86.08262460212675649, -45.00000000000000000 ) ) ;
#20599=ORIENTED_EDGE ( 'NONE', *, *, #16628, .F. ) ;
#20601=VECTOR ( 'NONE', #23319, 1000.000000000000000 ) ;
#20602=CARTESIAN_POINT ( 'NONE',  ( 157.9999999999996589, 279.1890001801680796, -45.00000000000000000 ) ) ;
#20605=ORIENTED_EDGE ( 'NONE', *, *, #24879, .T. ) ;
#20615=CARTESIAN_POINT ( 'NONE',  ( 157.4999999999998579, 166.0806873385985796, 45.00000000000000000 ) ) ;
#20616=ORIENTED_EDGE ( 'NONE', *, *, #10956, .T. ) ;
#20618=ORIENTED_EDGE ( 'NONE', *, *, #13101, .F. ) ;
#20619=DIRECTION ( 'NONE',  ( -0.000000000000000000, -0.000000000000000000, -1.000000000000000000 ) ) ;
#20622=DIRECTION ( 'NONE',  ( 0.000000000000000000, -1.000000000000000000, 0.000000000000000000 ) ) ;
#20626=DIRECTION ( 'NONE',  ( -0.8916010070293409751, -0.4528218681383056610, 0.000000000000000000 ) ) ;
#20627=VECTOR ( 'NONE', #5828, 1000.000000000000000 ) ;
#20629=CARTESIAN_POINT ( 'NONE',  ( 158.0000000000004832, 163.3188748273380213, -45.00000000000000000 ) ) ;
#20631=CARTESIAN_POINT ( 'NONE',  ( 157.9999999999996589, 274.1732501651540588, 45.00000000000000000 ) ) ;
#20633=DIRECTION ( 'NONE',  ( 0.000000000000000000, -1.000000000000000000, 0.000000000000000000 ) ) ;
#20635=ORIENTED_EDGE ( 'NONE', *, *, #25702, .F. ) ;
#20639=DIRECTION ( 'NONE',  ( 0.4528218681380302146, -0.8916010070294808632, 0.000000000000000000 ) ) ;
#20640=ORIENTED_EDGE ( 'NONE', *, *, #25752, .T. ) ;
#20641=EDGE_CURVE ( 'NONE', #583, #20671, #5657, .T. ) ;
#20651=EDGE_LOOP ( 'NONE', ( #12209, #20680, #21172, #4285 ) ) ;
#20664=DIRECTION ( 'NONE',  ( -0.000000000000000000, -0.000000000000000000, -1.000000000000000000 ) ) ;
#20665=VECTOR ( 'NONE', #18029, 1000.000000000000000 ) ;
#20671=VERTEX_POINT ( 'NONE', #20602 ) ;
#20672=EDGE_CURVE ( 'NONE', #15498, #16458, #7541, .T. ) ;
#20673=EDGE_CURVE ( 'NONE', #19152, #7888, #26929, .T. ) ;
#20674=CARTESIAN_POINT ( 'NONE',  ( 157.9999999999998863, 216.4921249924925348, 45.00000000000000000 ) ) ;
#20675=EDGE_CURVE ( 'NONE', #12678, #21329, #25191, .T. ) ;
#20677=ORIENTED_EDGE ( 'NONE', *, *, #12709, .F. ) ;
#20679=ORIENTED_EDGE ( 'NONE', *, *, #23476, .F. ) ;
#20680=ORIENTED_EDGE ( 'NONE', *, *, #27843, .F. ) ;
#20683=VECTOR ( 'NONE', #8869, 1000.000000000000114 ) ;
#20686=FACE_OUTER_BOUND ( 'NONE', #1073, .T. ) ;
#20687=LINE ( 'NONE', #18264, #20408 ) ;
#20688=FACE_OUTER_BOUND ( 'NONE', #21980, .T. ) ;
#20689=LINE ( 'NONE', #3581, #6552 ) ;
#20696=DIRECTION ( 'NONE',  ( 0.000000000000000000, -1.000000000000000000, 0.000000000000000000 ) ) ;
#20698=FACE_OUTER_BOUND ( 'NONE', #9272, .T. ) ;
#20699=EDGE_CURVE ( 'NONE', #22709, #9224, #787, .T. ) ;
#20700=VECTOR ( 'NONE', #5466, 1000.000000000000000 ) ;
#20708=LINE ( 'NONE', #21274, #11318 ) ;
#20711=DIRECTION ( 'NONE',  ( -0.000000000000000000, -0.000000000000000000, -1.000000000000000000 ) ) ;
#20714=LINE ( 'NONE', #22743, #17840 ) ;
#20717=ORIENTED_EDGE ( 'NONE', *, *, #5908, .T. ) ;
#20719=LINE ( 'NONE', #5492, #14820 ) ;
#20720=AXIS2_PLACEMENT_3D ( 'NONE', #8732, #26250, #6576 ) ;
#20721=LINE ( 'NONE', #487, #24108 ) ;
#20722=CARTESIAN_POINT ( 'NONE',  ( 158.0000000000014779, 63.51174953456337136, -45.00000000000000000 ) ) ;
#20723=EDGE_CURVE ( 'NONE', #18134, #7521, #27474, .T. ) ;
#20726=DIRECTION ( 'NONE',  ( -0.8916010070293783896, -0.4528218681382319422, 0.000000000000000000 ) ) ;
#20731=DIRECTION ( 'NONE',  ( 0.000000000000000000, -1.000000000000000000, 0.000000000000000000 ) ) ;
#20733=EDGE_LOOP ( 'NONE', ( #9773, #3208, #10184, #19115 ) ) ;
#20734=DIRECTION ( 'NONE',  ( 0.000000000000000000, -1.000000000000000000, 0.000000000000000000 ) ) ;
#20735=ORIENTED_EDGE ( 'NONE', *, *, #2655, .F. ) ;
#20740=VERTEX_POINT ( 'NONE', #3067 ) ;
#20742=CARTESIAN_POINT ( 'NONE',  ( 158.0000000000009663, 115.6692496847042264, 45.00000000000000000 ) ) ;
#20744=ORIENTED_EDGE ( 'NONE', *, *, #22102, .T. ) ;
#20747=DIRECTION ( 'NONE',  ( -0.8916010070296023216, -0.4528218681377911281, 0.000000000000000000 ) ) ;
#20750=ORIENTED_EDGE ( 'NONE', *, *, #4436, .T. ) ;
#20754=ORIENTED_EDGE ( 'NONE', *, *, #9786, .F. ) ;
#20756=VECTOR ( 'NONE', #19944, 1000.000000000000000 ) ;
#20757=LINE ( 'NONE', #14306, #22130 ) ;
#20763=AXIS2_PLACEMENT_3D ( 'NONE', #23189, #3498, #12284 ) ;
#20770=FACE_OUTER_BOUND ( 'NONE', #26077, .T. ) ;
#20771=DIRECTION ( 'NONE',  ( 0.8916010070294402290, 0.4528218681381102617, 0.000000000000000000 ) ) ;
#20774=LINE ( 'NONE', #20918, #26353 ) ;
#20778=AXIS2_PLACEMENT_3D ( 'NONE', #13005, #12858, #21754 ) ;
#20779=EDGE_CURVE ( 'NONE', #855, #4042, #19290, .T. ) ;
#20782=CARTESIAN_POINT ( 'NONE',  ( 157.4999999999998579, 123.4468122109788482, -45.00000000000000000 ) ) ;
#20788=VECTOR ( 'NONE', #20747, 1000.000000000000000 ) ;
#20791=VERTEX_POINT ( 'NONE', #27615 ) ;
#20794=CARTESIAN_POINT ( 'NONE',  ( 167.4999999999996589, 258.6181251126050711, 6.000000000000019540 ) ) ;
#20796=DIRECTION ( 'NONE',  ( -0.000000000000000000, -0.000000000000000000, -1.000000000000000000 ) ) ;
#20797=ADVANCED_FACE ( 'NONE', ( #19146 ), #27756, .F. ) ;
#20800=EDGE_CURVE ( 'NONE', #11282, #4619, #16993, .T. ) ;
#20802=CARTESIAN_POINT ( 'NONE',  ( 158.0000000000001421, 193.4133749174225443, -45.00000000000000000 ) ) ;
#20806=FACE_OUTER_BOUND ( 'NONE', #13308, .T. ) ;
#20811=CARTESIAN_POINT ( 'NONE',  ( 158.0000000000002558, 181.3818748873943889, 45.00000000000000000 ) ) ;
#20815=CARTESIAN_POINT ( 'NONE',  ( 157.4999999999998579, 201.1909374436971802, -45.00000000000000000 ) ) ;
#20816=VERTEX_POINT ( 'NONE', #7954 ) ;
#20821=EDGE_CURVE ( 'NONE', #21780, #2305, #16721, .T. ) ;
#20825=VECTOR ( 'NONE', #5366, 1000.000000000000000 ) ;
#20827=CARTESIAN_POINT ( 'NONE',  ( 157.9999999999996305, 286.7126252026890256, 45.00000000000000000 ) ) ;
#20828=CARTESIAN_POINT ( 'NONE',  ( 157.4999999999998010, 241.3169375638095460, -45.00000000000000000 ) ) ;
#20829=LINE ( 'NONE', #9921, #9634 ) ;
#20832=EDGE_CURVE ( 'NONE', #6513, #6126, #3914, .T. ) ;
#20835=CARTESIAN_POINT ( 'NONE',  ( 157.9999999999996589, 278.6811251726610976, 45.00000000000000000 ) ) ;
#20836=CARTESIAN_POINT ( 'NONE',  ( 158.0000000000007958, 128.7164997297464595, -45.00000000000000000 ) ) ;
#20837=VECTOR ( 'NONE', #26466, 1000.000000000000000 ) ;
#20840=CARTESIAN_POINT ( 'NONE',  ( 158.0000000000012506, 86.08262460212675649, 45.00000000000000000 ) ) ;
#20842=CARTESIAN_POINT ( 'NONE',  ( 158.0000000000000284, 203.9527499549551806, 45.00000000000000000 ) ) ;
#20843=ORIENTED_EDGE ( 'NONE', *, *, #14849, .T. ) ;
#20849=ORIENTED_EDGE ( 'NONE', *, *, #20582, .T. ) ;
#20853=LINE ( 'NONE', #14120, #14512 ) ;
#20854=ORIENTED_EDGE ( 'NONE', *, *, #28211, .F. ) ;
#20856=ORIENTED_EDGE ( 'NONE', *, *, #2323, .F. ) ;
#20860=ORIENTED_EDGE ( 'NONE', *, *, #11520, .F. ) ;
#20861=EDGE_CURVE ( 'NONE', #23826, #11334, #17416, .T. ) ;
#20865=LINE ( 'NONE', #23022, #17106 ) ;
#20866=EDGE_CURVE ( 'NONE', #17812, #5015, #13263, .T. ) ;
#20868=CARTESIAN_POINT ( 'NONE',  ( 158.0000000000010516, 103.6377496546760568, 45.00000000000000000 ) ) ;
#20871=CARTESIAN_POINT ( 'NONE',  ( 157.4999999999998295, 228.7775625262745223, 45.00000000000000000 ) ) ;
#20875=DIRECTION ( 'NONE',  ( -0.8916010070298462376, -0.4528218681373109011, 0.000000000000000000 ) ) ;
#20878=DIRECTION ( 'NONE',  ( 0.4528218681383106015, -0.8916010070293384215, 0.000000000000000000 ) ) ;
#20879=LINE ( 'NONE', #16576, #5676 ) ;
#20881=VECTOR ( 'NONE', #21344, 1000.000000000000000 ) ;
#20882=DIRECTION ( 'NONE',  ( 0.8916010070293510781, -0.4528218681382856770, 0.000000000000000000 ) ) ;
#20884=DIRECTION ( 'NONE',  ( 0.8916010070293383105, -0.4528218681383106015, 0.000000000000000000 ) ) ;
#20886=DIRECTION ( 'NONE',  ( -0.8916010070296838119, -0.4528218681376305899, 0.000000000000000000 ) ) ;
#20887=ORIENTED_EDGE ( 'NONE', *, *, #20151, .F. ) ;
#20888=CARTESIAN_POINT ( 'NONE',  ( 158.0000000000002274, 183.8897498949014278, 45.00000000000000000 ) ) ;
#20891=PLANE ( 'NONE',  #2420 ) ;
#20893=VERTEX_POINT ( 'NONE', #15558 ) ;
#20895=LINE ( 'NONE', #5807, #18208 ) ;
#20897=EDGE_CURVE ( 'NONE', #24116, #27097, #22009, .T. ) ;
#20898=VECTOR ( 'NONE', #10836, 1000.000000000000000 ) ;
#20900=ORIENTED_EDGE ( 'NONE', *, *, #11461, .T. ) ;
#20901=VECTOR ( 'NONE', #15772, 1000.000000000000114 ) ;
#20905=CARTESIAN_POINT ( 'NONE',  ( 158.0000000000003126, 178.3661248723802828, -45.00000000000000000 ) ) ;
#20906=VECTOR ( 'NONE', #6518, 1000.000000000000000 ) ;
#20908=CARTESIAN_POINT ( 'NONE',  ( 158.0000000000016769, 47.95662448201407102, 45.00000000000000000 ) ) ;
#20909=CARTESIAN_POINT ( 'NONE',  ( 158.0000000000016769, 45.95662448201407102, 45.00000000000000000 ) ) ;
#20915=VERTEX_POINT ( 'NONE', #10957 ) ;
#20918=CARTESIAN_POINT ( 'NONE',  ( 158.0000000000003126, 178.3661248723802828, 45.00000000000000000 ) ) ;
#20919=AXIS2_PLACEMENT_3D ( 'NONE', #16705, #25318, #1047 ) ;
#20923=VECTOR ( 'NONE', #21485, 1000.000000000000000 ) ;
#20925=ORIENTED_EDGE ( 'NONE', *, *, #20355, .T. ) ;
#20926=CARTESIAN_POINT ( 'NONE',  ( 157.4999999999998579, 73.28931206083800021, 45.00000000000000000 ) ) ;
#20932=ORIENTED_EDGE ( 'NONE', *, *, #10406, .F. ) ;
#20933=ORIENTED_EDGE ( 'NONE', *, *, #12963, .T. ) ;
#20936=CARTESIAN_POINT ( 'NONE',  ( 157.4999999999997726, 248.8405625863305204, 45.00000000000000000 ) ) ;
#20939=CARTESIAN_POINT ( 'NONE',  ( 158.0000000000014779, 63.51174953456337136, -45.00000000000000000 ) ) ;
#20947=DIRECTION ( 'NONE',  ( 0.8916010070294904111, -0.4528218681380115074, 0.000000000000000000 ) ) ;
#20949=CARTESIAN_POINT ( 'NONE',  ( 157.4999999999998579, 113.4153121809506786, -45.00000000000000000 ) ) ;
#20950=ORIENTED_EDGE ( 'NONE', *, *, #28296, .T. ) ;
#20953=CARTESIAN_POINT ( 'NONE',  ( 157.9999999999998295, 226.0157500150140208, 45.00000000000000000 ) ) ;
#20954=ORIENTED_EDGE ( 'NONE', *, *, #13619, .F. ) ;
#20957=EDGE_CURVE ( 'NONE', #25380, #17988, #21871, .T. ) ;
#20959=EDGE_LOOP ( 'NONE', ( #363, #4512, #4690, #19620 ) ) ;
#20960=ORIENTED_EDGE ( 'NONE', *, *, #12141, .F. ) ;
#20964=EDGE_CURVE ( 'NONE', #477, #22143, #15421, .T. ) ;
#20965=ORIENTED_EDGE ( 'NONE', *, *, #3638, .F. ) ;
#20969=PLANE ( 'NONE',  #19421 ) ;
#20972=CARTESIAN_POINT ( 'NONE',  ( 157.4999999999998579, 60.74993702330277756, 45.00000000000000000 ) ) ;
#20976=CARTESIAN_POINT ( 'NONE',  ( 158.0000000000011653, 95.60624962464788723, 45.00000000000000000 ) ) ;
#20978=CARTESIAN_POINT ( 'NONE',  ( 157.4999999999998579, 100.8759371434154701, 45.00000000000000000 ) ) ;
#20985=EDGE_LOOP ( 'NONE', ( #19578, #27007, #11898, #11331 ) ) ;
#20987=VECTOR ( 'NONE', #3196, 1000.000000000000000 ) ;
#20990=EDGE_LOOP ( 'NONE', ( #6221, #17912, #3608, #1042 ) ) ;
#20992=LINE ( 'NONE', #10087, #14548 ) ;
#20994=LINE ( 'NONE', #23016, #21061 ) ;
#20995=ORIENTED_EDGE ( 'NONE', *, *, #18284, .F. ) ;
#21000=CARTESIAN_POINT ( 'NONE',  ( 158.0000000000006253, 146.2716247822957598, 45.00000000000000000 ) ) ;
#21002=DIRECTION ( 'NONE',  ( 0.4528218681379702626, -0.8916010070295112833, 0.000000000000000000 ) ) ;
#21005=VECTOR ( 'NONE', #12344, 1000.000000000000000 ) ;
#21006=ORIENTED_EDGE ( 'NONE', *, *, #13788, .T. ) ;
#21008=DIRECTION ( 'NONE',  ( 0.4528218681371922183, 0.8916010070299064116, -0.000000000000000000 ) ) ;
#21012=LINE ( 'NONE', #16301, #20825 ) ;
#21014=LINE ( 'NONE', #4049, #22900 ) ;
#21015=ORIENTED_EDGE ( 'NONE', *, *, #6659, .T. ) ;
#21018=DIRECTION ( 'NONE',  ( 1.000000000000000000, -0.000000000000000000, -0.000000000000000000 ) ) ;
#21019=ORIENTED_EDGE ( 'NONE', *, *, #22662, .T. ) ;
#21020=DIRECTION ( 'NONE',  ( 0.8916010070293584056, -0.4528218681382712996, 0.000000000000000000 ) ) ;
#21023=EDGE_LOOP ( 'NONE', ( #25304, #23392, #15676, #16206 ) ) ;
#21029=ORIENTED_EDGE ( 'NONE', *, *, #10623, .F. ) ;
#21030=ORIENTED_EDGE ( 'NONE', *, *, #16904, .T. ) ;
#21031=DIRECTION ( 'NONE',  ( 0.4528218681376106058, -0.8916010070296940260, 0.000000000000000000 ) ) ;
#21040=LINE ( 'NONE', #14730, #25679 ) ;
#21041=DIRECTION ( 'NONE',  ( -0.000000000000000000, -0.000000000000000000, -1.000000000000000000 ) ) ;
#21047=CARTESIAN_POINT ( 'NONE',  ( 157.4999999999998579, 80.81293708335913095, 45.00000000000000000 ) ) ;
#21049=CARTESIAN_POINT ( 'NONE',  ( 158.0000000000001990, 186.3976249024084666, 45.00000000000000000 ) ) ;
#21050=ORIENTED_EDGE ( 'NONE', *, *, #3205, .F. ) ;
#21053=AXIS2_PLACEMENT_3D ( 'NONE', #1786, #28208, #13019 ) ;
#21055=AXIS2_PLACEMENT_3D ( 'NONE', #18963, #3721, #27563 ) ;
#21060=ORIENTED_EDGE ( 'NONE', *, *, #9358, .T. ) ;
#21061=VECTOR ( 'NONE', #9671, 1000.000000000000000 ) ;
#21069=VECTOR ( 'NONE', #20734, 1000.000000000000000 ) ;
#21071=ORIENTED_EDGE ( 'NONE', *, *, #10364, .F. ) ;
#21074=CARTESIAN_POINT ( 'NONE',  ( 158.0000000000007105, 138.2401247522676044, 45.00000000000000000 ) ) ;
#21077=PLANE ( 'NONE',  #15603 ) ;
#21078=AXIS2_PLACEMENT_3D ( 'NONE', #5877, #10479, #14939 ) ;
#21085=PLANE ( 'NONE',  #3573 ) ;
#21086=DIRECTION ( 'NONE',  ( -0.000000000000000000, -0.000000000000000000, -1.000000000000000000 ) ) ;
#21095=CARTESIAN_POINT ( 'NONE',  ( 158.0000000000010800, 103.1298746471690038, -45.00000000000000000 ) ) ;
#21096=ORIENTED_EDGE ( 'NONE', *, *, #13847, .T. ) ;
#21099=EDGE_CURVE ( 'NONE', #14425, #7228, #14345, .T. ) ;
#21101=EDGE_LOOP ( 'NONE', ( #13235, #12728, #22240, #6179 ) ) ;
#21103=EDGE_LOOP ( 'NONE', ( #19979, #2176, #25659, #4522 ) ) ;
#21109=VECTOR ( 'NONE', #1709, 999.9999999999998863 ) ;
#21111=EDGE_CURVE ( 'NONE', #24116, #22290, #3263, .T. ) ;
#21115=DIRECTION ( 'NONE',  ( -0.000000000000000000, -0.000000000000000000, -1.000000000000000000 ) ) ;
#21119=VERTEX_POINT ( 'NONE', #20939 ) ;
#21126=ORIENTED_EDGE ( 'NONE', *, *, #15350, .T. ) ;
#21129=EDGE_CURVE ( 'NONE', #21244, #1387, #24185, .T. ) ;
#21130=CARTESIAN_POINT ( 'NONE',  ( 157.9999999999997158, 259.1260001201120531, 45.00000000000000000 ) ) ;
#21136=CARTESIAN_POINT ( 'NONE',  ( 157.9999999999997158, 259.1260001201120531, -45.00000000000000000 ) ) ;
#21137=VERTEX_POINT ( 'NONE', #17568 ) ;
#21139=ORIENTED_EDGE ( 'NONE', *, *, #17251, .F. ) ;
#21148=ADVANCED_FACE ( 'NONE', ( #26608 ), #20153, .F. ) ;
#21152=CARTESIAN_POINT ( 'NONE',  ( 217.4999999999996305, 258.6181251126050711, 1.387778780781445676E-14 ) ) ;
#21153=ADVANCED_FACE ( 'NONE', ( #24467 ), #2188, .F. ) ;
#21162=CARTESIAN_POINT ( 'NONE',  ( 158.0000000000007958, 128.7164997297464595, -45.00000000000000000 ) ) ;
#21165=CARTESIAN_POINT ( 'NONE',  ( 157.4999999999998579, 90.84443711338730054, 45.00000000000000000 ) ) ;
#21166=VERTEX_POINT ( 'NONE', #10971 ) ;
#21167=VECTOR ( 'NONE', #18060, 1000.000000000000000 ) ;
#21168=LINE ( 'NONE', #10824, #19344 ) ;
#21169=LINE ( 'NONE', #8243, #8539 ) ;
#21171=VECTOR ( 'NONE', #364, 1000.000000000000000 ) ;
#21172=ORIENTED_EDGE ( 'NONE', *, *, #4597, .F. ) ;
#21174=ORIENTED_EDGE ( 'NONE', *, *, #12847, .T. ) ;
#21178=LINE ( 'NONE', #25626, #153 ) ;
#21182=EDGE_CURVE ( 'NONE', #27871, #1905, #9096, .T. ) ;
#21189=DIRECTION ( 'NONE',  ( -0.8916010070296327417, 0.4528218681377311206, 0.000000000000000000 ) ) ;
#21190=VECTOR ( 'NONE', #5054, 1000.000000000000000 ) ;
#21191=CARTESIAN_POINT ( 'NONE',  ( 158.0000000000013927, 75.54324956459154805, -45.00000000000000000 ) ) ;
#21192=LINE ( 'NONE', #28344, #8891 ) ;
#21197=FACE_OUTER_BOUND ( 'NONE', #3926, .T. ) ;
#21199=DIRECTION ( 'NONE',  ( -0.8916010070295922185, -0.4528218681378110566, 0.000000000000000000 ) ) ;
#21202=VERTEX_POINT ( 'NONE', #17427 ) ;
#21204=VERTEX_POINT ( 'NONE', #6368 ) ;
#21206=VERTEX_POINT ( 'NONE', #10829 ) ;
#21210=ORIENTED_EDGE ( 'NONE', *, *, #8026, .T. ) ;
#21211=VERTEX_POINT ( 'NONE', #6933 ) ;
#21212=VECTOR ( 'NONE', #7703, 1000.000000000000114 ) ;
#21214=LINE ( 'NONE', #14761, #10988 ) ;
#21215=CARTESIAN_POINT ( 'NONE',  ( 158.0000000000007105, 136.2401247522676044, 45.00000000000000000 ) ) ;
#21216=AXIS2_PLACEMENT_3D ( 'NONE', #21737, #11656, #11214 ) ;
#21228=DIRECTION ( 'NONE',  ( -0.8916010070297751833, -0.4528218681374507892, 0.000000000000000000 ) ) ;
#21230=VECTOR ( 'NONE', #15045, 1000.000000000000114 ) ;
#21231=VECTOR ( 'NONE', #26416, 1000.000000000000000 ) ;
#21234=AXIS2_PLACEMENT_3D ( 'NONE', #16334, #25083, #22929 ) ;
#21237=VECTOR ( 'NONE', #23646, 1000.000000000000000 ) ;
#21239=VERTEX_POINT ( 'NONE', #20006 ) ;
#21240=ORIENTED_EDGE ( 'NONE', *, *, #25718, .F. ) ;
#21241=VERTEX_POINT ( 'NONE', #9241 ) ;
#21242=ORIENTED_EDGE ( 'NONE', *, *, #24398, .F. ) ;
#21244=VERTEX_POINT ( 'NONE', #26046 ) ;
#21257=ADVANCED_FACE ( 'NONE', ( #48 ), #22166, .F. ) ;
#21270=VERTEX_POINT ( 'NONE', #22876 ) ;
#21274=CARTESIAN_POINT ( 'NONE',  ( 158.0000000000003126, 176.3661248723802828, -45.00000000000000000 ) ) ;
#21275=ORIENTED_EDGE ( 'NONE', *, *, #25462, .F. ) ;
#21277=DIRECTION ( 'NONE',  ( -0.8916010070298462376, -0.4528218681373109011, 0.000000000000000000 ) ) ;
#21278=EDGE_CURVE ( 'NONE', #8983, #21204, #9391, .T. ) ;
#21279=CARTESIAN_POINT ( 'NONE',  ( 157.4999999999994600, 216.2381874887387880, -45.00000000000000000 ) ) ;
#21283=ORIENTED_EDGE ( 'NONE', *, *, #24019, .T. ) ;
#21286=LINE ( 'NONE', #14978, #1114 ) ;
#21287=LINE ( 'NONE', #27742, #18168 ) ;
#21288=VECTOR ( 'NONE', #26740, 1000.000000000000227 ) ;
#21294=EDGE_CURVE ( 'NONE', #2548, #17145, #14265, .T. ) ;
#21297=DIRECTION ( 'NONE',  ( -0.8916010070317489378, 0.4528218681335642870, 0.000000000000000000 ) ) ;
#21299=ORIENTED_EDGE ( 'NONE', *, *, #21986, .T. ) ;
#21300=DIRECTION ( 'NONE',  ( 0.8916010070299578150, 0.4528218681370910770, 0.000000000000000000 ) ) ;
#21302=CARTESIAN_POINT ( 'NONE',  ( 158.0000000000013927, 75.54324956459154805, 45.00000000000000000 ) ) ;
#21303=CARTESIAN_POINT ( 'NONE',  ( 157.4999999999998579, 93.35231212089433939, 45.00000000000000000 ) ) ;
#21305=DIRECTION ( 'NONE',  ( 0.4528218681380902222, -0.8916010070294504430, 0.000000000000000000 ) ) ;
#21306=CARTESIAN_POINT ( 'NONE',  ( 158.0000000000008527, 123.7007497147323960, -45.00000000000000000 ) ) ;
#21307=ORIENTED_EDGE ( 'NONE', *, *, #664, .T. ) ;
#21309=ADVANCED_FACE ( 'NONE', ( #13705 ), #22601, .F. ) ;
#21311=DIRECTION ( 'NONE',  ( 0.000000000000000000, -1.000000000000000000, 0.000000000000000000 ) ) ;
#21312=VERTEX_POINT ( 'NONE', #5348 ) ;
#21314=ORIENTED_EDGE ( 'NONE', *, *, #7556, .F. ) ;
#21315=EDGE_CURVE ( 'NONE', #3398, #24937, #1179, .T. ) ;
#21316=CARTESIAN_POINT ( 'NONE',  ( 158.0000000000013927, 73.54324956459154805, 45.00000000000000000 ) ) ;
#21319=VERTEX_POINT ( 'NONE', #11973 ) ;
#21321=DIRECTION ( 'NONE',  ( -0.000000000000000000, -0.000000000000000000, -1.000000000000000000 ) ) ;
#21322=DIRECTION ( 'NONE',  ( 0.4528218681371310450, -0.8916010070299376089, 0.000000000000000000 ) ) ;
#21323=LINE ( 'NONE', #1119, #655 ) ;
#21325=AXIS2_PLACEMENT_3D ( 'NONE', #7460, #2993, #982 ) ;
#21329=VERTEX_POINT ( 'NONE', #27313 ) ;
#21330=CARTESIAN_POINT ( 'NONE',  ( 157.9999999999996305, 288.7126252026890256, 45.00000000000000000 ) ) ;
#21334=LINE ( 'NONE', #1928, #3841 ) ;
#21341=ORIENTED_EDGE ( 'NONE', *, *, #7890, .F. ) ;
#21343=VERTEX_POINT ( 'NONE', #11555 ) ;
#21344=DIRECTION ( 'NONE',  ( -0.000000000000000000, -0.000000000000000000, -1.000000000000000000 ) ) ;
#21346=AXIS2_PLACEMENT_3D ( 'NONE', #26912, #5354, #15871 ) ;
#21352=DIRECTION ( 'NONE',  ( -0.000000000000000000, -0.000000000000000000, -1.000000000000000000 ) ) ;
#21353=ORIENTED_EDGE ( 'NONE', *, *, #18687, .T. ) ;
#21358=CARTESIAN_POINT ( 'NONE',  ( 157.9999999999999716, 208.9684999699701393, 45.00000000000000000 ) ) ;
#21360=DIRECTION ( 'NONE',  ( -0.8916010070296733758, -0.4528218681376511845, 0.000000000000000000 ) ) ;
#21361=DIRECTION ( 'NONE',  ( -0.000000000000000000, 0.000000000000000000, -1.000000000000000000 ) ) ;
#21371=AXIS2_PLACEMENT_3D ( 'NONE', #7117, #20186, #4807 ) ;
#21374=DIRECTION ( 'NONE',  ( 0.4528218681383305855, -0.8916010070293283185, 0.000000000000000000 ) ) ;
#21381=ORIENTED_EDGE ( 'NONE', *, *, #13652, .F. ) ;
#21382=ORIENTED_EDGE ( 'NONE', *, *, #4597, .T. ) ;
#21385=EDGE_CURVE ( 'NONE', #1213, #5230, #11834, .T. ) ;
#21387=EDGE_CURVE ( 'NONE', #27632, #17961, #15864, .T. ) ;
#21389=ORIENTED_EDGE ( 'NONE', *, *, #28250, .F. ) ;
#21390=ORIENTED_EDGE ( 'NONE', *, *, #16682, .F. ) ;
#21391=VECTOR ( 'NONE', #22059, 1000.000000000000000 ) ;
#21392=CARTESIAN_POINT ( 'NONE',  ( 157.9999999999996305, 284.2047501951820436, 45.00000000000000000 ) ) ;
#21394=VECTOR ( 'NONE', #19460, 1000.000000000000000 ) ;
#21395=FACE_OUTER_BOUND ( 'NONE', #13952, .T. ) ;
#21403=CARTESIAN_POINT ( 'NONE',  ( 157.4999999999998579, 151.0334372935563465, 45.00000000000000000 ) ) ;
#21404=VERTEX_POINT ( 'NONE', #24611 ) ;
#21408=EDGE_CURVE ( 'NONE', #21673, #2119, #16698, .T. ) ;
#21409=LINE ( 'NONE', #14531, #7153 ) ;
#21410=ORIENTED_EDGE ( 'NONE', *, *, #20821, .T. ) ;
#21412=VERTEX_POINT ( 'NONE', #21279 ) ;
#21414=DIRECTION ( 'NONE',  ( 0.8916010070293710621, -0.4528218681382463195, 0.000000000000000000 ) ) ;
#21424=ORIENTED_EDGE ( 'NONE', *, *, #22173, .T. ) ;
#21425=VECTOR ( 'NONE', #21277, 1000.000000000000114 ) ;
#21433=CARTESIAN_POINT ( 'NONE',  ( 157.4999999999997158, 258.8720626163585621, -45.00000000000000000 ) ) ;
#21438=EDGE_CURVE ( 'NONE', #19932, #21119, #3603, .T. ) ;
#21441=LINE ( 'NONE', #26031, #18381 ) ;
#21443=EDGE_LOOP ( 'NONE', ( #23511, #10327, #5527, #14148 ) ) ;
#21445=VERTEX_POINT ( 'NONE', #8070 ) ;
#21447=DIRECTION ( 'NONE',  ( 0.8916010070295820045, 0.4528218681378310406, 0.000000000000000000 ) ) ;
#21451=DIRECTION ( 'NONE',  ( 0.000000000000000000, -1.000000000000000000, 0.000000000000000000 ) ) ;
#21452=EDGE_LOOP ( 'NONE', ( #22443, #10823, #13564, #9376 ) ) ;
#21454=ADVANCED_FACE ( 'NONE', ( #16833 ), #27733, .F. ) ;
#21455=ORIENTED_EDGE ( 'NONE', *, *, #4498, .F. ) ;
#21461=CARTESIAN_POINT ( 'NONE',  ( 157.9999999999997442, 256.1102501050980322, -45.00000000000000000 ) ) ;
#21469=DIRECTION ( 'NONE',  ( 1.000000000000000000, 0.000000000000000000, -0.000000000000000000 ) ) ;
#21470=LINE ( 'NONE', #3519, #9718 ) ;
#21472=LINE ( 'NONE', #16885, #12579 ) ;
#21473=VERTEX_POINT ( 'NONE', #7013 ) ;
#21476=CARTESIAN_POINT ( 'NONE',  ( 157.4999999999996305, 288.9665627064425735, -45.00000000000000000 ) ) ;
#21481=EDGE_LOOP ( 'NONE', ( #1835, #17843, #25819, #11421 ) ) ;
#21482=VECTOR ( 'NONE', #24372, 1000.000000000000000 ) ;
#21485=DIRECTION ( 'NONE',  ( -0.000000000000000000, -0.000000000000000000, -1.000000000000000000 ) ) ;
#21486=VECTOR ( 'NONE', #19068, 1000.000000000000000 ) ;
#21489=CARTESIAN_POINT ( 'NONE',  ( 158.0000000000007390, 133.7322497447605656, 45.00000000000000000 ) ) ;
#21495=LINE ( 'NONE', #21358, #21230 ) ;
#21496=AXIS2_PLACEMENT_3D ( 'NONE', #21542, #12661, #23848 ) ;
#21499=VECTOR ( 'NONE', #10563, 1000.000000000000000 ) ;
#21507=CARTESIAN_POINT ( 'NONE',  ( 157.9999999999996305, 281.6968751876750616, 45.00000000000000000 ) ) ;
#21510=VECTOR ( 'NONE', #27589, 1000.000000000000114 ) ;
#21511=EDGE_CURVE ( 'NONE', #18838, #2768, #4706, .T. ) ;
#21519=VECTOR ( 'NONE', #21582, 999.9999999999998863 ) ;
#21521=EDGE_LOOP ( 'NONE', ( #20392, #18717, #25765, #10322 ) ) ;
#21522=ORIENTED_EDGE ( 'NONE', *, *, #20699, .T. ) ;
#21523=AXIS2_PLACEMENT_3D ( 'NONE', #5351, #22457, #13563 ) ;
#21524=EDGE_LOOP ( 'NONE', ( #12297, #14050, #17560, #19722 ) ) ;
#21533=CARTESIAN_POINT ( 'NONE',  ( 157.4999999999998579, 186.1436873986549188, 45.00000000000000000 ) ) ;
#21542=CARTESIAN_POINT ( 'NONE',  ( 157.4999999999998579, 178.6200623761337738, 45.00000000000000000 ) ) ;
#21546=DIRECTION ( 'NONE',  ( 0.8916010070298556744, -0.4528218681372921384, 0.000000000000000000 ) ) ;
#21547=ORIENTED_EDGE ( 'NONE', *, *, #11378, .F. ) ;
#21549=VECTOR ( 'NONE', #839, 1000.000000000000000 ) ;
#21551=ORIENTED_EDGE ( 'NONE', *, *, #13619, .T. ) ;
#21553=ORIENTED_EDGE ( 'NONE', *, *, #10019, .F. ) ;
#21559=ORIENTED_EDGE ( 'NONE', *, *, #25834, .F. ) ;
#21564=VERTEX_POINT ( 'NONE', #28158 ) ;
#21566=ORIENTED_EDGE ( 'NONE', *, *, #12906, .T. ) ;
#21568=EDGE_CURVE ( 'NONE', #26462, #5196, #2022, .T. ) ;
#21569=EDGE_CURVE ( 'NONE', #3560, #10864, #2840, .T. ) ;
#21570=DIRECTION ( 'NONE',  ( 0.4528218681371523058, 0.8916010070299268397, -0.000000000000000000 ) ) ;
#21572=EDGE_CURVE ( 'NONE', #24562, #2081, #5141, .T. ) ;
#21573=CARTESIAN_POINT ( 'NONE',  ( 0.000000000000000000, 0.000000000000000000, 45.00000000000000000 ) ) ;
#21574=ORIENTED_EDGE ( 'NONE', *, *, #14419, .T. ) ;
#21575=VECTOR ( 'NONE', #18478, 1000.000000000000114 ) ;
#21578=LINE ( 'NONE', #17267, #3697 ) ;
#21579=CARTESIAN_POINT ( 'NONE',  ( 158.0000000000003126, 178.3661248723802828, 45.00000000000000000 ) ) ;
#21581=ORIENTED_EDGE ( 'NONE', *, *, #23785, .F. ) ;
#21582=DIRECTION ( 'NONE',  ( 0.8916010070293584056, -0.4528218681382712996, 0.000000000000000000 ) ) ;
#21586=FACE_OUTER_BOUND ( 'NONE', #24810, .T. ) ;
#21594=VERTEX_POINT ( 'NONE', #2551 ) ;
#21596=ORIENTED_EDGE ( 'NONE', *, *, #28077, .T. ) ;
#21597=AXIS2_PLACEMENT_3D ( 'NONE', #12269, #25883, #8366 ) ;
#21598=VERTEX_POINT ( 'NONE', #11634 ) ;
#21600=ORIENTED_EDGE ( 'NONE', *, *, #10845, .F. ) ;
#21602=VECTOR ( 'NONE', #6031, 1000.000000000000000 ) ;
#21606=LINE ( 'NONE', #10699, #1627 ) ;
#21613=DIRECTION ( 'NONE',  ( -0.000000000000000000, 0.000000000000000000, -1.000000000000000000 ) ) ;
#21615=DIRECTION ( 'NONE',  ( 0.000000000000000000, -1.000000000000000000, 0.000000000000000000 ) ) ;
#21618=EDGE_CURVE ( 'NONE', #2305, #11934, #413, .T. ) ;
#21619=AXIS2_PLACEMENT_3D ( 'NONE', #23212, #18895, #21189 ) ;
#21620=DIRECTION ( 'NONE',  ( -0.8916010070296429557, -0.4528218681377111920, 0.000000000000000000 ) ) ;
#21622=FACE_OUTER_BOUND ( 'NONE', #17518, .T. ) ;
#21623=CARTESIAN_POINT ( 'NONE',  ( 157.9999999999996305, 286.7126252026890256, -45.00000000000000000 ) ) ;
#21624=LINE ( 'NONE', #16892, #10639 ) ;
#21625=VERTEX_POINT ( 'NONE', #7162 ) ;
#21626=VECTOR ( 'NONE', #2356, 1000.000000000000000 ) ;
#21632=ADVANCED_FACE ( 'NONE', ( #27116 ), #12196, .F. ) ;
#21634=LINE ( 'NONE', #11300, #3030 ) ;
#21636=EDGE_LOOP ( 'NONE', ( #11626, #7810, #5136, #2600 ) ) ;
#21637=ORIENTED_EDGE ( 'NONE', *, *, #25821, .F. ) ;
#21638=DIRECTION ( 'NONE',  ( 1.000000000000000000, 0.000000000000000000, -0.000000000000000000 ) ) ;
#21640=FACE_OUTER_BOUND ( 'NONE', #25260, .T. ) ;
#21641=EDGE_CURVE ( 'NONE', #20791, #19423, #1255, .T. ) ;
#21644=DIRECTION ( 'NONE',  ( 1.000000000000000000, 0.000000000000000000, -0.000000000000000000 ) ) ;
#21645=VECTOR ( 'NONE', #27624, 1000.000000000000000 ) ;
#21651=FACE_OUTER_BOUND ( 'NONE', #12278, .T. ) ;
#21652=FACE_OUTER_BOUND ( 'NONE', #21452, .T. ) ;
#21653=DIRECTION ( 'NONE',  ( 0.000000000000000000, -1.000000000000000000, 0.000000000000000000 ) ) ;
#21654=CARTESIAN_POINT ( 'NONE',  ( 157.4999999999998295, 40.68693696324645970, 45.00000000000000000 ) ) ;
#21661=ORIENTED_EDGE ( 'NONE', *, *, #8352, .T. ) ;
#21666=AXIS2_PLACEMENT_3D ( 'NONE', #6045, #14825, #23576 ) ;
#21668=EDGE_LOOP ( 'NONE', ( #2289, #20078, #21844, #20433 ) ) ;
#21669=AXIS2_PLACEMENT_3D ( 'NONE', #23119, #16795, #16242 ) ;
#21673=VERTEX_POINT ( 'NONE', #10165 ) ;
#21675=DIRECTION ( 'NONE',  ( -0.000000000000000000, 0.000000000000000000, -1.000000000000000000 ) ) ;
#21677=FACE_OUTER_BOUND ( 'NONE', #4988, .T. ) ;
#21687=CARTESIAN_POINT ( 'NONE',  ( 158.0000000000002842, 178.8739998798873216, -45.00000000000000000 ) ) ;
#21692=DIRECTION ( 'NONE',  ( -0.8916010070295820045, -0.4528218681378310406, 0.000000000000000000 ) ) ;
#21693=CARTESIAN_POINT ( 'NONE',  ( 157.4999999999998579, 90.84443711338730054, 45.00000000000000000 ) ) ;
#21697=LINE ( 'NONE', #18973, #25946 ) ;
#21703=VECTOR ( 'NONE', #22045, 1000.000000000000114 ) ;
#21708=ORIENTED_EDGE ( 'NONE', *, *, #17787, .T. ) ;
#21709=EDGE_CURVE ( 'NONE', #26764, #11364, #11772, .T. ) ;
#21714=ORIENTED_EDGE ( 'NONE', *, *, #19550, .F. ) ;
#21720=VECTOR ( 'NONE', #2029, 1000.000000000000000 ) ;
#21723=AXIS2_PLACEMENT_3D ( 'NONE', #2473, #11261, #18289 ) ;
#21725=EDGE_CURVE ( 'NONE', #10196, #14755, #5565, .T. ) ;
#21727=CARTESIAN_POINT ( 'NONE',  ( 157.4999999999998579, 48.21056198576756202, 45.00000000000000000 ) ) ;
#21728=VECTOR ( 'NONE', #13158, 999.9999999999998863 ) ;
#21729=CARTESIAN_POINT ( 'NONE',  ( 158.0000000000001705, 190.9054999099155054, -45.00000000000000000 ) ) ;
#21730=ORIENTED_EDGE ( 'NONE', *, *, #24150, .T. ) ;
#21736=ORIENTED_EDGE ( 'NONE', *, *, #23009, .T. ) ;
#21737=CARTESIAN_POINT ( 'NONE',  ( 157.9999999999999716, 210.9684999699701393, 45.00000000000000000 ) ) ;
#21743=VECTOR ( 'NONE', #4635, 1000.000000000000000 ) ;
#21746=CARTESIAN_POINT ( 'NONE',  ( 157.9999999999997726, 246.5866250825770294, -45.00000000000000000 ) ) ;
#21747=ORIENTED_EDGE ( 'NONE', *, *, #26768, .F. ) ;
#21750=ADVANCED_FACE ( 'NONE', ( #3829 ), #10446, .F. ) ;
#21751=EDGE_LOOP ( 'NONE', ( #16872, #5544, #20463, #17777 ) ) ;
#21752=ORIENTED_EDGE ( 'NONE', *, *, #15722, .F. ) ;
#21754=DIRECTION ( 'NONE',  ( -0.000000000000000000, 0.000000000000000000, -1.000000000000000000 ) ) ;
#21761=VERTEX_POINT ( 'NONE', #6269 ) ;
#21762=CARTESIAN_POINT ( 'NONE',  ( 157.9999999999997726, 243.5708750675630370, 45.00000000000000000 ) ) ;
#21766=VERTEX_POINT ( 'NONE', #10305 ) ;
#21767=AXIS2_PLACEMENT_3D ( 'NONE', #11530, #6631, #15407 ) ;
#21768=CARTESIAN_POINT ( 'NONE',  ( 157.9999999999999147, 213.9842499849850697, -45.00000000000000000 ) ) ;
#21770=CARTESIAN_POINT ( 'NONE',  ( 157.4999999999996305, 286.4586876989355915, 45.00000000000000000 ) ) ;
#21771=PLANE ( 'NONE',  #22719 ) ;
#21773=DIRECTION ( 'NONE',  ( -0.000000000000000000, 1.000000000000000000, -0.000000000000000000 ) ) ;
#21774=AXIS2_PLACEMENT_3D ( 'NONE', #17484, #2250, #6284 ) ;
#21775=ORIENTED_EDGE ( 'NONE', *, *, #9471, .F. ) ;
#21778=ORIENTED_EDGE ( 'NONE', *, *, #5060, .T. ) ;
#21780=VERTEX_POINT ( 'NONE', #12896 ) ;
#21781=VERTEX_POINT ( 'NONE', #12616 ) ;
#21782=CARTESIAN_POINT ( 'NONE',  ( 157.4999999999998579, 176.1121873686267350, 45.00000000000000000 ) ) ;
#21783=ADVANCED_FACE ( 'NONE', ( #21640 ), #8576, .F. ) ;
#21787=VECTOR ( 'NONE', #9042, 1000.000000000000227 ) ;
#21790=EDGE_CURVE ( 'NONE', #25403, #6335, #21495, .T. ) ;
#21791=CARTESIAN_POINT ( 'NONE',  ( 158.0000000000008811, 123.1928747072253572, 45.00000000000000000 ) ) ;
#21793=VECTOR ( 'NONE', #20886, 1000.000000000000000 ) ;
#21794=LINE ( 'NONE', #526, #5503 ) ;
#21800=DIRECTION ( 'NONE',  ( 1.000000000000000000, 0.000000000000000000, -0.000000000000000000 ) ) ;
#21804=LINE ( 'NONE', #1970, #5017 ) ;
#21806=VECTOR ( 'NONE', #2097, 1000.000000000000000 ) ;
#21808=VERTEX_POINT ( 'NONE', #19064 ) ;
#21810=EDGE_CURVE ( 'NONE', #729, #26706, #23661, .T. ) ;
#21818=ORIENTED_EDGE ( 'NONE', *, *, #25411, .F. ) ;
#21821=EDGE_CURVE ( 'NONE', #19430, #16733, #23373, .T. ) ;
#21823=VECTOR ( 'NONE', #20585, 999.9999999999998863 ) ;
#21826=DIRECTION ( 'NONE',  ( -0.000000000000000000, -0.000000000000000000, -1.000000000000000000 ) ) ;
#21828=LINE ( 'NONE', #19805, #20683 ) ;
#21830=CARTESIAN_POINT ( 'NONE',  ( 158.0000000000006537, 141.2558747672816821, -45.00000000000000000 ) ) ;
#21832=PLANE ( 'NONE',  #4471 ) ;
#21835=EDGE_CURVE ( 'NONE', #18558, #6129, #17191, .T. ) ;
#21839=CARTESIAN_POINT ( 'NONE',  ( 158.0000000000005400, 153.7952498048169048, -45.00000000000000000 ) ) ;
#21840=ORIENTED_EDGE ( 'NONE', *, *, #11907, .F. ) ;
#21843=CARTESIAN_POINT ( 'NONE',  ( 157.4999999999998579, 133.4783122410070462, -45.00000000000000000 ) ) ;
#21844=ORIENTED_EDGE ( 'NONE', *, *, #20672, .F. ) ;
#21847=ORIENTED_EDGE ( 'NONE', *, *, #13363, .F. ) ;
#21848=VECTOR ( 'NONE', #21414, 1000.000000000000114 ) ;
#21856=LINE ( 'NONE', #24579, #26100 ) ;
#21859=EDGE_LOOP ( 'NONE', ( #10690, #17810, #12578, #12276 ) ) ;
#21861=LINE ( 'NONE', #24294, #18104 ) ;
#21868=ORIENTED_EDGE ( 'NONE', *, *, #7517, .T. ) ;
#21871=LINE ( 'NONE', #15281, #24952 ) ;
#21872=PLANE ( 'NONE',  #20412 ) ;
#21874=EDGE_CURVE ( 'NONE', #465, #20505, #1363, .T. ) ;
#21875=ORIENTED_EDGE ( 'NONE', *, *, #26982, .F. ) ;
#21876=DIRECTION ( 'NONE',  ( -0.8916010070293584056, 0.4528218681382713551, 0.000000000000000000 ) ) ;
#21879=AXIS2_PLACEMENT_3D ( 'NONE', #12397, #1453, #12536 ) ;
#21887=EDGE_CURVE ( 'NONE', #9116, #11111, #16186, .T. ) ;
#21888=LINE ( 'NONE', #17574, #20898 ) ;
#21889=CARTESIAN_POINT ( 'NONE',  ( 158.0000000000011369, 98.11412463215494029, 45.00000000000000000 ) ) ;
#21891=DIRECTION ( 'NONE',  ( 0.8916010070298867607, 0.4528218681372308541, 0.000000000000000000 ) ) ;
#21895=CARTESIAN_POINT ( 'NONE',  ( 158.0000000000003126, 176.3661248723802828, 45.00000000000000000 ) ) ;
#21896=ADVANCED_FACE ( 'NONE', ( #7273 ), #9989, .F. ) ;
#21897=CARTESIAN_POINT ( 'NONE',  ( 157.9999999999997726, 244.0787500750700474, -45.00000000000000000 ) ) ;
#21898=CARTESIAN_POINT ( 'NONE',  ( 157.9999999999996874, 264.1417501351260171, 45.00000000000000000 ) ) ;
#21900=VECTOR ( 'NONE', #24254, 1000.000000000000000 ) ;
#21903=DIRECTION ( 'NONE',  ( 1.000000000000000000, 0.000000000000000000, -0.000000000000000000 ) ) ;
#21906=ADVANCED_FACE ( 'NONE', ( #14038 ), #22785, .F. ) ;
#21907=DIRECTION ( 'NONE',  ( 0.8916010070293783896, -0.4528218681382319422, 0.000000000000000000 ) ) ;
#21911=CARTESIAN_POINT ( 'NONE',  ( 158.0000000000013927, 73.54324956459154805, -45.00000000000000000 ) ) ;
#21912=ORIENTED_EDGE ( 'NONE', *, *, #5841, .T. ) ;
#21914=ORIENTED_EDGE ( 'NONE', *, *, #10270, .T. ) ;
#21915=FACE_OUTER_BOUND ( 'NONE', #27903, .T. ) ;
#21917=EDGE_LOOP ( 'NONE', ( #21126, #22315, #17743, #16355 ) ) ;
#21918=LINE ( 'NONE', #26221, #2109 ) ;
#21926=EDGE_CURVE ( 'NONE', #1420, #19053, #20757, .T. ) ;
#21928=ADVANCED_FACE ( 'NONE', ( #16460 ), #25210, .F. ) ;
#21933=CARTESIAN_POINT ( 'NONE',  ( 157.4999999999994884, 211.2224374737238577, -45.00000000000000000 ) ) ;
#21934=LINE ( 'NONE', #13191, #26517 ) ;
#21936=EDGE_LOOP ( 'NONE', ( #659, #2506, #1140, #23968 ) ) ;
#21941=FACE_OUTER_BOUND ( 'NONE', #18119, .T. ) ;
#21947=DIRECTION ( 'NONE',  ( 0.8916010070293383105, -0.4528218681383106015, 0.000000000000000000 ) ) ;
#21948=ORIENTED_EDGE ( 'NONE', *, *, #27441, .F. ) ;
#21951=ORIENTED_EDGE ( 'NONE', *, *, #22716, .F. ) ;
#21952=ORIENTED_EDGE ( 'NONE', *, *, #16016, .F. ) ;
#21957=CARTESIAN_POINT ( 'NONE',  ( 158.0000000000006537, 143.2558747672816821, 45.00000000000000000 ) ) ;
#21961=ADVANCED_FACE ( 'NONE', ( #3511 ), #12299, .F. ) ;
#21965=DIRECTION ( 'NONE',  ( -0.000000000000000000, -0.000000000000000000, -1.000000000000000000 ) ) ;
#21967=AXIS2_PLACEMENT_3D ( 'NONE', #22188, #4795, #13296 ) ;
#21971=CARTESIAN_POINT ( 'NONE',  ( 157.4999999999996305, 288.9665627064425735, 45.00000000000000000 ) ) ;
#21975=VECTOR ( 'NONE', #24064, 1000.000000000000000 ) ;
#21980=EDGE_LOOP ( 'NONE', ( #18527, #8, #24356, #23996 ) ) ;
#21981=ORIENTED_EDGE ( 'NONE', *, *, #23394, .F. ) ;
#21982=ORIENTED_EDGE ( 'NONE', *, *, #14390, .F. ) ;
#21986=EDGE_CURVE ( 'NONE', #18534, #4389, #3792, .T. ) ;
#21988=EDGE_CURVE ( 'NONE', #21204, #2468, #21178, .T. ) ;
#21990=LINE ( 'NONE', #4455, #3616 ) ;
#21994=DIRECTION ( 'NONE',  ( 0.000000000000000000, -1.000000000000000000, 0.000000000000000000 ) ) ;
#22000=FACE_OUTER_BOUND ( 'NONE', #11665, .T. ) ;
#22002=DIRECTION ( 'NONE',  ( 0.4528218681381900867, -0.8916010070293997058, 0.000000000000000000 ) ) ;
#22006=EDGE_CURVE ( 'NONE', #23905, #27805, #8114, .T. ) ;
#22007=EDGE_CURVE ( 'NONE', #4103, #5352, #19164, .T. ) ;
#22009=LINE ( 'NONE', #9083, #5193 ) ;
#22018=EDGE_LOOP ( 'NONE', ( #24963, #23000, #12492, #13666 ) ) ;
#22019=EDGE_CURVE ( 'NONE', #749, #20032, #10410, .T. ) ;
#22022=DIRECTION ( 'NONE',  ( -0.8916010070294598799, 0.4528218681380715149, 0.000000000000000000 ) ) ;
#22024=ORIENTED_EDGE ( 'NONE', *, *, #6109, .T. ) ;
#22025=EDGE_CURVE ( 'NONE', #6585, #23830, #17153, .T. ) ;
#22033=LINE ( 'NONE', #8962, #17817 ) ;
#22036=PLANE ( 'NONE',  #8222 ) ;
#22037=ORIENTED_EDGE ( 'NONE', *, *, #10845, .T. ) ;
#22045=DIRECTION ( 'NONE',  ( 0.8916010070295511403, -0.4528218681378915478, 0.000000000000000000 ) ) ;
#22046=CARTESIAN_POINT ( 'NONE',  ( 158.0000000000010232, 106.1456246621830957, 45.00000000000000000 ) ) ;
#22049=CARTESIAN_POINT ( 'NONE',  ( 157.9999999999998010, 233.5393750375350237, 45.00000000000000000 ) ) ;
#22051=ADVANCED_FACE ( 'NONE', ( #23620 ), #19308, .F. ) ;
#22054=LINE ( 'NONE', #13305, #138 ) ;
#22055=ORIENTED_EDGE ( 'NONE', *, *, #9290, .F. ) ;
#22056=LINE ( 'NONE', #17602, #733 ) ;
#22059=DIRECTION ( 'NONE',  ( -0.000000000000000000, -0.000000000000000000, -1.000000000000000000 ) ) ;
#22068=EDGE_CURVE ( 'NONE', #26043, #19122, #1500, .T. ) ;
#22071=CARTESIAN_POINT ( 'NONE',  ( 158.0000000000011937, 93.09837461714084839, 45.00000000000000000 ) ) ;
#22073=CARTESIAN_POINT ( 'NONE',  ( 158.0000000000006537, 141.2558747672816821, 45.00000000000000000 ) ) ;
#22078=CARTESIAN_POINT ( 'NONE',  ( 167.4999999999996589, 258.6181251126050711, 1.387778780781445676E-14 ) ) ;
#22080=EDGE_LOOP ( 'NONE', ( #20148, #20500, #3255, #22552 ) ) ;
#22082=VECTOR ( 'NONE', #4867, 1000.000000000000000 ) ;
#22084=CARTESIAN_POINT ( 'NONE',  ( 157.4999999999998579, 143.5098122710352015, 45.00000000000000000 ) ) ;
#22086=EDGE_LOOP ( 'NONE', ( #20115, #11877, #2882, #14336 ) ) ;
#22089=DIRECTION ( 'NONE',  ( 0.4528218681373308296, -0.8916010070298360235, 0.000000000000000000 ) ) ;
#22090=ORIENTED_EDGE ( 'NONE', *, *, #21790, .F. ) ;
#22092=AXIS2_PLACEMENT_3D ( 'NONE', #17336, #5997, #1823 ) ;
#22093=ORIENTED_EDGE ( 'NONE', *, *, #6027, .T. ) ;
#22095=VECTOR ( 'NONE', #6222, 999.9999999999998863 ) ;
#22096=ORIENTED_EDGE ( 'NONE', *, *, #18841, .F. ) ;
#22102=EDGE_CURVE ( 'NONE', #26043, #17587, #19452, .T. ) ;
#22107=DIRECTION ( 'NONE',  ( -0.8916010070299166257, 0.4528218681371722343, 0.000000000000000000 ) ) ;
#22110=DIRECTION ( 'NONE',  ( -0.000000000000000000, -0.000000000000000000, -1.000000000000000000 ) ) ;
#22112=VECTOR ( 'NONE', #27468, 1000.000000000000000 ) ;
#22117=VECTOR ( 'NONE', #25159, 1000.000000000000000 ) ;
#22118=ORIENTED_EDGE ( 'NONE', *, *, #1605, .F. ) ;
#22129=ORIENTED_EDGE ( 'NONE', *, *, #26195, .T. ) ;
#22130=VECTOR ( 'NONE', #18609, 1000.000000000000227 ) ;
#22134=CARTESIAN_POINT ( 'NONE',  ( 158.0000000000009095, 120.6849996997183183, -45.00000000000000000 ) ) ;
#22138=DIRECTION ( 'NONE',  ( -0.000000000000000000, 0.000000000000000000, -1.000000000000000000 ) ) ;
#22141=DIRECTION ( 'NONE',  ( -0.000000000000000000, 1.000000000000000000, -0.000000000000000000 ) ) ;
#22143=VERTEX_POINT ( 'NONE', #17715 ) ;
#22148=EDGE_LOOP ( 'NONE', ( #8392, #27773, #17043, #3188 ) ) ;
#22154=LINE ( 'NONE', #4616, #23163 ) ;
#22160=LINE ( 'NONE', #19719, #14787 ) ;
#22163=VECTOR ( 'NONE', #4925, 1000.000000000000000 ) ;
#22166=PLANE ( 'NONE',  #21723 ) ;
#22173=EDGE_CURVE ( 'NONE', #6438, #12064, #6658, .T. ) ;
#22175=DIRECTION ( 'NONE',  ( -0.8916010070297548662, -0.4528218681374907573, 0.000000000000000000 ) ) ;
#22176=FACE_OUTER_BOUND ( 'NONE', #16202, .T. ) ;
#22178=DIRECTION ( 'NONE',  ( 0.4528218681372309096, -0.8916010070298868717, 0.000000000000000000 ) ) ;
#22179=CARTESIAN_POINT ( 'NONE',  ( 157.9999999999996874, 269.1575001501400379, 45.00000000000000000 ) ) ;
#22182=CARTESIAN_POINT ( 'NONE',  ( 158.0000000000015064, 61.00387452705632541, -45.00000000000000000 ) ) ;
#22183=LINE ( 'NONE', #22328, #11102 ) ;
#22184=FACE_OUTER_BOUND ( 'NONE', #14401, .T. ) ;
#22188=CARTESIAN_POINT ( 'NONE',  ( 157.4999999999998579, 181.1279373836408411, 45.00000000000000000 ) ) ;
#22191=CARTESIAN_POINT ( 'NONE',  ( 157.4999999999998579, 171.0964373536126573, 45.00000000000000000 ) ) ;
#22192=LINE ( 'NONE', #16027, #15161 ) ;
#22194=ORIENTED_EDGE ( 'NONE', *, *, #16085, .T. ) ;
#22195=CARTESIAN_POINT ( 'NONE',  ( 157.4999999999998579, 80.81293708335913095, 45.00000000000000000 ) ) ;
#22196=EDGE_LOOP ( 'NONE', ( #10995, #8975, #15355, #12362 ) ) ;
#22197=VECTOR ( 'NONE', #17435, 1000.000000000000000 ) ;
#22198=EDGE_CURVE ( 'NONE', #5015, #21239, #6793, .T. ) ;
#22199=CARTESIAN_POINT ( 'NONE',  ( 157.4999999999998579, 58.24206201579573872, 45.00000000000000000 ) ) ;
#22202=ORIENTED_EDGE ( 'NONE', *, *, #3175, .T. ) ;
#22205=EDGE_LOOP ( 'NONE', ( #15065, #2760, #15170, #3462 ) ) ;
#22206=FACE_OUTER_BOUND ( 'NONE', #6639, .T. ) ;
#22207=ORIENTED_EDGE ( 'NONE', *, *, #11473, .T. ) ;
#22209=VERTEX_POINT ( 'NONE', #13565 ) ;
#22211=LINE ( 'NONE', #12898, #26585 ) ;
#22212=DIRECTION ( 'NONE',  ( -0.000000000000000000, -0.000000000000000000, -1.000000000000000000 ) ) ;
#22215=LINE ( 'NONE', #13185, #28198 ) ;
#22217=FACE_OUTER_BOUND ( 'NONE', #12821, .T. ) ;
#22218=LINE ( 'NONE', #2523, #13108 ) ;
#22222=DIRECTION ( 'NONE',  ( 0.8916010070295820045, -0.4528218681378310406, 0.000000000000000000 ) ) ;
#22224=DIRECTION ( 'NONE',  ( -0.000000000000000000, -0.000000000000000000, -1.000000000000000000 ) ) ;
#22226=CARTESIAN_POINT ( 'NONE',  ( 157.4999999999996589, 278.9350626764145318, 45.00000000000000000 ) ) ;
#22227=FACE_OUTER_BOUND ( 'NONE', #20651, .T. ) ;
#22229=EDGE_LOOP ( 'NONE', ( #4733, #24682, #7841, #20750 ) ) ;
#22230=ADVANCED_FACE ( 'NONE', ( #18154 ), #27185, .F. ) ;
#22231=FACE_OUTER_BOUND ( 'NONE', #2606, .T. ) ;
#22232=VERTEX_POINT ( 'NONE', #14132 ) ;
#22234=ORIENTED_EDGE ( 'NONE', *, *, #2482, .T. ) ;
#22237=VERTEX_POINT ( 'NONE', #26909 ) ;
#22238=VERTEX_POINT ( 'NONE', #27453 ) ;
#22240=ORIENTED_EDGE ( 'NONE', *, *, #10209, .F. ) ;
#22242=CARTESIAN_POINT ( 'NONE',  ( 158.0000000000006253, 148.2716247822957882, 45.00000000000000000 ) ) ;
#22244=FACE_OUTER_BOUND ( 'NONE', #6264, .T. ) ;
#22248=FACE_OUTER_BOUND ( 'NONE', #13345, .T. ) ;
#22249=ADVANCED_FACE ( 'NONE', ( #11839 ), #16007, .F. ) ;
#22250=DIRECTION ( 'NONE',  ( 0.8916010070296327417, -0.4528218681377311761, 0.000000000000000000 ) ) ;
#22251=CARTESIAN_POINT ( 'NONE',  ( 157.4999999999998579, 75.79718706834503905, 45.00000000000000000 ) ) ;
#22255=VECTOR ( 'NONE', #16534, 999.9999999999998863 ) ;
#22260=CARTESIAN_POINT ( 'NONE',  ( 157.9999999999998295, 229.0315000300280417, 45.00000000000000000 ) ) ;
#22261=VECTOR ( 'NONE', #6217, 1000.000000000000000 ) ;
#22262=ORIENTED_EDGE ( 'NONE', *, *, #22717, .T. ) ;
#22264=PLANE ( 'NONE',  #12838 ) ;
#22267=LINE ( 'NONE', #20105, #1490 ) ;
#22271=VERTEX_POINT ( 'NONE', #18433 ) ;
#22272=ORIENTED_EDGE ( 'NONE', *, *, #10019, .T. ) ;
#22273=CARTESIAN_POINT ( 'NONE',  ( 157.9999999999998010, 231.5393750375350237, -45.00000000000000000 ) ) ;
#22276=EDGE_LOOP ( 'NONE', ( #11689, #4089, #27522, #14794 ) ) ;
#22281=ORIENTED_EDGE ( 'NONE', *, *, #19596, .T. ) ;
#22286=CARTESIAN_POINT ( 'NONE',  ( 157.4999999999998579, 110.9074371734436255, 45.00000000000000000 ) ) ;
#22288=EDGE_CURVE ( 'NONE', #17959, #15548, #14001, .T. ) ;
#22289=EDGE_CURVE ( 'NONE', #21270, #6129, #16425, .T. ) ;
#22290=VERTEX_POINT ( 'NONE', #25314 ) ;
#22297=VECTOR ( 'NONE', #23193, 1000.000000000000000 ) ;
#22298=PLANE ( 'NONE',  #11474 ) ;
#22299=EDGE_CURVE ( 'NONE', #23503, #7481, #20865, .T. ) ;
#22304=AXIS2_PLACEMENT_3D ( 'NONE', #14555, #12547, #3757 ) ;
#22311=CARTESIAN_POINT ( 'NONE',  ( 158.0000000000004547, 165.8267498348450886, -45.00000000000000000 ) ) ;
#22312=CARTESIAN_POINT ( 'NONE',  ( 157.4999999999998579, 193.6673124211760353, 45.00000000000000000 ) ) ;
#22313=ORIENTED_EDGE ( 'NONE', *, *, #22789, .T. ) ;
#22314=CARTESIAN_POINT ( 'NONE',  ( 157.4999999999996589, 281.4429376839215138, -45.00000000000000000 ) ) ;
#22315=ORIENTED_EDGE ( 'NONE', *, *, #10353, .F. ) ;
#22318=CARTESIAN_POINT ( 'NONE',  ( 158.0000000000013642, 78.05112457209858690, -45.00000000000000000 ) ) ;
#22319=CARTESIAN_POINT ( 'NONE',  ( 158.0000000000010516, 103.6377496546760568, 45.00000000000000000 ) ) ;
#22325=EDGE_CURVE ( 'NONE', #15954, #14251, #14410, .T. ) ;
#22326=ORIENTED_EDGE ( 'NONE', *, *, #3642, .T. ) ;
#22328=CARTESIAN_POINT ( 'NONE',  ( 157.4999999999998579, 78.30506207585207790, 45.00000000000000000 ) ) ;
#22334=CARTESIAN_POINT ( 'NONE',  ( 187.4999999999996305, 288.9665627064425166, 45.00000000000000000 ) ) ;
#22337=ORIENTED_EDGE ( 'NONE', *, *, #16066, .F. ) ;
#22338=DIRECTION ( 'NONE',  ( -0.000000000000000000, -0.000000000000000000, -1.000000000000000000 ) ) ;
#22345=EDGE_CURVE ( 'NONE', #17770, #19699, #20719, .T. ) ;
#22347=ORIENTED_EDGE ( 'NONE', *, *, #27910, .T. ) ;
#22348=ORIENTED_EDGE ( 'NONE', *, *, #12318, .T. ) ;
#22350=VERTEX_POINT ( 'NONE', #5212 ) ;
#22352=ORIENTED_EDGE ( 'NONE', *, *, #19113, .T. ) ;
#22361=CARTESIAN_POINT ( 'NONE',  ( 157.4999999999998579, 141.0019372635281627, 45.00000000000000000 ) ) ;
#22363=DIRECTION ( 'NONE',  ( 0.000000000000000000, 0.000000000000000000, -1.000000000000000000 ) ) ;
#22364=CARTESIAN_POINT ( 'NONE',  ( 158.0000000000005116, 160.8109998198309825, -45.00000000000000000 ) ) ;
#22368=ORIENTED_EDGE ( 'NONE', *, *, #25003, .F. ) ;
#22370=PLANE ( 'NONE',  #16516 ) ;
#22372=DIRECTION ( 'NONE',  ( 0.4528218681375507093, -0.8916010070297244461, 0.000000000000000000 ) ) ;
#22374=VECTOR ( 'NONE', #22430, 1000.000000000000114 ) ;
#22375=EDGE_CURVE ( 'NONE', #2585, #23830, #7932, .T. ) ;
#22382=VERTEX_POINT ( 'NONE', #8362 ) ;
#22384=CARTESIAN_POINT ( 'NONE',  ( 157.4999999999998579, 120.9389372034718093, -45.00000000000000000 ) ) ;
#22385=FACE_OUTER_BOUND ( 'NONE', #1106, .T. ) ;
#22386=CARTESIAN_POINT ( 'NONE',  ( 157.4999999999998579, 176.1121873686267350, 45.00000000000000000 ) ) ;
#22392=VECTOR ( 'NONE', #13083, 1000.000000000000227 ) ;
#22393=CARTESIAN_POINT ( 'NONE',  ( 158.0000000000010800, 103.1298746471690038, 45.00000000000000000 ) ) ;
#22397=DIRECTION ( 'NONE',  ( 0.4528218681382713551, -0.8916010070293584056, 0.000000000000000000 ) ) ;
#22404=DIRECTION ( 'NONE',  ( -0.000000000000000000, -0.000000000000000000, -1.000000000000000000 ) ) ;
#22406=VERTEX_POINT ( 'NONE', #10374 ) ;
#22411=ORIENTED_EDGE ( 'NONE', *, *, #11275, .T. ) ;
#22412=ORIENTED_EDGE ( 'NONE', *, *, #5312, .T. ) ;
#22414=VECTOR ( 'NONE', #818, 1000.000000000000114 ) ;
#22416=CARTESIAN_POINT ( 'NONE',  ( 157.4999999999998010, 238.8090625563025071, 45.00000000000000000 ) ) ;
#22420=CARTESIAN_POINT ( 'NONE',  ( 158.0000000000016769, 47.95662448201407102, -45.00000000000000000 ) ) ;
#22422=ORIENTED_EDGE ( 'NONE', *, *, #2763, .T. ) ;
#22425=CARTESIAN_POINT ( 'NONE',  ( 157.4999999999998579, 138.4940622560211239, 45.00000000000000000 ) ) ;
#22430=DIRECTION ( 'NONE',  ( -0.8916010070293409751, -0.4528218681383056610, 0.000000000000000000 ) ) ;
#22434=LINE ( 'NONE', #2743, #19676 ) ;
#22437=DIRECTION ( 'NONE',  ( 0.8916010070296531698, -0.4528218681376911525, 0.000000000000000000 ) ) ;
#22442=LINE ( 'NONE', #2609, #15861 ) ;
#22443=ORIENTED_EDGE ( 'NONE', *, *, #7483, .T. ) ;
#22444=SHAPE_REPRESENTATION_RELATIONSHIP ( 'NONE' , 'NONE' ,  #10277, #27021 ) ;
#22447=AXIS2_PLACEMENT_3D ( 'NONE', #8830, #19887, #11283 ) ;
#22451=VERTEX_POINT ( 'NONE', #25876 ) ;
#22452=CARTESIAN_POINT ( 'NONE',  ( 157.9999999999997726, 243.5708750675630370, 45.00000000000000000 ) ) ;
#22455=DIRECTION ( 'NONE',  ( 0.4528218681375707488, -0.8916010070297142320, 0.000000000000000000 ) ) ;
#22456=ORIENTED_EDGE ( 'NONE', *, *, #13077, .T. ) ;
#22457=DIRECTION ( 'NONE',  ( 0.4528218681374108767, -0.8916010070297955004, 0.000000000000000000 ) ) ;
#22463=LINE ( 'NONE', #11414, #5293 ) ;
#22470=VECTOR ( 'NONE', #13261, 1000.000000000000000 ) ;
#22473=CARTESIAN_POINT ( 'NONE',  ( 157.4999999999998579, 151.0334372935563465, -45.00000000000000000 ) ) ;
#22474=LINE ( 'NONE', #4644, #1101 ) ;
#22478=ORIENTED_EDGE ( 'NONE', *, *, #15495, .F. ) ;
#22486=LINE ( 'NONE', #931, #7492 ) ;
#22488=CARTESIAN_POINT ( 'NONE',  ( 157.9999999999998295, 226.5236250225210313, 45.00000000000000000 ) ) ;
#22491=ORIENTED_EDGE ( 'NONE', *, *, #21986, .F. ) ;
#22492=DIRECTION ( 'NONE',  ( -0.000000000000000000, -0.000000000000000000, -1.000000000000000000 ) ) ;
#22496=VERTEX_POINT ( 'NONE', #19130 ) ;
#22500=AXIS2_PLACEMENT_3D ( 'NONE', #16532, #19100, #14653 ) ;
#22502=VECTOR ( 'NONE', #10244, 1000.000000000000114 ) ;
#22504=LINE ( 'NONE', #16190, #26149 ) ;
#22505=LINE ( 'NONE', #25081, #16543 ) ;
#22507=DIRECTION ( 'NONE',  ( -0.000000000000000000, 0.000000000000000000, -1.000000000000000000 ) ) ;
#22508=EDGE_CURVE ( 'NONE', #8798, #4392, #8645, .T. ) ;
#22512=LINE ( 'NONE', #19920, #21482 ) ;
#22513=LINE ( 'NONE', #26819, #23091 ) ;
#22519=FACE_OUTER_BOUND ( 'NONE', #2458, .T. ) ;
#22521=EDGE_CURVE ( 'NONE', #24784, #27410, #2165, .T. ) ;
#22522=AXIS2_PLACEMENT_3D ( 'NONE', #28381, #19778, #2529 ) ;
#22527=EDGE_CURVE ( 'NONE', #17008, #23616, #455, .T. ) ;
#22528=ORIENTED_EDGE ( 'NONE', *, *, #28105, .F. ) ;
#22530=ORIENTED_EDGE ( 'NONE', *, *, #26592, .F. ) ;
#22532=LINE ( 'NONE', #16080, #4007 ) ;
#22535=CARTESIAN_POINT ( 'NONE',  ( 158.0000000000002842, 178.8739998798873216, 45.00000000000000000 ) ) ;
#22537=AXIS2_PLACEMENT_3D ( 'NONE', #5329, #27161, #7497 ) ;
#22549=CARTESIAN_POINT ( 'NONE',  ( 157.4999999999998579, 58.24206201579573872, 45.00000000000000000 ) ) ;
#22550=CARTESIAN_POINT ( 'NONE',  ( 157.9999999999998579, 221.5078750075070104, 45.00000000000000000 ) ) ;
#22552=ORIENTED_EDGE ( 'NONE', *, *, #9140, .T. ) ;
#22555=VECTOR ( 'NONE', #4968, 1000.000000000000114 ) ;
#22556=PLANE ( 'NONE',  #27179 ) ;
#22559=VECTOR ( 'NONE', #21020, 999.9999999999998863 ) ;
#22560=ORIENTED_EDGE ( 'NONE', *, *, #2518, .F. ) ;
#22561=EDGE_CURVE ( 'NONE', #5556, #13208, #9215, .T. ) ;
#22562=AXIS2_PLACEMENT_3D ( 'NONE', #16927, #25682, #8595 ) ;
#22567=EDGE_LOOP ( 'NONE', ( #577, #22779, #1983, #14668 ) ) ;
#22568=PLANE ( 'NONE',  #23396 ) ;
#22569=PLANE ( 'NONE',  #7684 ) ;
#22573=DIRECTION ( 'NONE',  ( 0.8916010070294800860, -0.4528218681380314359, 0.000000000000000000 ) ) ;
#22575=CARTESIAN_POINT ( 'NONE',  ( 158.0000000000013927, 73.54324956459154805, 45.00000000000000000 ) ) ;
#22577=FACE_OUTER_BOUND ( 'NONE', #16378, .T. ) ;
#22578=PRODUCT_DEFINITION_FORMATION_WITH_SPECIFIED_SOURCE ( 'ANY', '', #19210, .NOT_KNOWN. ) ;
#22583=LINE ( 'NONE', #11681, #6074 ) ;
#22584=CARTESIAN_POINT ( 'NONE',  ( 158.0000000000005116, 160.8109998198309825, 45.00000000000000000 ) ) ;
#22588=CARTESIAN_POINT ( 'NONE',  ( 157.9999999999996589, 273.6653751576470768, -45.00000000000000000 ) ) ;
#22591=ORIENTED_EDGE ( 'NONE', *, *, #14915, .T. ) ;
#22593=ADVANCED_FACE ( 'NONE', ( #17400 ), #12968, .F. ) ;
#22594=VECTOR ( 'NONE', #18684, 1000.000000000000000 ) ;
#22595=DIRECTION ( 'NONE',  ( -0.000000000000000000, -0.000000000000000000, -1.000000000000000000 ) ) ;
#22597=ORIENTED_EDGE ( 'NONE', *, *, #22962, .F. ) ;
#22601=PLANE ( 'NONE',  #16683 ) ;
#22603=ORIENTED_EDGE ( 'NONE', *, *, #10266, .F. ) ;
#22604=CARTESIAN_POINT ( 'NONE',  ( 158.0000000000012506, 88.08262460212675649, -45.00000000000000000 ) ) ;
#22605=ORIENTED_EDGE ( 'NONE', *, *, #24300, .T. ) ;
#22608=LINE ( 'NONE', #14002, #21823 ) ;
#22609=VECTOR ( 'NONE', #20089, 1000.000000000000000 ) ;
#22619=DIRECTION ( 'NONE',  ( 0.4528218681373921140, 0.8916010070298049373, -0.000000000000000000 ) ) ;
#22622=FACE_OUTER_BOUND ( 'NONE', #18285, .T. ) ;
#22627=ORIENTED_EDGE ( 'NONE', *, *, #9227, .F. ) ;
#22633=EDGE_CURVE ( 'NONE', #13806, #20506, #6762, .T. ) ;
#22637=ORIENTED_EDGE ( 'NONE', *, *, #1533, .T. ) ;
#22638=EDGE_CURVE ( 'NONE', #26868, #2799, #26730, .T. ) ;
#22642=ORIENTED_EDGE ( 'NONE', *, *, #5592, .T. ) ;
#22643=DIRECTION ( 'NONE',  ( -0.8916010070299070778, -0.4528218681371909971, 0.000000000000000000 ) ) ;
#22648=DIRECTION ( 'NONE',  ( 0.4528218681372110921, -0.8916010070298969747, 0.000000000000000000 ) ) ;
#22649=DIRECTION ( 'NONE',  ( -0.000000000000000000, -0.000000000000000000, -1.000000000000000000 ) ) ;
#22650=DIRECTION ( 'NONE',  ( 0.000000000000000000, -1.000000000000000000, 0.000000000000000000 ) ) ;
#22651=DIRECTION ( 'NONE',  ( 0.000000000000000000, -1.000000000000000000, 0.000000000000000000 ) ) ;
#22653=DIRECTION ( 'NONE',  ( 0.4528218681383106015, 0.8916010070293384215, -0.000000000000000000 ) ) ;
#22655=CARTESIAN_POINT ( 'NONE',  ( 158.0000000000010232, 108.1456246621830957, 45.00000000000000000 ) ) ;
#22657=CARTESIAN_POINT ( 'NONE',  ( 157.9999999999996874, 268.6496251426330559, 45.00000000000000000 ) ) ;
#22661=EDGE_CURVE ( 'NONE', #23530, #3711, #15406, .T. ) ;
#22662=EDGE_CURVE ( 'NONE', #2950, #28150, #24583, .T. ) ;
#22664=PLANE ( 'NONE',  #23393 ) ;
#22665=PLANE ( 'NONE',  #1138 ) ;
#22669=CARTESIAN_POINT ( 'NONE',  ( 158.0000000000016769, 47.95662448201407102, 45.00000000000000000 ) ) ;
#22670=ORIENTED_EDGE ( 'NONE', *, *, #18993, .F. ) ;
#22672=CARTESIAN_POINT ( 'NONE',  ( 158.0000000000000853, 196.4291249324366504, 45.00000000000000000 ) ) ;
#22674=ADVANCED_FACE ( 'NONE', ( #12087 ), #7627, .F. ) ;
#22676=ORIENTED_EDGE ( 'NONE', *, *, #4979, .F. ) ;
#22677=VERTEX_POINT ( 'NONE', #26880 ) ;
#22678=CARTESIAN_POINT ( 'NONE',  ( 157.9999999999996874, 266.1417501351260171, 45.00000000000000000 ) ) ;
#22680=DIRECTION ( 'NONE',  ( -0.000000000000000000, -0.000000000000000000, -1.000000000000000000 ) ) ;
#22681=DIRECTION ( 'NONE',  ( -0.000000000000000000, -0.000000000000000000, -1.000000000000000000 ) ) ;
#22687=CARTESIAN_POINT ( 'NONE',  ( 157.4999999999998579, 223.7618125112605298, 45.00000000000000000 ) ) ;
#22689=PLANE ( 'NONE',  #21325 ) ;
#22690=CARTESIAN_POINT ( 'NONE',  ( 157.4999999999998579, 110.9074371734436255, -45.00000000000000000 ) ) ;
#22694=LINE ( 'NONE', #11925, #10068 ) ;
#22696=DIRECTION ( 'NONE',  ( -0.8916010070296531698, -0.4528218681376911525, 0.000000000000000000 ) ) ;
#22698=ORIENTED_EDGE ( 'NONE', *, *, #16955, .F. ) ;
#22702=EDGE_LOOP ( 'NONE', ( #2223, #26314, #6902, #17967 ) ) ;
#22704=ORIENTED_EDGE ( 'NONE', *, *, #25436, .F. ) ;
#22705=EDGE_CURVE ( 'NONE', #6158, #12778, #18541, .T. ) ;
#22706=PLANE ( 'NONE',  #7901 ) ;
#22707=EDGE_CURVE ( 'NONE', #8565, #12700, #20409, .T. ) ;
#22709=VERTEX_POINT ( 'NONE', #1005 ) ;
#22710=EDGE_LOOP ( 'NONE', ( #11659, #3098, #12780, #4018 ) ) ;
#22715=CARTESIAN_POINT ( 'NONE',  ( 157.9999999999998295, 231.0315000300280417, -45.00000000000000000 ) ) ;
#22716=EDGE_CURVE ( 'NONE', #21766, #6126, #7204, .T. ) ;
#22717=EDGE_CURVE ( 'NONE', #6126, #3644, #20267, .T. ) ;
#22719=AXIS2_PLACEMENT_3D ( 'NONE', #4237, #28349, #8697 ) ;
#22724=CARTESIAN_POINT ( 'NONE',  ( 157.4999999999998295, 218.7460624962465090, -45.00000000000000000 ) ) ;
#22725=CARTESIAN_POINT ( 'NONE',  ( 157.4999999999998579, 161.0649373235845019, -45.00000000000000000 ) ) ;
#22726=CARTESIAN_POINT ( 'NONE',  ( 158.0000000000001990, 188.3976249024084666, -45.00000000000000000 ) ) ;
#22730=DIRECTION ( 'NONE',  ( -0.000000000000000000, -0.000000000000000000, -1.000000000000000000 ) ) ;
#22731=EDGE_LOOP ( 'NONE', ( #13233, #8832, #6934, #10849 ) ) ;
#22732=VECTOR ( 'NONE', #14553, 1000.000000000000000 ) ;
#22735=LINE ( 'NONE', #27033, #1461 ) ;
#22743=CARTESIAN_POINT ( 'NONE',  ( 157.4999999999998579, 48.21056198576756202, 45.00000000000000000 ) ) ;
#22744=VERTEX_POINT ( 'NONE', #18263 ) ;
#22752=VECTOR ( 'NONE', #16333, 1000.000000000000000 ) ;
#22761=EDGE_CURVE ( 'NONE', #3887, #22709, #1151, .T. ) ;
#22762=VECTOR ( 'NONE', #22250, 1000.000000000000114 ) ;
#22767=ORIENTED_EDGE ( 'NONE', *, *, #25944, .T. ) ;
#22769=CARTESIAN_POINT ( 'NONE',  ( 157.4999999999996589, 273.9193126614005678, -45.00000000000000000 ) ) ;
#22770=LINE ( 'NONE', #927, #21793 ) ;
#22771=ORIENTED_EDGE ( 'NONE', *, *, #17804, .F. ) ;
#22772=LINE ( 'NONE', #2648, #3729 ) ;
#22778=VECTOR ( 'NONE', #24081, 1000.000000000000227 ) ;
#22779=ORIENTED_EDGE ( 'NONE', *, *, #3351, .F. ) ;
#22781=ORIENTED_EDGE ( 'NONE', *, *, #11239, .T. ) ;
#22785=PLANE ( 'NONE',  #27171 ) ;
#22788=CARTESIAN_POINT ( 'NONE',  ( 158.0000000000017053, 43.44874947450702507, 45.00000000000000000 ) ) ;
#22789=EDGE_CURVE ( 'NONE', #4657, #3701, #1290, .T. ) ;
#22794=EDGE_CURVE ( 'NONE', #12610, #27327, #27559, .T. ) ;
#22795=CARTESIAN_POINT ( 'NONE',  ( 157.9999999999996874, 266.6496251426330559, -45.00000000000000000 ) ) ;
#22796=FACE_OUTER_BOUND ( 'NONE', #3422, .T. ) ;
#22803=PLANE ( 'NONE',  #12621 ) ;
#22804=PLANE ( 'NONE',  #12031 ) ;
#22809=CARTESIAN_POINT ( 'NONE',  ( 157.4999999999995168, 208.7145624662163925, 45.00000000000000000 ) ) ;
#22812=ORIENTED_EDGE ( 'NONE', *, *, #2225, .T. ) ;
#22814=CARTESIAN_POINT ( 'NONE',  ( 158.0000000000017053, 45.44874947450702507, -45.00000000000000000 ) ) ;
#22815=VECTOR ( 'NONE', #16419, 1000.000000000000000 ) ;
#22819=EDGE_CURVE ( 'NONE', #10398, #548, #23408, .T. ) ;
#22826=ADVANCED_FACE ( 'NONE', ( #10480 ), #20969, .F. ) ;
#22829=PLANE ( 'NONE',  #23923 ) ;
#22832=LINE ( 'NONE', #5301, #9146 ) ;
#22837=VECTOR ( 'NONE', #15797, 1000.000000000000227 ) ;
#22843=ORIENTED_EDGE ( 'NONE', *, *, #27306, .T. ) ;
#22844=LINE ( 'NONE', #5451, #25240 ) ;
#22845=CARTESIAN_POINT ( 'NONE',  ( 157.4999999999998295, 226.2696875187675118, 45.00000000000000000 ) ) ;
#22851=DIRECTION ( 'NONE',  ( 0.5150380749100565980, 0.000000000000000000, -0.8571673007021108903 ) ) ;
#22856=CARTESIAN_POINT ( 'NONE',  ( 157.9999999999998010, 234.0472500450420341, 45.00000000000000000 ) ) ;
#22865=DIRECTION ( 'NONE',  ( -0.8916010070295614653, 0.4528218681378716193, 0.000000000000000000 ) ) ;
#22869=EDGE_CURVE ( 'NONE', #17461, #4617, #12789, .T. ) ;
#22874=LINE ( 'NONE', #20573, #17303 ) ;
#22875=ADVANCED_FACE ( 'NONE', ( #21395 ), #10059, .F. ) ;
#22876=CARTESIAN_POINT ( 'NONE',  ( 157.4999999999998579, 125.9546872184859012, -45.00000000000000000 ) ) ;
#22882=AXIS2_PLACEMENT_3D ( 'NONE', #24774, #9548, #5081 ) ;
#22887=LINE ( 'NONE', #27323, #20987 ) ;
#22888=VECTOR ( 'NONE', #28297, 1000.000000000000114 ) ;
#22891=DIRECTION ( 'NONE',  ( -0.000000000000000000, -0.000000000000000000, -1.000000000000000000 ) ) ;
#22893=EDGE_CURVE ( 'NONE', #1534, #4885, #27420, .T. ) ;
#22896=DIRECTION ( 'NONE',  ( -0.8916010070293384215, 0.4528218681383106015, 0.000000000000000000 ) ) ;
#22897=ORIENTED_EDGE ( 'NONE', *, *, #13406, .T. ) ;
#22900=VECTOR ( 'NONE', #20882, 1000.000000000000114 ) ;
#22902=LINE ( 'NONE', #18729, #14704 ) ;
#22909=VECTOR ( 'NONE', #25823, 999.9999999999998863 ) ;
#22913=EDGE_CURVE ( 'NONE', #25491, #23391, #19665, .T. ) ;
#22921=ORIENTED_EDGE ( 'NONE', *, *, #25473, .F. ) ;
#22923=VECTOR ( 'NONE', #857, 1000.000000000000000 ) ;
#22924=LINE ( 'NONE', #20198, #15854 ) ;
#22929=DIRECTION ( 'NONE',  ( -0.000000000000000000, 0.000000000000000000, -1.000000000000000000 ) ) ;
#22930=CARTESIAN_POINT ( 'NONE',  ( 157.9999999999996874, 269.1575001501400379, 45.00000000000000000 ) ) ;
#22933=PLANE ( 'NONE',  #3610 ) ;
#22935=ORIENTED_EDGE ( 'NONE', *, *, #26446, .F. ) ;
#22936=AXIS2_PLACEMENT_3D ( 'NONE', #13934, #16361, #11635 ) ;
#22942=LINE ( 'NONE', #20782, #11627 ) ;
#22945=VECTOR ( 'NONE', #2705, 999.9999999999998863 ) ;
#22946=EDGE_CURVE ( 'NONE', #12922, #8771, #4710, .T. ) ;
#22948=EDGE_CURVE ( 'NONE', #22744, #4103, #19528, .T. ) ;
#22950=ORIENTED_EDGE ( 'NONE', *, *, #17597, .F. ) ;
#22959=LINE ( 'NONE', #24977, #21486 ) ;
#22961=VECTOR ( 'NONE', #26506, 1000.000000000000000 ) ;
#22962=EDGE_CURVE ( 'NONE', #9868, #548, #15372, .T. ) ;
#22963=DIRECTION ( 'NONE',  ( -0.000000000000000000, -0.000000000000000000, -1.000000000000000000 ) ) ;
#22973=CARTESIAN_POINT ( 'NONE',  ( 158.0000000000003695, 171.3503748573662051, 45.00000000000000000 ) ) ;
#22977=ORIENTED_EDGE ( 'NONE', *, *, #21294, .T. ) ;
#22980=ORIENTED_EDGE ( 'NONE', *, *, #27367, .F. ) ;
#22981=EDGE_CURVE ( 'NONE', #2545, #6857, #11193, .T. ) ;
#22982=VECTOR ( 'NONE', #2709, 1000.000000000000227 ) ;
#22983=ADVANCED_FACE ( 'NONE', ( #26404 ), #13353, .F. ) ;
#22984=ORIENTED_EDGE ( 'NONE', *, *, #18472, .F. ) ;
#22988=VECTOR ( 'NONE', #27429, 1000.000000000000000 ) ;
#22989=LINE ( 'NONE', #2881, #1796 ) ;
#22991=DIRECTION ( 'NONE',  ( -0.000000000000000000, -0.000000000000000000, -1.000000000000000000 ) ) ;
#22995=VECTOR ( 'NONE', #24231, 1000.000000000000000 ) ;
#22999=DIRECTION ( 'NONE',  ( 0.4528218681383056610, -0.8916010070293409751, 0.000000000000000000 ) ) ;
#23000=ORIENTED_EDGE ( 'NONE', *, *, #3251, .F. ) ;
#23006=ORIENTED_EDGE ( 'NONE', *, *, #26151, .F. ) ;
#23008=DIRECTION ( 'NONE',  ( -0.8916010070294503320, -0.4528218681380901667, 0.000000000000000000 ) ) ;
#23009=EDGE_CURVE ( 'NONE', #695, #20671, #13411, .T. ) ;
#23012=FACE_OUTER_BOUND ( 'NONE', #13444, .T. ) ;
#23016=CARTESIAN_POINT ( 'NONE',  ( 217.4999999999996305, 258.6181251126050711, -5.999999999999991118 ) ) ;
#23021=VECTOR ( 'NONE', #23782, 1000.000000000000000 ) ;
#23022=CARTESIAN_POINT ( 'NONE',  ( 158.0000000000011084, 98.62199963966197913, 45.00000000000000000 ) ) ;
#23026=DIRECTION ( 'NONE',  ( -0.8916010070296632728, -0.4528218681376712240, 0.000000000000000000 ) ) ;
#23029=DIRECTION ( 'NONE',  ( 0.000000000000000000, -1.000000000000000000, 0.000000000000000000 ) ) ;
#23031=ORIENTED_EDGE ( 'NONE', *, *, #24597, .F. ) ;
#23037=CARTESIAN_POINT ( 'NONE',  ( 158.0000000000014211, 73.03537455708450921, -45.00000000000000000 ) ) ;
#23040=VECTOR ( 'NONE', #27853, 1000.000000000000000 ) ;
#23045=PLANE ( 'NONE',  #8339 ) ;
#23047=VECTOR ( 'NONE', #24516, 1000.000000000000114 ) ;
#23052=CARTESIAN_POINT ( 'NONE',  ( 158.0000000000001137, 193.9212499249295831, 45.00000000000000000 ) ) ;
#23054=EDGE_LOOP ( 'NONE', ( #27079, #7011, #3594, #20616 ) ) ;
#23058=EDGE_CURVE ( 'NONE', #16902, #9313, #27120, .T. ) ;
#23059=ORIENTED_EDGE ( 'NONE', *, *, #17154, .F. ) ;
#23062=DIRECTION ( 'NONE',  ( 1.000000000000000000, 0.000000000000000000, -0.000000000000000000 ) ) ;
#23063=VECTOR ( 'NONE', #24069, 1000.000000000000000 ) ;
#23064=DIRECTION ( 'NONE',  ( -0.000000000000000000, -0.000000000000000000, -1.000000000000000000 ) ) ;
#23074=DIRECTION ( 'NONE',  ( 0.000000000000000000, -1.000000000000000000, 0.000000000000000000 ) ) ;
#23075=DIRECTION ( 'NONE',  ( 0.4528218681370311249, -0.8916010070299883461, 0.000000000000000000 ) ) ;
#23079=CARTESIAN_POINT ( 'NONE',  ( 157.9999999999997158, 258.6181251126050711, -45.00000000000000000 ) ) ;
#23081=EDGE_CURVE ( 'NONE', #3367, #8626, #20230, .T. ) ;
#23087=LINE ( 'NONE', #3392, #8853 ) ;
#23089=CARTESIAN_POINT ( 'NONE',  ( 157.9999999999996874, 269.1575001501400379, -45.00000000000000000 ) ) ;
#23091=VECTOR ( 'NONE', #26377, 1000.000000000000000 ) ;
#23098=PLANE ( 'NONE',  #8618 ) ;
#23100=CARTESIAN_POINT ( 'NONE',  ( 158.0000000000016200, 52.97237449702815582, 45.00000000000000000 ) ) ;
#23103=LINE ( 'NONE', #16365, #867 ) ;
#23104=DIRECTION ( 'NONE',  ( 0.8916010070295616874, 0.4528218681378710087, 0.000000000000000000 ) ) ;
#23106=LINE ( 'NONE', #7314, #1195 ) ;
#23112=ORIENTED_EDGE ( 'NONE', *, *, #8775, .F. ) ;
#23113=EDGE_CURVE ( 'NONE', #12854, #61, #20086, .T. ) ;
#23117=VERTEX_POINT ( 'NONE', #13790 ) ;
#23119=CARTESIAN_POINT ( 'NONE',  ( 157.4999999999998579, 176.1121873686267350, 45.00000000000000000 ) ) ;
#23120=VERTEX_POINT ( 'NONE', #20376 ) ;
#23121=ORIENTED_EDGE ( 'NONE', *, *, #22345, .T. ) ;
#23122=VECTOR ( 'NONE', #9400, 1000.000000000000000 ) ;
#23125=VECTOR ( 'NONE', #26026, 999.9999999999998863 ) ;
#23127=DIRECTION ( 'NONE',  ( 0.4528218681380102306, -0.8916010070294909662, 0.000000000000000000 ) ) ;
#23138=EDGE_CURVE ( 'NONE', #9116, #12431, #9179, .T. ) ;
#23143=CARTESIAN_POINT ( 'NONE',  ( 157.9999999999999147, 215.9842499849850697, 45.00000000000000000 ) ) ;
#23149=VERTEX_POINT ( 'NONE', #14209 ) ;
#23151=ORIENTED_EDGE ( 'NONE', *, *, #17927, .F. ) ;
#23154=ORIENTED_EDGE ( 'NONE', *, *, #18917, .T. ) ;
#23155=VECTOR ( 'NONE', #27562, 1000.000000000000000 ) ;
#23156=ORIENTED_EDGE ( 'NONE', *, *, #4998, .F. ) ;
#23160=EDGE_LOOP ( 'NONE', ( #5674, #4071, #23289, #20402 ) ) ;
#23163=VECTOR ( 'NONE', #13402, 1000.000000000000000 ) ;
#23165=ADVANCED_FACE ( 'NONE', ( #11636 ), #9751, .F. ) ;
#23170=DIRECTION ( 'NONE',  ( 0.4528218681382713551, 0.8916010070293584056, -0.000000000000000000 ) ) ;
#23173=ORIENTED_EDGE ( 'NONE', *, *, #14243, .T. ) ;
#23183=ORIENTED_EDGE ( 'NONE', *, *, #664, .F. ) ;
#23184=CARTESIAN_POINT ( 'NONE',  ( 157.9999999999996589, 281.1890001801680796, -45.00000000000000000 ) ) ;
#23187=ORIENTED_EDGE ( 'NONE', *, *, #17778, .F. ) ;
#23188=DIRECTION ( 'NONE',  ( -0.000000000000000000, -0.000000000000000000, -1.000000000000000000 ) ) ;
#23189=CARTESIAN_POINT ( 'NONE',  ( 158.0000000000008242, 128.2086247222394206, 45.00000000000000000 ) ) ;
#23191=ORIENTED_EDGE ( 'NONE', *, *, #23297, .T. ) ;
#23192=DIRECTION ( 'NONE',  ( -0.8916010070293483025, -0.4528218681382912281, 0.000000000000000000 ) ) ;
#23193=DIRECTION ( 'NONE',  ( -0.000000000000000000, -0.000000000000000000, -1.000000000000000000 ) ) ;
#23194=VERTEX_POINT ( 'NONE', #12585 ) ;
#23198=EDGE_LOOP ( 'NONE', ( #26797, #7997, #12767, #22348 ) ) ;
#23199=ORIENTED_EDGE ( 'NONE', *, *, #13382, .F. ) ;
#23201=AXIS2_PLACEMENT_3D ( 'NONE', #10724, #8986, #19899 ) ;
#23203=VECTOR ( 'NONE', #27881, 1000.000000000000000 ) ;
#23204=EDGE_CURVE ( 'NONE', #16446, #11698, #21323, .T. ) ;
#23205=CARTESIAN_POINT ( 'NONE',  ( 158.0000000000015632, 55.98812451204224061, 45.00000000000000000 ) ) ;
#23208=LINE ( 'NONE', #25632, #9658 ) ;
#23210=LINE ( 'NONE', #12166, #7471 ) ;
#23211=DIRECTION ( 'NONE',  ( -0.8916010070293409751, -0.4528218681383056610, 0.000000000000000000 ) ) ;
#23212=CARTESIAN_POINT ( 'NONE',  ( 157.4999999999998579, 143.5098122710352015, 45.00000000000000000 ) ) ;
#23216=LINE ( 'NONE', #25369, #27448 ) ;
#23221=AXIS2_PLACEMENT_3D ( 'NONE', #18233, #14347, #23104 ) ;
#23223=DIRECTION ( 'NONE',  ( 0.000000000000000000, -1.000000000000000000, 0.000000000000000000 ) ) ;
#23226=DIRECTION ( 'NONE',  ( -0.000000000000000000, -0.000000000000000000, -1.000000000000000000 ) ) ;
#23229=ORIENTED_EDGE ( 'NONE', *, *, #9909, .F. ) ;
#23231=EDGE_CURVE ( 'NONE', #19001, #16156, #27912, .T. ) ;
#23234=ADVANCED_FACE ( 'NONE', ( #8258, #9887 ), #8401, .F. ) ;
#23236=VERTEX_POINT ( 'NONE', #21461 ) ;
#23241=FACE_OUTER_BOUND ( 'NONE', #20985, .T. ) ;
#23248=CARTESIAN_POINT ( 'NONE',  ( 158.0000000000008527, 125.7007497147323818, 45.00000000000000000 ) ) ;
#23250=CARTESIAN_POINT ( 'NONE',  ( 157.9999999999997158, 263.6338751276190351, -45.00000000000000000 ) ) ;
#23255=CARTESIAN_POINT ( 'NONE',  ( 157.9999999999996305, 288.7126252026890256, 45.00000000000000000 ) ) ;
#23259=ORIENTED_EDGE ( 'NONE', *, *, #10977, .T. ) ;
#23262=ADVANCED_FACE ( 'NONE', ( #28055 ), #17013, .F. ) ;
#23266=EDGE_LOOP ( 'NONE', ( #25523, #16103, #9984, #3599 ) ) ;
#23267=ORIENTED_EDGE ( 'NONE', *, *, #10517, .F. ) ;
#23270=EDGE_CURVE ( 'NONE', #83, #23194, #1917, .T. ) ;
#23272=EDGE_CURVE ( 'NONE', #24388, #24788, #28196, .T. ) ;
#23274=LINE ( 'NONE', #1573, #25238 ) ;
#23276=PLANE ( 'NONE',  #21055 ) ;
#23282=LINE ( 'NONE', #14386, #23040 ) ;
#23286=ORIENTED_EDGE ( 'NONE', *, *, #983, .T. ) ;
#23289=ORIENTED_EDGE ( 'NONE', *, *, #16972, .F. ) ;
#23290=AXIS2_PLACEMENT_3D ( 'NONE', #4181, #10806, #19563 ) ;
#23295=ORIENTED_EDGE ( 'NONE', *, *, #17888, .T. ) ;
#23297=EDGE_CURVE ( 'NONE', #883, #11955, #11117, .T. ) ;
#23299=EDGE_CURVE ( 'NONE', #729, #26043, #2479, .T. ) ;
#23300=DIRECTION ( 'NONE',  ( 1.000000000000000000, 0.000000000000000000, -0.000000000000000000 ) ) ;
#23303=ORIENTED_EDGE ( 'NONE', *, *, #15869, .F. ) ;
#23305=CARTESIAN_POINT ( 'NONE',  ( 158.0000000000002558, 183.3818748873943889, 45.00000000000000000 ) ) ;
#23306=CARTESIAN_POINT ( 'NONE',  ( 157.4999999999998579, 70.78143705333094715, 45.00000000000000000 ) ) ;
#23312=ORIENTED_EDGE ( 'NONE', *, *, #12866, .T. ) ;
#23314=VECTOR ( 'NONE', #20875, 1000.000000000000114 ) ;
#23316=DIRECTION ( 'NONE',  ( -0.000000000000000000, 0.000000000000000000, -1.000000000000000000 ) ) ;
#23319=DIRECTION ( 'NONE',  ( -0.8916010070293485246, -0.4528218681382906730, 0.000000000000000000 ) ) ;
#23320=ORIENTED_EDGE ( 'NONE', *, *, #15762, .F. ) ;
#23323=DIRECTION ( 'NONE',  ( -0.8916010070296834789, -0.4528218681376312005, 0.000000000000000000 ) ) ;
#23325=CARTESIAN_POINT ( 'NONE',  ( 157.4999999999996589, 276.4271876689075498, 45.00000000000000000 ) ) ;
#23326=ORIENTED_EDGE ( 'NONE', *, *, #27306, .F. ) ;
#23328=CARTESIAN_POINT ( 'NONE',  ( 157.4999999999998579, 103.3838121509225090, 45.00000000000000000 ) ) ;
#23332=EDGE_LOOP ( 'NONE', ( #1660, #24776, #11433, #11304 ) ) ;
#23333=EDGE_CURVE ( 'NONE', #1220, #24140, #18011, .T. ) ;
#23336=VECTOR ( 'NONE', #10144, 999.9999999999998863 ) ;
#23339=VERTEX_POINT ( 'NONE', #56 ) ;
#23341=ORIENTED_EDGE ( 'NONE', *, *, #9977, .T. ) ;
#23343=LINE ( 'NONE', #1503, #3435 ) ;
#23346=DIRECTION ( 'NONE',  ( 0.8916010070295820045, -0.4528218681378310406, 0.000000000000000000 ) ) ;
#23350=LINE ( 'NONE', #10421, #17048 ) ;
#23351=LINE ( 'NONE', #25638, #27882 ) ;
#23353=ORIENTED_EDGE ( 'NONE', *, *, #20447, .T. ) ;
#23355=DIRECTION ( 'NONE',  ( -0.000000000000000000, -0.000000000000000000, -1.000000000000000000 ) ) ;
#23356=CARTESIAN_POINT ( 'NONE',  ( 158.0000000000015064, 63.00387452705633251, -45.00000000000000000 ) ) ;
#23359=ADVANCED_FACE ( 'NONE', ( #20013 ), #8814, .F. ) ;
#23363=ORIENTED_EDGE ( 'NONE', *, *, #16523, .T. ) ;
#23364=ORIENTED_EDGE ( 'NONE', *, *, #7692, .F. ) ;
#23368=VECTOR ( 'NONE', #11976, 1000.000000000000000 ) ;
#23370=ORIENTED_EDGE ( 'NONE', *, *, #14741, .F. ) ;
#23373=LINE ( 'NONE', #19629, #13422 ) ;
#23377=VECTOR ( 'NONE', #18400, 1000.000000000000000 ) ;
#23386=VERTEX_POINT ( 'NONE', #24474 ) ;
#23391=VERTEX_POINT ( 'NONE', #24323 ) ;
#23392=ORIENTED_EDGE ( 'NONE', *, *, #14074, .F. ) ;
#23393=AXIS2_PLACEMENT_3D ( 'NONE', #5269, #958, #2531 ) ;
#23394=EDGE_CURVE ( 'NONE', #5337, #23117, #9104, .T. ) ;
#23396=AXIS2_PLACEMENT_3D ( 'NONE', #7482, #23127, #27415 ) ;
#23397=ORIENTED_EDGE ( 'NONE', *, *, #18662, .F. ) ;
#23399=ORIENTED_EDGE ( 'NONE', *, *, #16229, .T. ) ;
#23401=ORIENTED_EDGE ( 'NONE', *, *, #16085, .F. ) ;
#23405=EDGE_CURVE ( 'NONE', #4212, #13878, #11563, .T. ) ;
#23406=VECTOR ( 'NONE', #2955, 1000.000000000000227 ) ;
#23407=LINE ( 'NONE', #12788, #26121 ) ;
#23408=LINE ( 'NONE', #10339, #15777 ) ;
#23412=FACE_OUTER_BOUND ( 'NONE', #6089, .T. ) ;
#23414=ADVANCED_FACE ( 'NONE', ( #17862 ), #13148, .F. ) ;
#23416=CARTESIAN_POINT ( 'NONE',  ( 158.0000000000014495, 68.01962454207041731, 45.00000000000000000 ) ) ;
#23418=LINE ( 'NONE', #21403, #22594 ) ;
#23419=ORIENTED_EDGE ( 'NONE', *, *, #22946, .F. ) ;
#23421=EDGE_CURVE ( 'NONE', #13130, #9383, #2337, .T. ) ;
#23422=VECTOR ( 'NONE', #22651, 1000.000000000000000 ) ;
#23424=EDGE_LOOP ( 'NONE', ( #4157, #20735, #3749, #20933 ) ) ;
#23427=ORIENTED_EDGE ( 'NONE', *, *, #21569, .F. ) ;
#23430=CARTESIAN_POINT ( 'NONE',  ( 158.0000000000015916, 53.48024950453520177, 45.00000000000000000 ) ) ;
#23431=CARTESIAN_POINT ( 'NONE',  ( 158.0000000000002274, 183.8897498949014278, -45.00000000000000000 ) ) ;
#23433=VERTEX_POINT ( 'NONE', #199 ) ;
#23436=AXIS2_PLACEMENT_3D ( 'NONE', #13965, #3013, #16389 ) ;
#23440=ORIENTED_EDGE ( 'NONE', *, *, #22025, .F. ) ;
#23442=AXIS2_PLACEMENT_3D ( 'NONE', #712, #23877, #20237 ) ;
#23446=DIRECTION ( 'NONE',  ( 0.4528218681377111920, -0.8916010070296429557, 0.000000000000000000 ) ) ;
#23447=CARTESIAN_POINT ( 'NONE',  ( 157.4999999999998579, 73.28931206083800021, -45.00000000000000000 ) ) ;
#23448=AXIS2_PLACEMENT_3D ( 'NONE', #19960, #17513, #24705 ) ;
#23450=VERTEX_POINT ( 'NONE', #26772 ) ;
#23451=LINE ( 'NONE', #12132, #23314 ) ;
#23452=CARTESIAN_POINT ( 'NONE',  ( 158.0000000000011084, 98.62199963966197913, -45.00000000000000000 ) ) ;
#23453=DIRECTION ( 'NONE',  ( 1.000000000000000000, 0.000000000000000000, -0.000000000000000000 ) ) ;
#23454=EDGE_CURVE ( 'NONE', #13425, #2326, #8960, .T. ) ;
#23458=EDGE_CURVE ( 'NONE', #11964, #24937, #6797, .T. ) ;
#23460=DIRECTION ( 'NONE',  ( -0.8916010070298665546, -0.4528218681372709331, 0.000000000000000000 ) ) ;
#23464=DIRECTION ( 'NONE',  ( 0.8916010070293584056, -0.4528218681382712996, 0.000000000000000000 ) ) ;
#23465=DIRECTION ( 'NONE',  ( 0.8916010070294301260, 0.4528218681381301347, 0.000000000000000000 ) ) ;
#23474=ORIENTED_EDGE ( 'NONE', *, *, #495, .T. ) ;
#23476=EDGE_CURVE ( 'NONE', #17780, #8629, #27457, .T. ) ;
#23477=ORIENTED_EDGE ( 'NONE', *, *, #13454, .T. ) ;
#23480=EDGE_CURVE ( 'NONE', #12943, #1444, #16011, .T. ) ;
#23484=CARTESIAN_POINT ( 'NONE',  ( 157.9999999999998295, 226.5236250225210313, 45.00000000000000000 ) ) ;
#23485=CARTESIAN_POINT ( 'NONE',  ( 158.0000000000009663, 111.1613746771971876, 45.00000000000000000 ) ) ;
#23489=CARTESIAN_POINT ( 'NONE',  ( 157.9999999999996305, 288.7126252026890256, 45.00000000000000000 ) ) ;
#23491=DIRECTION ( 'NONE',  ( 0.8916010070297745171, -0.4528218681374519550, 0.000000000000000000 ) ) ;
#23492=VECTOR ( 'NONE', #6647, 1000.000000000000000 ) ;
#23495=ORIENTED_EDGE ( 'NONE', *, *, #11568, .F. ) ;
#23496=EDGE_CURVE ( 'NONE', #15403, #1139, #11981, .T. ) ;
#23497=DIRECTION ( 'NONE',  ( 0.000000000000000000, -1.000000000000000000, 0.000000000000000000 ) ) ;
#23499=PLANE ( 'NONE',  #14225 ) ;
#23503=VERTEX_POINT ( 'NONE', #27598 ) ;
#23508=EDGE_LOOP ( 'NONE', ( #3962, #21912, #4192 ) ) ;
#23509=LINE ( 'NONE', #3824, #8563 ) ;
#23510=EDGE_LOOP ( 'NONE', ( #17032, #21981, #10161, #14444 ) ) ;
#23511=ORIENTED_EDGE ( 'NONE', *, *, #1428, .T. ) ;
#23512=VECTOR ( 'NONE', #10140, 1000.000000000000114 ) ;
#23513=CARTESIAN_POINT ( 'NONE',  ( 157.4999999999997726, 243.8248125713165280, 45.00000000000000000 ) ) ;
#23514=DIRECTION ( 'NONE',  ( -0.8916010070295719014, -0.4528218681378510246, 0.000000000000000000 ) ) ;
#23515=CARTESIAN_POINT ( 'NONE',  ( 157.4999999999998579, 148.5255622860493077, 45.00000000000000000 ) ) ;
#23520=PLANE ( 'NONE',  #14628 ) ;
#23524=DIRECTION ( 'NONE',  ( 0.000000000000000000, 0.000000000000000000, -1.000000000000000000 ) ) ;
#23527=CARTESIAN_POINT ( 'NONE',  ( 157.4999999999994600, 213.7303124812313513, 45.00000000000000000 ) ) ;
#23530=VERTEX_POINT ( 'NONE', #18299 ) ;
#23533=EDGE_CURVE ( 'NONE', #27901, #19692, #3194, .T. ) ;
#23535=DIRECTION ( 'NONE',  ( 0.8916010070293409751, 0.4528218681383056610, 0.000000000000000000 ) ) ;
#23541=EDGE_CURVE ( 'NONE', #21119, #15548, #27049, .T. ) ;
#23543=ORIENTED_EDGE ( 'NONE', *, *, #9598, .F. ) ;
#23544=VERTEX_POINT ( 'NONE', #16427 ) ;
#23546=ORIENTED_EDGE ( 'NONE', *, *, #8113, .T. ) ;
#23552=CARTESIAN_POINT ( 'NONE',  ( 158.0000000000014495, 66.01962454207041731, -45.00000000000000000 ) ) ;
#23557=EDGE_CURVE ( 'NONE', #14195, #9494, #3332, .T. ) ;
#23558=LINE ( 'NONE', #25557, #14451 ) ;
#23559=LINE ( 'NONE', #20972, #13673 ) ;
#23560=DIRECTION ( 'NONE',  ( 0.8916010070298860946, -0.4528218681372321863, 0.000000000000000000 ) ) ;
#23562=CARTESIAN_POINT ( 'NONE',  ( 158.0000000000014211, 73.03537455708450921, 45.00000000000000000 ) ) ;
#23563=CARTESIAN_POINT ( 'NONE',  ( 157.4999999999997726, 248.8405625863305204, -45.00000000000000000 ) ) ;
#23569=VECTOR ( 'NONE', #26761, 1000.000000000000000 ) ;
#23571=DIRECTION ( 'NONE',  ( 0.4528218681382319422, 0.8916010070293783896, -0.000000000000000000 ) ) ;
#23572=VERTEX_POINT ( 'NONE', #21000 ) ;
#23576=DIRECTION ( 'NONE',  ( 0.8916010070293384215, 0.4528218681383106015, 0.000000000000000000 ) ) ;
#23579=ORIENTED_EDGE ( 'NONE', *, *, #17650, .T. ) ;
#23580=ADVANCED_FACE ( 'NONE', ( #1327 ), #10096, .F. ) ;
#23581=LINE ( 'NONE', #11971, #8125 ) ;
#23585=ORIENTED_EDGE ( 'NONE', *, *, #19310, .T. ) ;
#23593=FACE_OUTER_BOUND ( 'NONE', #12855, .T. ) ;
#23595=ORIENTED_EDGE ( 'NONE', *, *, #22761, .T. ) ;
#23597=CARTESIAN_POINT ( 'NONE',  ( 158.0000000000010516, 105.6377496546760568, 45.00000000000000000 ) ) ;
#23599=DIRECTION ( 'NONE',  ( 0.000000000000000000, -1.000000000000000000, 0.000000000000000000 ) ) ;
#23601=DIRECTION ( 'NONE',  ( 0.4528218681370910770, -0.8916010070299578150, 0.000000000000000000 ) ) ;
#23602=EDGE_CURVE ( 'NONE', #8797, #3340, #21286, .T. ) ;
#23605=DIRECTION ( 'NONE',  ( 0.8916010070295106171, -0.4528218681379715393, 0.000000000000000000 ) ) ;
#23615=DIRECTION ( 'NONE',  ( 0.8916010070296940260, 0.4528218681376106058, 0.000000000000000000 ) ) ;
#23616=VERTEX_POINT ( 'NONE', #8364 ) ;
#23619=ADVANCED_FACE ( 'NONE', ( #5778 ), #19132, .F. ) ;
#23620=FACE_OUTER_BOUND ( 'NONE', #18006, .T. ) ;
#23622=CARTESIAN_POINT ( 'NONE',  ( 158.0000000000016200, 52.97237449702815582, 45.00000000000000000 ) ) ;
#23627=VECTOR ( 'NONE', #13046, 999.9999999999998863 ) ;
#23635=CARTESIAN_POINT ( 'NONE',  ( 157.4999999999998579, 45.70268697826052318, -45.00000000000000000 ) ) ;
#23636=LINE ( 'NONE', #26202, #21499 ) ;
#23637=LINE ( 'NONE', #4369, #6144 ) ;
#23641=DIRECTION ( 'NONE',  ( 0.4528218681383106015, 0.8916010070293384215, -0.000000000000000000 ) ) ;
#23643=( NAMED_UNIT ( * ) PLANE_ANGLE_UNIT ( ) SI_UNIT ( $, .RADIAN. ) );
#23646=DIRECTION ( 'NONE',  ( 0.000000000000000000, -1.000000000000000000, 0.000000000000000000 ) ) ;
#23659=CARTESIAN_POINT ( 'NONE',  ( 157.4999999999998579, 146.0176872785422404, -45.00000000000000000 ) ) ;
#23661=LINE ( 'NONE', #19490, #6071 ) ;
#23669=PLANE ( 'NONE',  #19554 ) ;
#23670=VECTOR ( 'NONE', #3331, 1000.000000000000000 ) ;
#23673=CARTESIAN_POINT ( 'NONE',  ( 157.9999999999998295, 231.0315000300280417, 45.00000000000000000 ) ) ;
#23674=DIRECTION ( 'NONE',  ( 0.8916010070293383105, -0.4528218681383106015, 0.000000000000000000 ) ) ;
#23675=VECTOR ( 'NONE', #16590, 1000.000000000000000 ) ;
#23677=CARTESIAN_POINT ( 'NONE',  ( 157.9999999999997726, 248.5866250825770294, -45.00000000000000000 ) ) ;
#23678=CARTESIAN_POINT ( 'NONE',  ( 157.9999999999997158, 261.6338751276190351, 45.00000000000000000 ) ) ;
#23687=ADVANCED_FACE ( 'NONE', ( #19562 ), #28020, .F. ) ;
#23688=EDGE_CURVE ( 'NONE', #19409, #18723, #3612, .T. ) ;
#23689=ORIENTED_EDGE ( 'NONE', *, *, #24971, .F. ) ;
#23693=CARTESIAN_POINT ( 'NONE',  ( 158.0000000000000284, 203.9527499549551806, 45.00000000000000000 ) ) ;
#23698=DIRECTION ( 'NONE',  ( -0.8916010070296226386, -0.4528218681377511046, 0.000000000000000000 ) ) ;
#23701=FACE_OUTER_BOUND ( 'NONE', #2754, .T. ) ;
#23706=CARTESIAN_POINT ( 'NONE',  ( 158.0000000000007958, 130.7164997297464595, -45.00000000000000000 ) ) ;
#23711=VERTEX_POINT ( 'NONE', #3900 ) ;
#23725=ORIENTED_EDGE ( 'NONE', *, *, #11868, .F. ) ;
#23726=VECTOR ( 'NONE', #12228, 1000.000000000000000 ) ;
#23733=VERTEX_POINT ( 'NONE', #10945 ) ;
#23734=LINE ( 'NONE', #4187, #6795 ) ;
#23751=DIRECTION ( 'NONE',  ( -0.000000000000000000, -0.000000000000000000, -1.000000000000000000 ) ) ;
#23758=ORIENTED_EDGE ( 'NONE', *, *, #17759, .F. ) ;
#23759=CARTESIAN_POINT ( 'NONE',  ( 158.0000000000009948, 110.6534996696901345, -45.00000000000000000 ) ) ;
#23760=ADVANCED_FACE ( 'NONE', ( #13116 ), #26436, .F. ) ;
#23765=LINE ( 'NONE', #4076, #20906 ) ;
#23772=PLANE ( 'NONE',  #1007 ) ;
#23775=VERTEX_POINT ( 'NONE', #17541 ) ;
#23776=EDGE_CURVE ( 'NONE', #4884, #13140, #21861, .T. ) ;
#23777=DIRECTION ( 'NONE',  ( -0.8916010070297749612, -0.4528218681374510668, 0.000000000000000000 ) ) ;
#23781=DIRECTION ( 'NONE',  ( -0.8916010070293384215, 0.4528218681383106015, 0.000000000000000000 ) ) ;
#23782=DIRECTION ( 'NONE',  ( -0.8916010070294402290, -0.4528218681381102062, 0.000000000000000000 ) ) ;
#23785=EDGE_CURVE ( 'NONE', #7159, #15242, #2167, .T. ) ;
#23786=ADVANCED_FACE ( 'NONE', ( #4460 ), #4891, .F. ) ;
#23789=VERTEX_POINT ( 'NONE', #24161 ) ;
#23790=DIRECTION ( 'NONE',  ( 0.4528218681383106015, -0.8916010070293384215, 0.000000000000000000 ) ) ;
#23791=VECTOR ( 'NONE', #4360, 1000.000000000000000 ) ;
#23794=ORIENTED_EDGE ( 'NONE', *, *, #1428, .F. ) ;
#23796=ORIENTED_EDGE ( 'NONE', *, *, #23944, .F. ) ;
#23805=PLANE ( 'NONE',  #18811 ) ;
#23806=DIRECTION ( 'NONE',  ( 0.000000000000000000, -1.000000000000000000, 0.000000000000000000 ) ) ;
#23812=VECTOR ( 'NONE', #7058, 1000.000000000000000 ) ;
#23813=LINE ( 'NONE', #6843, #4837 ) ;
#23816=CARTESIAN_POINT ( 'NONE',  ( 157.4999999999998579, 85.82868709837320864, 45.00000000000000000 ) ) ;
#23817=VERTEX_POINT ( 'NONE', #17828 ) ;
#23819=CARTESIAN_POINT ( 'NONE',  ( 158.0000000000012221, 90.59049960963380954, 45.00000000000000000 ) ) ;
#23820=DIRECTION ( 'NONE',  ( -0.8916010070296023216, -0.4528218681377911281, 0.000000000000000000 ) ) ;
#23821=EDGE_LOOP ( 'NONE', ( #28222, #6546, #14217, #10153 ) ) ;
#23826=VERTEX_POINT ( 'NONE', #11232 ) ;
#23828=ORIENTED_EDGE ( 'NONE', *, *, #14170, .T. ) ;
#23830=VERTEX_POINT ( 'NONE', #19983 ) ;
#23831=VECTOR ( 'NONE', #19220, 1000.000000000000000 ) ;
#23832=VERTEX_POINT ( 'NONE', #9216 ) ;
#23834=ORIENTED_EDGE ( 'NONE', *, *, #7062, .F. ) ;
#23835=LINE ( 'NONE', #10764, #6761 ) ;
#23837=EDGE_CURVE ( 'NONE', #1313, #16168, #6910, .T. ) ;
#23840=DIRECTION ( 'NONE',  ( 0.8916010070299774659, -0.4528218681370523302, 0.000000000000000000 ) ) ;
#23841=DIRECTION ( 'NONE',  ( -0.8916010070294903000, 0.4528218681380115629, 0.000000000000000000 ) ) ;
#23842=VECTOR ( 'NONE', #5334, 999.9999999999998863 ) ;
#23845=CARTESIAN_POINT ( 'NONE',  ( 158.0000000000009379, 118.1771246922112653, 45.00000000000000000 ) ) ;
#23848=DIRECTION ( 'NONE',  ( -0.8916010070295208312, 0.4528218681379515553, 0.000000000000000000 ) ) ;
#23850=LINE ( 'NONE', #12517, #2335 ) ;
#23855=EDGE_CURVE ( 'NONE', #17304, #25380, #18123, .T. ) ;
#23856=EDGE_CURVE ( 'NONE', #27854, #11176, #15979, .T. ) ;
#23858=EDGE_LOOP ( 'NONE', ( #15907, #16455, #6327, #16356 ) ) ;
#23860=ORIENTED_EDGE ( 'NONE', *, *, #20073, .F. ) ;
#23862=CARTESIAN_POINT ( 'NONE',  ( 157.4999999999996589, 281.4429376839215138, 45.00000000000000000 ) ) ;
#23863=VECTOR ( 'NONE', #18611, 1000.000000000000000 ) ;
#23864=DIRECTION ( 'NONE',  ( 0.8916010070296838119, 0.4528218681376304788, 0.000000000000000000 ) ) ;
#23865=ORIENTED_EDGE ( 'NONE', *, *, #18979, .F. ) ;
#23870=CARTESIAN_POINT ( 'NONE',  ( 158.0000000000009663, 113.6692496847042264, 45.00000000000000000 ) ) ;
#23871=ORIENTED_EDGE ( 'NONE', *, *, #7857, .T. ) ;
#23873=ORIENTED_EDGE ( 'NONE', *, *, #25693, .T. ) ;
#23877=DIRECTION ( 'NONE',  ( 0.4528218681380314914, 0.8916010070294801970, -0.000000000000000000 ) ) ;
#23879=ORIENTED_EDGE ( 'NONE', *, *, #19086, .F. ) ;
#23880=VECTOR ( 'NONE', #13012, 1000.000000000000000 ) ;
#23888=EDGE_CURVE ( 'NONE', #15403, #13270, #5184, .T. ) ;
#23892=ORIENTED_EDGE ( 'NONE', *, *, #23888, .F. ) ;
#23893=LINE ( 'NONE', #26999, #9770 ) ;
#23898=ORIENTED_EDGE ( 'NONE', *, *, #7344, .T. ) ;
#23902=VECTOR ( 'NONE', #7386, 1000.000000000000000 ) ;
#23903=DIRECTION ( 'NONE',  ( 0.4528218681377710886, -0.8916010070296124246, 0.000000000000000000 ) ) ;
#23905=VERTEX_POINT ( 'NONE', #3441 ) ;
#23906=DIRECTION ( 'NONE',  ( 0.000000000000000000, -1.000000000000000000, 0.000000000000000000 ) ) ;
#23907=VECTOR ( 'NONE', #18269, 1000.000000000000114 ) ;
#23911=LINE ( 'NONE', #10983, #23880 ) ;
#23912=DIRECTION ( 'NONE',  ( 0.000000000000000000, -1.000000000000000000, 0.000000000000000000 ) ) ;
#23913=ADVANCED_FACE ( 'NONE', ( #13826 ), #3158, .F. ) ;
#23915=ORIENTED_EDGE ( 'NONE', *, *, #26187, .T. ) ;
#23916=DIRECTION ( 'NONE',  ( 0.4528218681377511601, -0.8916010070296226386, 0.000000000000000000 ) ) ;
#23920=LINE ( 'NONE', #10710, #26774 ) ;
#23922=PLANE ( 'NONE',  #22447 ) ;
#23923=AXIS2_PLACEMENT_3D ( 'NONE', #9759, #27264, #8588 ) ;
#23925=DIRECTION ( 'NONE',  ( -0.8916010070294700940, 0.4528218681380514754, 0.000000000000000000 ) ) ;
#23926=CARTESIAN_POINT ( 'NONE',  ( 157.4999999999997158, 263.8878126313725829, 45.00000000000000000 ) ) ;
#23927=CARTESIAN_POINT ( 'NONE',  ( 187.4999999999996305, 288.9665627064425166, -45.00000000000000000 ) ) ;
#23937=ORIENTED_EDGE ( 'NONE', *, *, #14019, .T. ) ;
#23938=CARTESIAN_POINT ( 'NONE',  ( 157.4999999999998579, 130.9704372334999789, -45.00000000000000000 ) ) ;
#23939=ORIENTED_EDGE ( 'NONE', *, *, #2482, .F. ) ;
#23941=EDGE_CURVE ( 'NONE', #18196, #17639, #20687, .T. ) ;
#23944=EDGE_CURVE ( 'NONE', #16156, #13878, #16119, .T. ) ;
#23945=AXIS2_PLACEMENT_3D ( 'NONE', #16988, #3908, #21297 ) ;
#23946=CARTESIAN_POINT ( 'NONE',  ( 158.0000000000002558, 181.3818748873943889, -45.00000000000000000 ) ) ;
#23949=VECTOR ( 'NONE', #8947, 1000.000000000000227 ) ;
#23951=LINE ( 'NONE', #13462, #27983 ) ;
#23953=LINE ( 'NONE', #57, #19533 ) ;
#23954=DIRECTION ( 'NONE',  ( -0.000000000000000000, -0.000000000000000000, -1.000000000000000000 ) ) ;
#23958=CARTESIAN_POINT ( 'NONE',  ( 158.0000000000004832, 161.3188748273380213, 45.00000000000000000 ) ) ;
#23963=LINE ( 'NONE', #23678, #2500 ) ;
#23966=VECTOR ( 'NONE', #12518, 1000.000000000000114 ) ;
#23968=ORIENTED_EDGE ( 'NONE', *, *, #7094, .T. ) ;
#23971=VECTOR ( 'NONE', #26293, 1000.000000000000000 ) ;
#23973=VECTOR ( 'NONE', #4553, 1000.000000000000114 ) ;
#23978=CARTESIAN_POINT ( 'NONE',  ( 157.9999999999996305, 283.6968751876750616, 45.00000000000000000 ) ) ;
#23979=VECTOR ( 'NONE', #4569, 1000.000000000000000 ) ;
#23980=CARTESIAN_POINT ( 'NONE',  ( 158.0000000000000853, 200.9369999399436892, 45.00000000000000000 ) ) ;
#23983=CARTESIAN_POINT ( 'NONE',  ( 158.0000000000010232, 108.1456246621830957, 45.00000000000000000 ) ) ;
#23985=VECTOR ( 'NONE', #10713, 1000.000000000000000 ) ;
#23988=ADVANCED_FACE ( 'NONE', ( #7493 ), #16258, .F. ) ;
#23990=DIRECTION ( 'NONE',  ( -0.000000000000000000, -0.000000000000000000, -1.000000000000000000 ) ) ;
#23994=DIRECTION ( 'NONE',  ( -0.000000000000000000, -0.000000000000000000, -1.000000000000000000 ) ) ;
#23995=CARTESIAN_POINT ( 'NONE',  ( 157.4999999999998295, 218.7460624962465090, 45.00000000000000000 ) ) ;
#23996=ORIENTED_EDGE ( 'NONE', *, *, #21129, .T. ) ;
#24002=EDGE_LOOP ( 'NONE', ( #25418, #4013, #7823, #7001 ) ) ;
#24008=CARTESIAN_POINT ( 'NONE',  ( 158.0000000000008527, 123.7007497147323960, 45.00000000000000000 ) ) ;
#24010=VECTOR ( 'NONE', #7285, 1000.000000000000000 ) ;
#24012=LINE ( 'NONE', #16834, #22888 ) ;
#24019=EDGE_CURVE ( 'NONE', #14062, #15041, #25703, .T. ) ;
#24020=EDGE_CURVE ( 'NONE', #21204, #11039, #17086, .T. ) ;
#24021=DIRECTION ( 'NONE',  ( 1.000000000000000000, 0.000000000000000000, -0.000000000000000000 ) ) ;
#24025=ORIENTED_EDGE ( 'NONE', *, *, #6020, .T. ) ;
#24027=CARTESIAN_POINT ( 'NONE',  ( 157.4999999999998579, 95.86018712840139244, 45.00000000000000000 ) ) ;
#24028=CARTESIAN_POINT ( 'NONE',  ( 157.4999999999998579, 93.35231212089433939, -45.00000000000000000 ) ) ;
#24029=CARTESIAN_POINT ( 'NONE',  ( 158.0000000000016485, 48.46449948952110987, -45.00000000000000000 ) ) ;
#24031=LINE ( 'NONE', #19992, #25417 ) ;
#24035=FACE_OUTER_BOUND ( 'NONE', #11237, .T. ) ;
#24036=VERTEX_POINT ( 'NONE', #5741 ) ;
#24039=ORIENTED_EDGE ( 'NONE', *, *, #26622, .F. ) ;
#24040=FACE_OUTER_BOUND ( 'NONE', #21481, .T. ) ;
#24044=ORIENTED_EDGE ( 'NONE', *, *, #11513, .F. ) ;
#24047=EDGE_CURVE ( 'NONE', #14163, #8537, #23558, .T. ) ;
#24050=VERTEX_POINT ( 'NONE', #14946 ) ;
#24051=VECTOR ( 'NONE', #20696, 1000.000000000000000 ) ;
#24056=DIRECTION ( 'NONE',  ( -0.000000000000000000, -0.000000000000000000, -1.000000000000000000 ) ) ;
#24057=LINE ( 'NONE', #13421, #23791 ) ;
#24059=CARTESIAN_POINT ( 'NONE',  ( 158.0000000000000284, 205.9527499549551806, 45.00000000000000000 ) ) ;
#24061=ORIENTED_EDGE ( 'NONE', *, *, #17505, .T. ) ;
#24063=CARTESIAN_POINT ( 'NONE',  ( 157.4999999999994600, 216.2381874887387880, 45.00000000000000000 ) ) ;
#24064=DIRECTION ( 'NONE',  ( -0.000000000000000000, -0.000000000000000000, -1.000000000000000000 ) ) ;
#24065=CARTESIAN_POINT ( 'NONE',  ( 158.0000000000009379, 116.1771246922112653, -45.00000000000000000 ) ) ;
#24066=ORIENTED_EDGE ( 'NONE', *, *, #6909, .T. ) ;
#24068=DIRECTION ( 'NONE',  ( 0.000000000000000000, -1.000000000000000000, 0.000000000000000000 ) ) ;
#24069=DIRECTION ( 'NONE',  ( -1.000000000000000000, 1.850371707708594366E-15, 0.000000000000000000 ) ) ;
#24075=ORIENTED_EDGE ( 'NONE', *, *, #21790, .T. ) ;
#24080=ORIENTED_EDGE ( 'NONE', *, *, #13485, .F. ) ;
#24081=DIRECTION ( 'NONE',  ( 0.8916010070294395629, -0.4528218681381114274, 0.000000000000000000 ) ) ;
#24083=VECTOR ( 'NONE', #6975, 1000.000000000000000 ) ;
#24084=VERTEX_POINT ( 'NONE', #8472 ) ;
#24085=ORIENTED_EDGE ( 'NONE', *, *, #14232, .F. ) ;
#24086=DIRECTION ( 'NONE',  ( 0.000000000000000000, -1.000000000000000000, 0.000000000000000000 ) ) ;
#24099=PLANE ( 'NONE',  #15856 ) ;
#24104=ORIENTED_EDGE ( 'NONE', *, *, #21709, .T. ) ;
#24108=VECTOR ( 'NONE', #9248, 1000.000000000000000 ) ;
#24115=EDGE_LOOP ( 'NONE', ( #8338, #25549, #8710, #6355 ) ) ;
#24116=VERTEX_POINT ( 'NONE', #3867 ) ;
#24119=ORIENTED_EDGE ( 'NONE', *, *, #27346, .F. ) ;
#24122=CARTESIAN_POINT ( 'NONE',  ( 157.4999999999998579, 178.6200623761337738, 45.00000000000000000 ) ) ;
#24126=DIRECTION ( 'NONE',  ( 1.000000000000000000, 0.000000000000000000, -0.000000000000000000 ) ) ;
#24133=VECTOR ( 'NONE', #23954, 1000.000000000000000 ) ;
#24136=LINE ( 'NONE', #26413, #4507 ) ;
#24139=CARTESIAN_POINT ( 'NONE',  ( 187.4999999999996305, 40.68693696324645970, 45.00000000000000000 ) ) ;
#24140=VERTEX_POINT ( 'NONE', #8329 ) ;
#24146=ORIENTED_EDGE ( 'NONE', *, *, #7995, .F. ) ;
#24147=VECTOR ( 'NONE', #2583, 999.9999999999998863 ) ;
#24148=EDGE_CURVE ( 'NONE', #19656, #24242, #10913, .T. ) ;
#24149=ORIENTED_EDGE ( 'NONE', *, *, #5389, .F. ) ;
#24150=EDGE_CURVE ( 'NONE', #12678, #23433, #7025, .T. ) ;
#24151=FACE_OUTER_BOUND ( 'NONE', #18333, .T. ) ;
#24152=LINE ( 'NONE', #10505, #12691 ) ;
#24153=ORIENTED_EDGE ( 'NONE', *, *, #16500, .F. ) ;
#24154=EDGE_CURVE ( 'NONE', #26356, #15878, #6454, .T. ) ;
#24161=CARTESIAN_POINT ( 'NONE',  ( 157.9999999999996589, 276.6811251726610976, 45.00000000000000000 ) ) ;
#24164=VECTOR ( 'NONE', #11108, 1000.000000000000227 ) ;
#24165=ORIENTED_EDGE ( 'NONE', *, *, #11211, .T. ) ;
#24171=ORIENTED_EDGE ( 'NONE', *, *, #7742, .T. ) ;
#24173=CARTESIAN_POINT ( 'NONE',  ( 158.0000000000003979, 168.8424998498591663, -45.00000000000000000 ) ) ;
#24175=VERTEX_POINT ( 'NONE', #284 ) ;
#24176=ORIENTED_EDGE ( 'NONE', *, *, #10618, .F. ) ;
#24179=EDGE_CURVE ( 'NONE', #4619, #1981, #15517, .T. ) ;
#24185=LINE ( 'NONE', #13275, #8889 ) ;
#24186=VERTEX_POINT ( 'NONE', #15230 ) ;
#24189=DIRECTION ( 'NONE',  ( 0.000000000000000000, -1.000000000000000000, 0.000000000000000000 ) ) ;
#24192=CARTESIAN_POINT ( 'NONE',  ( 158.0000000000014211, 71.03537455708449500, 45.00000000000000000 ) ) ;
#24195=EDGE_LOOP ( 'NONE', ( #4382, #4605, #25299, #17713 ) ) ;
#24196=CARTESIAN_POINT ( 'NONE',  ( 157.4999999999998579, 171.0964373536126573, 45.00000000000000000 ) ) ;
#24197=FACE_OUTER_BOUND ( 'NONE', #15694, .T. ) ;
#24202=DIRECTION ( 'NONE',  ( 0.8916010070298563406, 0.4528218681372909171, 0.000000000000000000 ) ) ;
#24205=CARTESIAN_POINT ( 'NONE',  ( 157.4999999999998579, 191.1594374136689964, 45.00000000000000000 ) ) ;
#24208=LINE ( 'NONE', #24638, #21171 ) ;
#24210=ORIENTED_EDGE ( 'NONE', *, *, #20957, .T. ) ;
#24211=EDGE_CURVE ( 'NONE', #11551, #15954, #19952, .T. ) ;
#24212=CARTESIAN_POINT ( 'NONE',  ( 157.4999999999994600, 213.7303124812313513, 45.00000000000000000 ) ) ;
#24214=EDGE_CURVE ( 'NONE', #4314, #5835, #8616, .T. ) ;
#24216=ORIENTED_EDGE ( 'NONE', *, *, #21988, .F. ) ;
#24218=CARTESIAN_POINT ( 'NONE',  ( 157.4999999999998010, 236.3011875487955251, 45.00000000000000000 ) ) ;
#24225=CARTESIAN_POINT ( 'NONE',  ( 157.4999999999998579, 123.4468122109788482, -45.00000000000000000 ) ) ;
#24226=PLANE ( 'NONE',  #7805 ) ;
#24231=DIRECTION ( 'NONE',  ( 0.8916010070293783896, -0.4528218681382319422, 0.000000000000000000 ) ) ;
#24238=AXIS2_PLACEMENT_3D ( 'NONE', #21152, #1473, #9961 ) ;
#24239=DIRECTION ( 'NONE',  ( -0.000000000000000000, -0.000000000000000000, -1.000000000000000000 ) ) ;
#24242=VERTEX_POINT ( 'NONE', #424 ) ;
#24248=ORIENTED_EDGE ( 'NONE', *, *, #22198, .F. ) ;
#24250=AXIS2_PLACEMENT_3D ( 'NONE', #22856, #3162, #19987 ) ;
#24252=ORIENTED_EDGE ( 'NONE', *, *, #3351, .T. ) ;
#24254=DIRECTION ( 'NONE',  ( 0.000000000000000000, -1.000000000000000000, 0.000000000000000000 ) ) ;
#24255=AXIS2_PLACEMENT_3D ( 'NONE', #21898, #2205, #19740 ) ;
#24261=DIRECTION ( 'NONE',  ( -0.000000000000000000, -0.000000000000000000, -1.000000000000000000 ) ) ;
#24263=CARTESIAN_POINT ( 'NONE',  ( 157.4999999999998579, 120.9389372034718093, 45.00000000000000000 ) ) ;
#24264=CARTESIAN_POINT ( 'NONE',  ( 158.0000000000016485, 48.46449948952110987, 45.00000000000000000 ) ) ;
#24268=VECTOR ( 'NONE', #35, 1000.000000000000000 ) ;
#24270=DIRECTION ( 'NONE',  ( -0.8916010070296935819, 0.4528218681376112165, 0.000000000000000000 ) ) ;
#24272=FACE_OUTER_BOUND ( 'NONE', #15220, .T. ) ;
#24274=ORIENTED_EDGE ( 'NONE', *, *, #20149, .F. ) ;
#24279=VERTEX_POINT ( 'NONE', #6531 ) ;
#24281=EDGE_CURVE ( 'NONE', #21312, #26943, #20093, .T. ) ;
#24283=ADVANCED_FACE ( 'NONE', ( #4433 ), #17943, .F. ) ;
#24287=VECTOR ( 'NONE', #24878, 1000.000000000000227 ) ;
#24294=CARTESIAN_POINT ( 'NONE',  ( 158.0000000000015064, 63.00387452705633251, 45.00000000000000000 ) ) ;
#24300=EDGE_CURVE ( 'NONE', #12920, #170, #3127, .T. ) ;
#24303=LINE ( 'NONE', #464, #21288 ) ;
#24308=CARTESIAN_POINT ( 'NONE',  ( 158.0000000000006537, 143.2558747672816821, 45.00000000000000000 ) ) ;
#24314=ORIENTED_EDGE ( 'NONE', *, *, #27982, .F. ) ;
#24320=DIRECTION ( 'NONE',  ( -0.8916010070296429557, -0.4528218681377111920, 0.000000000000000000 ) ) ;
#24323=CARTESIAN_POINT ( 'NONE',  ( 158.0000000000004263, 166.3346248423521274, -45.00000000000000000 ) ) ;
#24324=CARTESIAN_POINT ( 'NONE',  ( 158.0000000000014495, 68.01962454207041731, 45.00000000000000000 ) ) ;
#24325=EDGE_CURVE ( 'NONE', #11442, #24784, #7737, .T. ) ;
#24326=LINE ( 'NONE', #2481, #25155 ) ;
#24327=ADVANCED_FACE ( 'NONE', ( #5152 ), #22689, .F. ) ;
#24332=DIRECTION ( 'NONE',  ( -0.8916010070295719014, -0.4528218681378510246, 0.000000000000000000 ) ) ;
#24333=CARTESIAN_POINT ( 'NONE',  ( 157.4999999999998010, 236.3011875487955251, 45.00000000000000000 ) ) ;
#24337=FACE_OUTER_BOUND ( 'NONE', #11720, .T. ) ;
#24338=EDGE_LOOP ( 'NONE', ( #21424, #8343, #478, #16656 ) ) ;
#24339=CARTESIAN_POINT ( 'NONE',  ( 157.9999999999996589, 271.6653751576470768, -45.00000000000000000 ) ) ;
#24340=DIRECTION ( 'NONE',  ( 0.8916010070293383105, -0.4528218681383106015, 0.000000000000000000 ) ) ;
#24342=ORIENTED_EDGE ( 'NONE', *, *, #9290, .T. ) ;
#24343=FACE_OUTER_BOUND ( 'NONE', #3007, .T. ) ;
#24347=VERTEX_POINT ( 'NONE', #711 ) ;
#24349=ORIENTED_EDGE ( 'NONE', *, *, #15652, .T. ) ;
#24351=PLANE ( 'NONE',  #7638 ) ;
#24352=ORIENTED_EDGE ( 'NONE', *, *, #27948, .F. ) ;
#24354=ADVANCED_FACE ( 'NONE', ( #20806 ), #18094, .F. ) ;
#24356=ORIENTED_EDGE ( 'NONE', *, *, #14332, .F. ) ;
#24363=EDGE_CURVE ( 'NONE', #1132, #19895, #9757, .T. ) ;
#24364=DIRECTION ( 'NONE',  ( -0.8916010070294503320, -0.4528218681380901667, 0.000000000000000000 ) ) ;
#24372=DIRECTION ( 'NONE',  ( -0.000000000000000000, -0.000000000000000000, -1.000000000000000000 ) ) ;
#24374=VERTEX_POINT ( 'NONE', #3551 ) ;
#24378=DIRECTION ( 'NONE',  ( -0.000000000000000000, 0.000000000000000000, -1.000000000000000000 ) ) ;
#24381=CARTESIAN_POINT ( 'NONE',  ( 157.4999999999998579, 48.21056198576756202, 45.00000000000000000 ) ) ;
#24384=ORIENTED_EDGE ( 'NONE', *, *, #15315, .F. ) ;
#24386=VECTOR ( 'NONE', #918, 1000.000000000000000 ) ;
#24388=VERTEX_POINT ( 'NONE', #10453 ) ;
#24393=DIRECTION ( 'NONE',  ( 0.000000000000000000, -1.000000000000000000, 0.000000000000000000 ) ) ;
#24398=EDGE_CURVE ( 'NONE', #23789, #9022, #19073, .T. ) ;
#24400=DIRECTION ( 'NONE',  ( 0.000000000000000000, -1.000000000000000000, 0.000000000000000000 ) ) ;
#24404=EDGE_CURVE ( 'NONE', #13313, #14722, #5716, .T. ) ;
#24408=CARTESIAN_POINT ( 'NONE',  ( 157.4999999999998579, 166.0806873385985796, -45.00000000000000000 ) ) ;
#24409=ADVANCED_FACE ( 'NONE', ( #5996 ), #14772, .F. ) ;
#24415=VECTOR ( 'NONE', #20112, 1000.000000000000114 ) ;
#24425=ORIENTED_EDGE ( 'NONE', *, *, #25234, .F. ) ;
#24426=ORIENTED_EDGE ( 'NONE', *, *, #448, .T. ) ;
#24432=LINE ( 'NONE', #27010, #334 ) ;
#24434=AXIS2_PLACEMENT_3D ( 'NONE', #23995, #10780, #8762 ) ;
#24435=DIRECTION ( 'NONE',  ( 0.8916010070293584056, -0.4528218681382712996, 0.000000000000000000 ) ) ;
#24436=EDGE_LOOP ( 'NONE', ( #21868, #13374, #2362, #13815 ) ) ;
#24438=VECTOR ( 'NONE', #21228, 1000.000000000000114 ) ;
#24439=DIRECTION ( 'NONE',  ( -0.000000000000000000, -0.000000000000000000, -1.000000000000000000 ) ) ;
#24440=AXIS2_PLACEMENT_3D ( 'NONE', #8100, #6219, #19016 ) ;
#24443=ORIENTED_EDGE ( 'NONE', *, *, #28312, .F. ) ;
#24446=FACE_OUTER_BOUND ( 'NONE', #12157, .T. ) ;
#24448=DIRECTION ( 'NONE',  ( -0.000000000000000000, -0.000000000000000000, -1.000000000000000000 ) ) ;
#24455=DIRECTION ( 'NONE',  ( -0.000000000000000000, -0.000000000000000000, -1.000000000000000000 ) ) ;
#24458=ORIENTED_EDGE ( 'NONE', *, *, #22007, .F. ) ;
#24459=EDGE_CURVE ( 'NONE', #23572, #17489, #28243, .T. ) ;
#24460=AXIS2_PLACEMENT_3D ( 'NONE', #7437, #5129, #5409 ) ;
#24467=FACE_OUTER_BOUND ( 'NONE', #7817, .T. ) ;
#24469=VERTEX_POINT ( 'NONE', #248 ) ;
#24473=PLANE ( 'NONE',  #24575 ) ;
#24474=CARTESIAN_POINT ( 'NONE',  ( 158.0000000000006537, 143.2558747672816821, 45.00000000000000000 ) ) ;
#24477=FACE_OUTER_BOUND ( 'NONE', #21668, .T. ) ;
#24481=ADVANCED_FACE ( 'NONE', ( #21651 ), #24099, .F. ) ;
#24482=CARTESIAN_POINT ( 'NONE',  ( 158.0000000000015916, 55.48024950453520177, 45.00000000000000000 ) ) ;
#24483=LINE ( 'NONE', #19603, #7882 ) ;
#24486=ORIENTED_EDGE ( 'NONE', *, *, #8149, .T. ) ;
#24487=CARTESIAN_POINT ( 'NONE',  ( 157.9999999999999716, 210.9684999699701393, -45.00000000000000000 ) ) ;
#24492=ORIENTED_EDGE ( 'NONE', *, *, #10100, .T. ) ;
#24496=AXIS2_PLACEMENT_3D ( 'NONE', #7309, #5145, #976 ) ;
#24498=ORIENTED_EDGE ( 'NONE', *, *, #14243, .F. ) ;
#24504=EDGE_CURVE ( 'NONE', #2475, #8983, #17476, .T. ) ;
#24506=ORIENTED_EDGE ( 'NONE', *, *, #9614, .T. ) ;
#24507=EDGE_CURVE ( 'NONE', #23616, #15078, #22218, .T. ) ;
#24516=DIRECTION ( 'NONE',  ( -0.8916010070296327417, -0.4528218681377311761, 0.000000000000000000 ) ) ;
#24518=CARTESIAN_POINT ( 'NONE',  ( 157.9999999999997442, 251.6023750975910218, 45.00000000000000000 ) ) ;
#24520=CARTESIAN_POINT ( 'NONE',  ( 158.0000000000009663, 111.1613746771971876, -45.00000000000000000 ) ) ;
#24525=CARTESIAN_POINT ( 'NONE',  ( 157.4999999999995168, 208.7145624662163925, 45.00000000000000000 ) ) ;
#24526=DIRECTION ( 'NONE',  ( 1.000000000000000000, 0.000000000000000000, -0.000000000000000000 ) ) ;
#24538=ORIENTED_EDGE ( 'NONE', *, *, #28077, .F. ) ;
#24539=VECTOR ( 'NONE', #10430, 1000.000000000000000 ) ;
#24544=DIRECTION ( 'NONE',  ( 1.000000000000000000, 0.000000000000000000, -0.000000000000000000 ) ) ;
#24547=LINE ( 'NONE', #4856, #9587 ) ;
#24548=FACE_OUTER_BOUND ( 'NONE', #5362, .T. ) ;
#24549=DIRECTION ( 'NONE',  ( -0.000000000000000000, 0.000000000000000000, -1.000000000000000000 ) ) ;
#24552=DIRECTION ( 'NONE',  ( 0.000000000000000000, -1.000000000000000000, 0.000000000000000000 ) ) ;
#24553=CARTESIAN_POINT ( 'NONE',  ( 158.0000000000006537, 143.7637497747887210, -45.00000000000000000 ) ) ;
#24559=DIRECTION ( 'NONE',  ( -0.8916010070293682865, -0.4528218681382519262, 0.000000000000000000 ) ) ;
#24562=VERTEX_POINT ( 'NONE', #2241 ) ;
#24563=ORIENTED_EDGE ( 'NONE', *, *, #21511, .F. ) ;
#24564=FACE_OUTER_BOUND ( 'NONE', #22229, .T. ) ;
#24566=CARTESIAN_POINT ( 'NONE',  ( 157.9999999999999716, 210.9684999699701393, -45.00000000000000000 ) ) ;
#24567=ORIENTED_EDGE ( 'NONE', *, *, #6660, .T. ) ;
#24568=ORIENTED_EDGE ( 'NONE', *, *, #3892, .T. ) ;
#24574=ORIENTED_EDGE ( 'NONE', *, *, #486, .F. ) ;
#24575=AXIS2_PLACEMENT_3D ( 'NONE', #11562, #633, #24763 ) ;
#24576=ORIENTED_EDGE ( 'NONE', *, *, #13984, .T. ) ;
#24579=CARTESIAN_POINT ( 'NONE',  ( 157.4999999999998579, 100.8759371434154701, -45.00000000000000000 ) ) ;
#24581=DIRECTION ( 'NONE',  ( -0.000000000000000000, -0.000000000000000000, -1.000000000000000000 ) ) ;
#24582=VECTOR ( 'NONE', #25295, 1000.000000000000000 ) ;
#24583=LINE ( 'NONE', #16116, #15322 ) ;
#24585=LINE ( 'NONE', #13683, #22374 ) ;
#24592=CARTESIAN_POINT ( 'NONE',  ( 157.9999999999997726, 244.0787500750700474, 45.00000000000000000 ) ) ;
#24594=ORIENTED_EDGE ( 'NONE', *, *, #15688, .F. ) ;
#24595=VECTOR ( 'NONE', #7650, 1000.000000000000114 ) ;
#24597=EDGE_CURVE ( 'NONE', #7010, #4812, #23813, .T. ) ;
#24599=CARTESIAN_POINT ( 'NONE',  ( 157.9999999999997726, 248.5866250825770294, -45.00000000000000000 ) ) ;
#24600=ORIENTED_EDGE ( 'NONE', *, *, #7483, .F. ) ;
#24602=CONICAL_SURFACE ( 'NONE', #738, 6.000000000000005329, 1.029744258676651647 ) ;
#24605=CARTESIAN_POINT ( 'NONE',  ( 158.0000000000000568, 203.4448749474510407, -45.00000000000000000 ) ) ;
#24606=EDGE_CURVE ( 'NONE', #378, #7332, #26239, .T. ) ;
#24611=CARTESIAN_POINT ( 'NONE',  ( 157.4999999999995737, 203.6988124512014338, 45.00000000000000000 ) ) ;
#24613=LINE ( 'NONE', #2767, #17396 ) ;
#24614=ORIENTED_EDGE ( 'NONE', *, *, #17829, .F. ) ;
#24615=AXIS2_PLACEMENT_3D ( 'NONE', #19195, #27940, #19336 ) ;
#24618=CARTESIAN_POINT ( 'NONE',  ( 157.4999999999998579, 83.32081209086616980, 45.00000000000000000 ) ) ;
#24622=EDGE_CURVE ( 'NONE', #3041, #21312, #27093, .T. ) ;
#24623=CARTESIAN_POINT ( 'NONE',  ( 158.0000000000007390, 133.7322497447605656, 45.00000000000000000 ) ) ;
#24624=CARTESIAN_POINT ( 'NONE',  ( 158.0000000000012790, 85.57474959461971764, 45.00000000000000000 ) ) ;
#24630=ORIENTED_EDGE ( 'NONE', *, *, #25986, .T. ) ;
#24633=EDGE_CURVE ( 'NONE', #543, #6469, #11752, .T. ) ;
#24634=LINE ( 'NONE', #216, #19403 ) ;
#24638=CARTESIAN_POINT ( 'NONE',  ( 157.4999999999998579, 78.30506207585207790, 45.00000000000000000 ) ) ;
#24641=VECTOR ( 'NONE', #16180, 1000.000000000000000 ) ;
#24642=DIRECTION ( 'NONE',  ( 0.8916010070295005141, -0.4528218681379915789, 0.000000000000000000 ) ) ;
#24644=DIRECTION ( 'NONE',  ( -0.000000000000000000, -0.000000000000000000, -1.000000000000000000 ) ) ;
#24649=EDGE_LOOP ( 'NONE', ( #8425, #18744, #14829, #10188 ) ) ;
#24654=CARTESIAN_POINT ( 'NONE',  ( 158.0000000000003411, 175.8582498648732440, -45.00000000000000000 ) ) ;
#24657=EDGE_CURVE ( 'NONE', #11940, #4647, #9294, .T. ) ;
#24658=CARTESIAN_POINT ( 'NONE',  ( 158.0000000000006537, 145.7637497747887210, 45.00000000000000000 ) ) ;
#24663=CARTESIAN_POINT ( 'NONE',  ( 157.4999999999998579, 176.1121873686267350, 45.00000000000000000 ) ) ;
#24664=PLANE ( 'NONE',  #843 ) ;
#24665=DIRECTION ( 'NONE',  ( 0.000000000000000000, -1.000000000000000000, 0.000000000000000000 ) ) ;
#24666=VERTEX_POINT ( 'NONE', #24518 ) ;
#24668=EDGE_CURVE ( 'NONE', #26578, #25616, #16198, .T. ) ;
#24669=PLANE ( 'NONE',  #26581 ) ;
#24671=EDGE_CURVE ( 'NONE', #28009, #3903, #2961, .T. ) ;
#24675=CARTESIAN_POINT ( 'NONE',  ( 157.4999999999996874, 271.4114376538935289, 45.00000000000000000 ) ) ;
#24676=ORIENTED_EDGE ( 'NONE', *, *, #21926, .T. ) ;
#24678=VECTOR ( 'NONE', #13929, 999.9999999999998863 ) ;
#24679=ORIENTED_EDGE ( 'NONE', *, *, #3438, .T. ) ;
#24680=ORIENTED_EDGE ( 'NONE', *, *, #12229, .F. ) ;
#24681=EDGE_CURVE ( 'NONE', #27184, #1982, #389, .T. ) ;
#24682=ORIENTED_EDGE ( 'NONE', *, *, #25300, .F. ) ;
#24687=LINE ( 'NONE', #23100, #25225 ) ;
#24691=AXIS2_PLACEMENT_3D ( 'NONE', #8017, #16644, #25258 ) ;
#24695=AXIS2_PLACEMENT_3D ( 'NONE', #1747, #21008, #8085 ) ;
#24697=LINE ( 'NONE', #1886, #8767 ) ;
#24698=CARTESIAN_POINT ( 'NONE',  ( 158.0000000000008527, 123.7007497147323960, -45.00000000000000000 ) ) ;
#24705=DIRECTION ( 'NONE',  ( -0.8916010070298151513, 0.4528218681373720744, 0.000000000000000000 ) ) ;
#24708=ORIENTED_EDGE ( 'NONE', *, *, #12321, .F. ) ;
#24710=PLANE ( 'NONE',  #14343 ) ;
#24712=ORIENTED_EDGE ( 'NONE', *, *, #14332, .T. ) ;
#24724=CARTESIAN_POINT ( 'NONE',  ( 158.0000000000001705, 188.9054999099155054, 45.00000000000000000 ) ) ;
#24725=ORIENTED_EDGE ( 'NONE', *, *, #20136, .T. ) ;
#24728=VECTOR ( 'NONE', #16262, 1000.000000000000000 ) ;
#24730=ADVANCED_FACE ( 'NONE', ( #22796 ), #9444, .F. ) ;
#24731=DIRECTION ( 'NONE',  ( -0.8916010070297440970, 0.4528218681375119625, 0.000000000000000000 ) ) ;
#24735=DIRECTION ( 'NONE',  ( -0.8916010070299780210, -0.4528218681370510534, 0.000000000000000000 ) ) ;
#24739=CARTESIAN_POINT ( 'NONE',  ( 157.4999999999998579, 133.4783122410070462, 45.00000000000000000 ) ) ;
#24741=ORIENTED_EDGE ( 'NONE', *, *, #18472, .T. ) ;
#24742=VECTOR ( 'NONE', #4363, 1000.000000000000000 ) ;
#24747=VERTEX_POINT ( 'NONE', #3820 ) ;
#24751=ORIENTED_EDGE ( 'NONE', *, *, #22068, .F. ) ;
#24752=AXIS2_PLACEMENT_3D ( 'NONE', #24899, #7086, #7375 ) ;
#24754=CARTESIAN_POINT ( 'NONE',  ( 157.4999999999998579, 98.36806213590843129, 45.00000000000000000 ) ) ;
#24758=CARTESIAN_POINT ( 'NONE',  ( 157.4999999999998295, 40.68693696324645970, -45.00000000000000000 ) ) ;
#24759=ORIENTED_EDGE ( 'NONE', *, *, #14985, .T. ) ;
#24760=DIRECTION ( 'NONE',  ( 0.8916010070293483025, 0.4528218681382912836, 0.000000000000000000 ) ) ;
#24763=DIRECTION ( 'NONE',  ( -0.000000000000000000, 0.000000000000000000, -1.000000000000000000 ) ) ;
#24764=DIRECTION ( 'NONE',  ( 1.000000000000000000, 0.000000000000000000, -0.000000000000000000 ) ) ;
#24772=ADVANCED_FACE ( 'NONE', ( #17037 ), #5701, .F. ) ;
#24774=CARTESIAN_POINT ( 'NONE',  ( 157.4999999999998579, 158.5570623160774630, 45.00000000000000000 ) ) ;
#24775=LINE ( 'NONE', #24914, #176 ) ;
#24776=ORIENTED_EDGE ( 'NONE', *, *, #17648, .F. ) ;
#24779=ORIENTED_EDGE ( 'NONE', *, *, #21129, .F. ) ;
#24780=ADVANCED_FACE ( 'NONE', ( #18910 ), #8137, .F. ) ;
#24784=VERTEX_POINT ( 'NONE', #14607 ) ;
#24786=ORIENTED_EDGE ( 'NONE', *, *, #24823, .F. ) ;
#24788=VERTEX_POINT ( 'NONE', #23089 ) ;
#24792=CARTESIAN_POINT ( 'NONE',  ( 158.0000000000017053, 45.44874947450702507, 45.00000000000000000 ) ) ;
#24800=LINE ( 'NONE', #24654, #8038 ) ;
#24801=CARTESIAN_POINT ( 'NONE',  ( 158.0000000000007390, 133.7322497447605656, 45.00000000000000000 ) ) ;
#24804=FACE_OUTER_BOUND ( 'NONE', #2202, .T. ) ;
#24805=CARTESIAN_POINT ( 'NONE',  ( 157.4999999999998579, 45.70268697826052318, -45.00000000000000000 ) ) ;
#24810=EDGE_LOOP ( 'NONE', ( #4984, #26224, #10301, #25158 ) ) ;
#24811=CARTESIAN_POINT ( 'NONE',  ( 158.0000000000017053, 43.44874947450702507, 45.00000000000000000 ) ) ;
#24814=EDGE_CURVE ( 'NONE', #17184, #4162, #14899, .T. ) ;
#24817=PLANE ( 'NONE',  #18880 ) ;
#24819=VECTOR ( 'NONE', #15630, 1000.000000000000000 ) ;
#24821=ORIENTED_EDGE ( 'NONE', *, *, #21315, .T. ) ;
#24823=EDGE_CURVE ( 'NONE', #17780, #14086, #5976, .T. ) ;
#24835=CARTESIAN_POINT ( 'NONE',  ( 157.4999999999998579, 55.73418700828869277, 45.00000000000000000 ) ) ;
#24838=CARTESIAN_POINT ( 'NONE',  ( 157.9999999999998010, 239.0630000600560550, 45.00000000000000000 ) ) ;
#24847=LINE ( 'NONE', #22260, #5179 ) ;
#24848=EDGE_LOOP ( 'NONE', ( #5950, #9057, #16405, #18185 ) ) ;
#24849=ORIENTED_EDGE ( 'NONE', *, *, #5827, .T. ) ;
#24850=DIRECTION ( 'NONE',  ( 1.000000000000000000, 0.000000000000000000, -0.000000000000000000 ) ) ;
#24851=AXIS2_PLACEMENT_3D ( 'NONE', #26240, #13328, #20205 ) ;
#24854=VECTOR ( 'NONE', #28218, 1000.000000000000000 ) ;
#24855=EDGE_LOOP ( 'NONE', ( #24883, #18423, #20854, #27038 ) ) ;
#24857=CARTESIAN_POINT ( 'NONE',  ( 157.4999999999998579, 148.5255622860493077, 45.00000000000000000 ) ) ;
#24863=EDGE_CURVE ( 'NONE', #18505, #23832, #12606, .T. ) ;
#24868=AXIS2_PLACEMENT_3D ( 'NONE', #5650, #8229, #10385 ) ;
#24869=DIRECTION ( 'NONE',  ( 0.8916010070298252543, -0.4528218681373520904, 0.000000000000000000 ) ) ;
#24870=VECTOR ( 'NONE', #15997, 1000.000000000000000 ) ;
#24874=DIRECTION ( 'NONE',  ( -0.8916010070293384215, 0.4528218681383106015, 0.000000000000000000 ) ) ;
#24875=FACE_OUTER_BOUND ( 'NONE', #2190, .T. ) ;
#24878=DIRECTION ( 'NONE',  ( 0.8916010070296936929, -0.4528218681376112165, 0.000000000000000000 ) ) ;
#24879=EDGE_CURVE ( 'NONE', #4884, #13125, #6123, .T. ) ;
#24882=VERTEX_POINT ( 'NONE', #1801 ) ;
#24883=ORIENTED_EDGE ( 'NONE', *, *, #22661, .T. ) ;
#24885=DIRECTION ( 'NONE',  ( 0.000000000000000000, -1.000000000000000000, 0.000000000000000000 ) ) ;
#24886=PLANE ( 'NONE',  #1638 ) ;
#24889=VECTOR ( 'NONE', #13377, 1000.000000000000000 ) ;
#24890=EDGE_LOOP ( 'NONE', ( #2093, #19546, #26263, #12752 ) ) ;
#24893=VECTOR ( 'NONE', #20534, 1000.000000000000000 ) ;
#24895=DIRECTION ( 'NONE',  ( -0.8916010070295922185, -0.4528218681378110566, 0.000000000000000000 ) ) ;
#24896=ADVANCED_FACE ( 'NONE', ( #228 ), #17458, .F. ) ;
#24899=CARTESIAN_POINT ( 'NONE',  ( 158.0000000000015916, 55.48024950453520177, 45.00000000000000000 ) ) ;
#24902=LINE ( 'NONE', #5070, #25489 ) ;
#24905=CARTESIAN_POINT ( 'NONE',  ( 158.0000000000009095, 118.6849996997183041, 45.00000000000000000 ) ) ;
#24907=LINE ( 'NONE', #27052, #23902 ) ;
#24908=CARTESIAN_POINT ( 'NONE',  ( 158.0000000000000284, 205.9527499549551806, 45.00000000000000000 ) ) ;
#24911=DIRECTION ( 'NONE',  ( 0.8916010070293384215, 0.4528218681383106015, 0.000000000000000000 ) ) ;
#24914=CARTESIAN_POINT ( 'NONE',  ( 157.9999999999998295, 226.0157500150140208, 45.00000000000000000 ) ) ;
#24917=ORIENTED_EDGE ( 'NONE', *, *, #15070, .T. ) ;
#24918=DIRECTION ( 'NONE',  ( -0.000000000000000000, -0.000000000000000000, -1.000000000000000000 ) ) ;
#24921=DIRECTION ( 'NONE',  ( 0.4528218681370511089, -0.8916010070299782431, 0.000000000000000000 ) ) ;
#24937=VERTEX_POINT ( 'NONE', #6545 ) ;
#24938=VECTOR ( 'NONE', #28379, 1000.000000000000000 ) ;
#24942=DIRECTION ( 'NONE',  ( 0.8916010070299273949, 0.4528218681371510290, 0.000000000000000000 ) ) ;
#24945=CARTESIAN_POINT ( 'NONE',  ( 158.0000000000002842, 180.8739998798873501, 45.00000000000000000 ) ) ;
#24948=CARTESIAN_POINT ( 'NONE',  ( 158.0000000000011084, 100.6219996396619791, 45.00000000000000000 ) ) ;
#24950=VERTEX_POINT ( 'NONE', #4243 ) ;
#24952=VECTOR ( 'NONE', #7070, 1000.000000000000227 ) ;
#24958=EDGE_CURVE ( 'NONE', #1444, #1356, #19333, .T. ) ;
#24961=LINE ( 'NONE', #22809, #1740 ) ;
#24963=ORIENTED_EDGE ( 'NONE', *, *, #1149, .T. ) ;
#24971=EDGE_CURVE ( 'NONE', #15116, #3105, #22056, .T. ) ;
#24973=EDGE_CURVE ( 'NONE', #13125, #15105, #15467, .T. ) ;
#24974=VECTOR ( 'NONE', #19573, 1000.000000000000000 ) ;
#24977=CARTESIAN_POINT ( 'NONE',  ( 158.0000000000013358, 80.55899957960563995, 45.00000000000000000 ) ) ;
#24981=CARTESIAN_POINT ( 'NONE',  ( 157.4999999999998579, 90.84443711338730054, 45.00000000000000000 ) ) ;
#24983=ADVANCED_FACE ( 'NONE', ( #21915 ), #8703, .F. ) ;
#24987=DIRECTION ( 'NONE',  ( -0.000000000000000000, -0.000000000000000000, -1.000000000000000000 ) ) ;
#24988=ORIENTED_EDGE ( 'NONE', *, *, #11907, .T. ) ;
#24998=ORIENTED_EDGE ( 'NONE', *, *, #3738, .T. ) ;
#25000=CARTESIAN_POINT ( 'NONE',  ( 158.0000000000010800, 101.1298746471690038, 45.00000000000000000 ) ) ;
#25001=FACE_OUTER_BOUND ( 'NONE', #19118, .T. ) ;
#25002=EDGE_CURVE ( 'NONE', #23711, #20791, #18184, .T. ) ;
#25003=EDGE_CURVE ( 'NONE', #14031, #3490, #11730, .T. ) ;
#25005=VECTOR ( 'NONE', #18198, 1000.000000000000000 ) ;
#25007=VECTOR ( 'NONE', #24869, 1000.000000000000114 ) ;
#25009=CARTESIAN_POINT ( 'NONE',  ( 157.4999999999998010, 238.8090625563025071, 45.00000000000000000 ) ) ;
#25013=EDGE_CURVE ( 'NONE', #23789, #4844, #11295, .T. ) ;
#25014=PLANE ( 'NONE',  #24250 ) ;
#25015=CARTESIAN_POINT ( 'NONE',  ( 157.4999999999998579, 223.7618125112605298, 45.00000000000000000 ) ) ;
#25016=LINE ( 'NONE', #9653, #13427 ) ;
#25017=PLANE ( 'NONE',  #9374 ) ;
#25018=ORIENTED_EDGE ( 'NONE', *, *, #19877, .T. ) ;
#25019=ADVANCED_FACE ( 'NONE', ( #13887 ), #11592, .F. ) ;
#25024=ORIENTED_EDGE ( 'NONE', *, *, #6300, .F. ) ;
#25027=ADVANCED_FACE ( 'NONE', ( #7407 ), #15752, .F. ) ;
#25030=LINE ( 'NONE', #20431, #6033 ) ;
#25031=PLANE ( 'NONE',  #19547 ) ;
#25032=ORIENTED_EDGE ( 'NONE', *, *, #10620, .F. ) ;
#25034=ORIENTED_EDGE ( 'NONE', *, *, #20216, .F. ) ;
#25037=DIRECTION ( 'NONE',  ( -0.000000000000000000, -0.000000000000000000, -1.000000000000000000 ) ) ;
#25039=ADVANCED_FACE ( 'NONE', ( #13593 ), #26938, .F. ) ;
#25044=VECTOR ( 'NONE', #25175, 1000.000000000000000 ) ;
#25047=VECTOR ( 'NONE', #5110, 1000.000000000000000 ) ;
#25048=LINE ( 'NONE', #13863, #2221 ) ;
#25050=PLANE ( 'NONE',  #8110 ) ;
#25052=CARTESIAN_POINT ( 'NONE',  ( 157.4999999999998579, 60.74993702330277756, 45.00000000000000000 ) ) ;
#25054=CARTESIAN_POINT ( 'NONE',  ( 157.9999999999997726, 248.5866250825770294, 45.00000000000000000 ) ) ;
#25055=CARTESIAN_POINT ( 'NONE',  ( 157.4999999999997442, 256.3641876088515232, 45.00000000000000000 ) ) ;
#25056=ORIENTED_EDGE ( 'NONE', *, *, #6019, .T. ) ;
#25064=ORIENTED_EDGE ( 'NONE', *, *, #17321, .F. ) ;
#25065=CARTESIAN_POINT ( 'NONE',  ( 0.000000000000000000, 0.000000000000000000, 0.000000000000000000 ) ) ;
#25067=ORIENTED_EDGE ( 'NONE', *, *, #25462, .T. ) ;
#25072=ORIENTED_EDGE ( 'NONE', *, *, #13852, .T. ) ;
#25078=DIRECTION ( 'NONE',  ( -0.000000000000000000, -0.000000000000000000, -1.000000000000000000 ) ) ;
#25080=LINE ( 'NONE', #3087, #27515 ) ;
#25081=CARTESIAN_POINT ( 'NONE',  ( 158.0000000000005400, 155.7952498048169048, 45.00000000000000000 ) ) ;
#25083=DIRECTION ( 'NONE',  ( 1.000000000000000000, 0.000000000000000000, -0.000000000000000000 ) ) ;
#25087=PLANE ( 'NONE',  #28129 ) ;
#25088=AXIS2_PLACEMENT_3D ( 'NONE', #24792, #27078, #5247 ) ;
#25089=ORIENTED_EDGE ( 'NONE', *, *, #26538, .F. ) ;
#25092=LINE ( 'NONE', #25508, #20627 ) ;
#25098=DIRECTION ( 'NONE',  ( 0.8916010070295922185, -0.4528218681378110566, 0.000000000000000000 ) ) ;
#25099=ORIENTED_EDGE ( 'NONE', *, *, #14307, .F. ) ;
#25101=ORIENTED_EDGE ( 'NONE', *, *, #18993, .T. ) ;
#25104=VECTOR ( 'NONE', #6049, 1000.000000000000114 ) ;
#25106=CARTESIAN_POINT ( 'NONE',  ( 158.0000000000015348, 58.49599951954928656, 45.00000000000000000 ) ) ;
#25109=CARTESIAN_POINT ( 'NONE',  ( 157.9999999999998010, 234.0472500450420341, -45.00000000000000000 ) ) ;
#25110=EDGE_CURVE ( 'NONE', #4442, #1347, #7687, .T. ) ;
#25113=CARTESIAN_POINT ( 'NONE',  ( 157.4999999999998579, 85.82868709837320864, 45.00000000000000000 ) ) ;
#25117=ORIENTED_EDGE ( 'NONE', *, *, #20047, .T. ) ;
#25118=EDGE_CURVE ( 'NONE', #26005, #23503, #3501, .T. ) ;
#25121=DIRECTION ( 'NONE',  ( -0.8916010070294098089, -0.4528218681381701027, 0.000000000000000000 ) ) ;
#25122=ORIENTED_EDGE ( 'NONE', *, *, #21887, .F. ) ;
#25125=ADVANCED_FACE ( 'NONE', ( #27625 ), #25201, .F. ) ;
#25126=CARTESIAN_POINT ( 'NONE',  ( 158.0000000000007390, 135.7322497447605656, 45.00000000000000000 ) ) ;
#25130=ORIENTED_EDGE ( 'NONE', *, *, #27716, .T. ) ;
#25131=ORIENTED_EDGE ( 'NONE', *, *, #17487, .F. ) ;
#25133=EDGE_CURVE ( 'NONE', #11334, #4392, #27484, .T. ) ;
#25137=CARTESIAN_POINT ( 'NONE',  ( 157.9999999999996305, 281.6968751876750616, 45.00000000000000000 ) ) ;
#25138=DIRECTION ( 'NONE',  ( 0.000000000000000000, -1.000000000000000000, 0.000000000000000000 ) ) ;
#25142=PLANE ( 'NONE',  #1325 ) ;
#25151=CONICAL_SURFACE ( 'NONE', #394, 6.000000000000005329, 1.029744258676651647 ) ;
#25152=ADVANCED_FACE ( 'NONE', ( #10400 ), #25614, .F. ) ;
#25155=VECTOR ( 'NONE', #3834, 1000.000000000000000 ) ;
#25157=VERTEX_POINT ( 'NONE', #19156 ) ;
#25158=ORIENTED_EDGE ( 'NONE', *, *, #21099, .T. ) ;
#25159=DIRECTION ( 'NONE',  ( -0.000000000000000000, -0.000000000000000000, -1.000000000000000000 ) ) ;
#25160=DIRECTION ( 'NONE',  ( -0.000000000000000000, -0.000000000000000000, -1.000000000000000000 ) ) ;
#25161=VERTEX_POINT ( 'NONE', #27899 ) ;
#25172=CARTESIAN_POINT ( 'NONE',  ( 157.4999999999998579, 63.25781203080982351, 45.00000000000000000 ) ) ;
#25174=VECTOR ( 'NONE', #14102, 1000.000000000000000 ) ;
#25175=DIRECTION ( 'NONE',  ( -0.000000000000000000, -0.000000000000000000, -1.000000000000000000 ) ) ;
#25176=EDGE_CURVE ( 'NONE', #13244, #6317, #21169, .T. ) ;
#25177=CARTESIAN_POINT ( 'NONE',  ( 157.4999999999998579, 68.27356204582390831, 45.00000000000000000 ) ) ;
#25179=DIRECTION ( 'NONE',  ( -0.8916010070293584056, 0.4528218681382713551, 0.000000000000000000 ) ) ;
#25182=CARTESIAN_POINT ( 'NONE',  ( 158.0000000000007674, 133.2243747372535267, 45.00000000000000000 ) ) ;
#25183=ORIENTED_EDGE ( 'NONE', *, *, #23421, .F. ) ;
#25184=CARTESIAN_POINT ( 'NONE',  ( 157.4999999999998579, 93.35231212089433939, -45.00000000000000000 ) ) ;
#25186=LINE ( 'NONE', #14424, #2011 ) ;
#25188=CARTESIAN_POINT ( 'NONE',  ( 158.0000000000014495, 66.01962454207041731, 45.00000000000000000 ) ) ;
#25190=VECTOR ( 'NONE', #24068, 1000.000000000000000 ) ;
#25191=LINE ( 'NONE', #14291, #615 ) ;
#25194=VERTEX_POINT ( 'NONE', #9840 ) ;
#25195=FACE_OUTER_BOUND ( 'NONE', #5754, .T. ) ;
#25201=PLANE ( 'NONE',  #2555 ) ;
#25204=VECTOR ( 'NONE', #9504, 1000.000000000000114 ) ;
#25207=EDGE_LOOP ( 'NONE', ( #1985, #8596, #1521, #24066 ) ) ;
#25208=ORIENTED_EDGE ( 'NONE', *, *, #23533, .F. ) ;
#25210=PLANE ( 'NONE',  #9762 ) ;
#25214=MECHANICAL_DESIGN_GEOMETRIC_PRESENTATION_REPRESENTATION('',(#17353),#7280);
#25216=CARTESIAN_POINT ( 'NONE',  ( 158.0000000000016485, 50.46449948952111697, 45.00000000000000000 ) ) ;
#25224=VERTEX_POINT ( 'NONE', #2613 ) ;
#25225=VECTOR ( 'NONE', #9608, 1000.000000000000000 ) ;
#25230=DIRECTION ( 'NONE',  ( 0.4528218681383056610, -0.8916010070293409751, 0.000000000000000000 ) ) ;
#25232=CARTESIAN_POINT ( 'NONE',  ( 157.4999999999998579, 88.33656210588026170, -45.00000000000000000 ) ) ;
#25234=EDGE_CURVE ( 'NONE', #24788, #8797, #9385, .T. ) ;
#25238=VECTOR ( 'NONE', #12370, 1000.000000000000000 ) ;
#25239=VERTEX_POINT ( 'NONE', #24605 ) ;
#25240=VECTOR ( 'NONE', #9501, 999.9999999999998863 ) ;
#25241=ORIENTED_EDGE ( 'NONE', *, *, #11806, .F. ) ;
#25243=ORIENTED_EDGE ( 'NONE', *, *, #26940, .T. ) ;
#25244=CARTESIAN_POINT ( 'NONE',  ( 158.0000000000005969, 150.7794997898028271, -45.00000000000000000 ) ) ;
#25247=EDGE_CURVE ( 'NONE', #21808, #12783, #13409, .T. ) ;
#25249=ADVANCED_FACE ( 'NONE', ( #17849 ), #24886, .F. ) ;
#25254=AXIS2_PLACEMENT_3D ( 'NONE', #16050, #1086, #24942 ) ;
#25258=DIRECTION ( 'NONE',  ( 0.8916010070293783896, 0.4528218681382319422, 0.000000000000000000 ) ) ;
#25260=EDGE_LOOP ( 'NONE', ( #4020, #7644, #25034, #20362 ) ) ;
#25265=ORIENTED_EDGE ( 'NONE', *, *, #27186, .T. ) ;
#25272=AXIS2_PLACEMENT_3D ( 'NONE', #14139, #7242, #16294 ) ;
#25273=EDGE_LOOP ( 'NONE', ( #582, #24274, #20318, #3704 ) ) ;
#25277=VECTOR ( 'NONE', #25993, 1000.000000000000000 ) ;
#25282=EDGE_CURVE ( 'NONE', #17145, #5416, #27035, .T. ) ;
#25290=LINE ( 'NONE', #10213, #18473 ) ;
#25293=LINE ( 'NONE', #3450, #2273 ) ;
#25294=VECTOR ( 'NONE', #25968, 1000.000000000000114 ) ;
#25295=DIRECTION ( 'NONE',  ( 0.000000000000000000, -1.000000000000000000, 0.000000000000000000 ) ) ;
#25299=ORIENTED_EDGE ( 'NONE', *, *, #7391, .F. ) ;
#25300=EDGE_CURVE ( 'NONE', #7477, #5352, #9236, .T. ) ;
#25302=DIRECTION ( 'NONE',  ( 0.8916010070293383105, -0.4528218681383106015, 0.000000000000000000 ) ) ;
#25304=ORIENTED_EDGE ( 'NONE', *, *, #3333, .T. ) ;
#25306=AXIS2_PLACEMENT_3D ( 'NONE', #27750, #14561, #23316 ) ;
#25314=CARTESIAN_POINT ( 'NONE',  ( 157.4999999999998579, 50.71843699327460797, -45.00000000000000000 ) ) ;
#25318=DIRECTION ( 'NONE',  ( 0.4528218681373508692, -0.8916010070298259205, 0.000000000000000000 ) ) ;
#25325=LINE ( 'NONE', #6064, #15537 ) ;
#25327=PLANE ( 'NONE',  #25306 ) ;
#25328=LINE ( 'NONE', #5652, #660 ) ;
#25329=ORIENTED_EDGE ( 'NONE', *, *, #12091, .T. ) ;
#25331=CARTESIAN_POINT ( 'NONE',  ( 157.4999999999996305, 286.4586876989355915, 45.00000000000000000 ) ) ;
#25340=AXIS2_PLACEMENT_3D ( 'NONE', #6753, #10931, #4451 ) ;
#25341=ORIENTED_EDGE ( 'NONE', *, *, #2643, .F. ) ;
#25342=VECTOR ( 'NONE', #25410, 1000.000000000000000 ) ;
#25344=CARTESIAN_POINT ( 'NONE',  ( 157.4999999999998579, 53.22631200078164682, 45.00000000000000000 ) ) ;
#25346=EDGE_LOOP ( 'NONE', ( #18243, #7724, #9914, #20193 ) ) ;
#25349=ORIENTED_EDGE ( 'NONE', *, *, #19028, .F. ) ;
#25355=EDGE_CURVE ( 'NONE', #15447, #3282, #27308, .T. ) ;
#25358=CARTESIAN_POINT ( 'NONE',  ( 158.0000000000005400, 155.7952498048169048, 45.00000000000000000 ) ) ;
#25361=LINE ( 'NONE', #8403, #26166 ) ;
#25364=PLANE ( 'NONE',  #1221 ) ;
#25368=VERTEX_POINT ( 'NONE', #18698 ) ;
#25369=CARTESIAN_POINT ( 'NONE',  ( 157.4999999999998579, 148.5255622860493077, -45.00000000000000000 ) ) ;
#25372=CARTESIAN_POINT ( 'NONE',  ( 158.0000000000005400, 153.7952498048169048, 45.00000000000000000 ) ) ;
#25375=EDGE_CURVE ( 'NONE', #23503, #19001, #12251, .T. ) ;
#25380=VERTEX_POINT ( 'NONE', #5901 ) ;
#25384=VECTOR ( 'NONE', #23674, 1000.000000000000114 ) ;
#25385=ORIENTED_EDGE ( 'NONE', *, *, #9977, .F. ) ;
#25389=CARTESIAN_POINT ( 'NONE',  ( 158.0000000000008242, 126.2086247222394206, -45.00000000000000000 ) ) ;
#25391=CARTESIAN_POINT ( 'NONE',  ( 157.9999999999996305, 288.7126252026890256, -45.00000000000000000 ) ) ;
#25396=VECTOR ( 'NONE', #13851, 1000.000000000000000 ) ;
#25397=DIRECTION ( 'NONE',  ( -0.000000000000000000, 0.000000000000000000, -1.000000000000000000 ) ) ;
#25399=VECTOR ( 'NONE', #19885, 1000.000000000000114 ) ;
#25400=DIRECTION ( 'NONE',  ( -0.000000000000000000, 0.000000000000000000, -1.000000000000000000 ) ) ;
#25401=CARTESIAN_POINT ( 'NONE',  ( 157.9999999999998010, 239.0630000600560550, -45.00000000000000000 ) ) ;
#25402=CARTESIAN_POINT ( 'NONE',  ( 157.9999999999998295, 224.0157500150140208, -45.00000000000000000 ) ) ;
#25403=VERTEX_POINT ( 'NONE', #9804 ) ;
#25408=ORIENTED_EDGE ( 'NONE', *, *, #7391, .T. ) ;
#25410=DIRECTION ( 'NONE',  ( 0.000000000000000000, -1.000000000000000000, 0.000000000000000000 ) ) ;
#25411=EDGE_CURVE ( 'NONE', #5026, #3340, #27582, .T. ) ;
#25413=ORIENTED_EDGE ( 'NONE', *, *, #24507, .T. ) ;
#25414=VECTOR ( 'NONE', #13643, 1000.000000000000000 ) ;
#25417=VECTOR ( 'NONE', #9078, 1000.000000000000000 ) ;
#25418=ORIENTED_EDGE ( 'NONE', *, *, #26538, .T. ) ;
#25419=ORIENTED_EDGE ( 'NONE', *, *, #9125, .T. ) ;
#25424=CARTESIAN_POINT ( 'NONE',  ( 158.0000000000005969, 150.7794997898028271, 45.00000000000000000 ) ) ;
#25426=LINE ( 'NONE', #1013, #13457 ) ;
#25432=CARTESIAN_POINT ( 'NONE',  ( 157.4999999999997442, 251.3484375938375024, -45.00000000000000000 ) ) ;
#25433=AXIS2_PLACEMENT_3D ( 'NONE', #11470, #18353, #397 ) ;
#25436=EDGE_CURVE ( 'NONE', #20816, #16250, #11967, .T. ) ;
#25437=EDGE_CURVE ( 'NONE', #28117, #24036, #10224, .T. ) ;
#25439=ORIENTED_EDGE ( 'NONE', *, *, #924, .T. ) ;
#25440=EDGE_LOOP ( 'NONE', ( #24426, #18808, #18279, #22326 ) ) ;
#25441=ORIENTED_EDGE ( 'NONE', *, *, #13823, .T. ) ;
#25444=ORIENTED_EDGE ( 'NONE', *, *, #16660, .T. ) ;
#25447=PLANE ( 'NONE',  #2147 ) ;
#25451=ORIENTED_EDGE ( 'NONE', *, *, #11403, .T. ) ;
#25454=DIRECTION ( 'NONE',  ( -0.000000000000000000, -0.000000000000000000, -1.000000000000000000 ) ) ;
#25455=CARTESIAN_POINT ( 'NONE',  ( 157.4999999999996874, 268.9035626463865469, 45.00000000000000000 ) ) ;
#25456=DIRECTION ( 'NONE',  ( 0.8916010070293783896, -0.4528218681382319422, 0.000000000000000000 ) ) ;
#25457=EDGE_CURVE ( 'NONE', #1534, #6404, #3740, .T. ) ;
#25460=LINE ( 'NONE', #5782, #26186 ) ;
#25462=EDGE_CURVE ( 'NONE', #1874, #12868, #20853, .T. ) ;
#25463=ORIENTED_EDGE ( 'NONE', *, *, #27105, .F. ) ;
#25464=CARTESIAN_POINT ( 'NONE',  ( 157.4999999999996305, 283.9508126914284958, 45.00000000000000000 ) ) ;
#25467=FACE_OUTER_BOUND ( 'NONE', #21636, .T. ) ;
#25470=VECTOR ( 'NONE', #26985, 1000.000000000000000 ) ;
#25473=EDGE_CURVE ( 'NONE', #27032, #2768, #20708, .T. ) ;
#25477=ORIENTED_EDGE ( 'NONE', *, *, #2169, .T. ) ;
#25484=DIRECTION ( 'NONE',  ( -0.8916010070299977830, 0.4528218681370124177, 0.000000000000000000 ) ) ;
#25486=ORIENTED_EDGE ( 'NONE', *, *, #19633, .T. ) ;
#25489=VECTOR ( 'NONE', #5215, 1000.000000000000000 ) ;
#25491=VERTEX_POINT ( 'NONE', #7511 ) ;
#25492=VECTOR ( 'NONE', #5682, 1000.000000000000000 ) ;
#25493=AXIS2_PLACEMENT_3D ( 'NONE', #25344, #12290, #25484 ) ;
#25494=ADVANCED_FACE ( 'NONE', ( #16278 ), #25031, .F. ) ;
#25504=DIRECTION ( 'NONE',  ( 0.8916010070317489378, -0.4528218681335642315, 0.000000000000000000 ) ) ;
#25507=LINE ( 'NONE', #5691, #13248 ) ;
#25508=CARTESIAN_POINT ( 'NONE',  ( 157.9999999999998010, 236.0472500450420341, 45.00000000000000000 ) ) ;
#25509=CARTESIAN_POINT ( 'NONE',  ( 157.4999999999998579, 103.3838121509225090, -45.00000000000000000 ) ) ;
#25515=ADVANCED_FACE ( 'NONE', ( #26004 ), #10792, .F. ) ;
#25519=ORIENTED_EDGE ( 'NONE', *, *, #10483, .F. ) ;
#25520=ORIENTED_EDGE ( 'NONE', *, *, #21408, .T. ) ;
#25523=ORIENTED_EDGE ( 'NONE', *, *, #18083, .T. ) ;
#25526=DIRECTION ( 'NONE',  ( -0.000000000000000000, -0.000000000000000000, -1.000000000000000000 ) ) ;
#25541=LINE ( 'NONE', #19222, #15693 ) ;
#25542=ORIENTED_EDGE ( 'NONE', *, *, #7217, .T. ) ;
#25547=ORIENTED_EDGE ( 'NONE', *, *, #20675, .T. ) ;
#25549=ORIENTED_EDGE ( 'NONE', *, *, #25110, .F. ) ;
#25553=EDGE_CURVE ( 'NONE', #17961, #13726, #17529, .T. ) ;
#25556=PLANE ( 'NONE',  #22500 ) ;
#25557=CARTESIAN_POINT ( 'NONE',  ( 158.0000000000005116, 160.8109998198309825, 45.00000000000000000 ) ) ;
#25559=VECTOR ( 'NONE', #25696, 1000.000000000000114 ) ;
#25562=DIRECTION ( 'NONE',  ( -0.8916010070294396739, 0.4528218681381114274, 0.000000000000000000 ) ) ;
#25564=ORIENTED_EDGE ( 'NONE', *, *, #1640, .F. ) ;
#25566=EDGE_CURVE ( 'NONE', #21412, #18321, #26294, .T. ) ;
#25568=ORIENTED_EDGE ( 'NONE', *, *, #15869, .T. ) ;
#25573=PLANE ( 'NONE',  #13389 ) ;
#25575=CARTESIAN_POINT ( 'NONE',  ( 158.0000000000011084, 98.62199963966197913, 45.00000000000000000 ) ) ;
#25576=ORIENTED_EDGE ( 'NONE', *, *, #26398, .F. ) ;
#25577=ORIENTED_EDGE ( 'NONE', *, *, #436, .T. ) ;
#25582=ADVANCED_FACE ( 'NONE', ( #2157 ), #2017, .F. ) ;
#25586=EDGE_CURVE ( 'NONE', #28150, #7922, #24152, .T. ) ;
#25590=DIRECTION ( 'NONE',  ( -0.000000000000000000, -0.000000000000000000, -1.000000000000000000 ) ) ;
#25591=PLANE ( 'NONE',  #19622 ) ;
#25595=ORIENTED_EDGE ( 'NONE', *, *, #7673, .F. ) ;
#25596=DIRECTION ( 'NONE',  ( 1.000000000000000000, -0.000000000000000000, -0.000000000000000000 ) ) ;
#25599=DIRECTION ( 'NONE',  ( -0.000000000000000000, -0.000000000000000000, -1.000000000000000000 ) ) ;
#25602=CARTESIAN_POINT ( 'NONE',  ( 157.9999999999998579, 219.0000000000000284, -45.00000000000000000 ) ) ;
#25603=ORIENTED_EDGE ( 'NONE', *, *, #23557, .F. ) ;
#25606=FACE_OUTER_BOUND ( 'NONE', #590, .T. ) ;
#25608=EDGE_LOOP ( 'NONE', ( #5619, #15294, #22704, #723 ) ) ;
#25609=LINE ( 'NONE', #3214, #22559 ) ;
#25614=PLANE ( 'NONE',  #25493 ) ;
#25616=VERTEX_POINT ( 'NONE', #19262 ) ;
#25618=ADVANCED_FACE ( 'NONE', ( #2293 ), #8350, .F. ) ;
#25619=ORIENTED_EDGE ( 'NONE', *, *, #25437, .T. ) ;
#25620=EDGE_CURVE ( 'NONE', #27414, #16958, #25866, .T. ) ;
#25624=VERTEX_POINT ( 'NONE', #16967 ) ;
#25626=CARTESIAN_POINT ( 'NONE',  ( 158.0000000000007958, 128.7164997297464595, 45.00000000000000000 ) ) ;
#25627=VECTOR ( 'NONE', #24435, 999.9999999999998863 ) ;
#25629=CARTESIAN_POINT ( 'NONE',  ( 157.4999999999998579, 196.1751874286831026, 45.00000000000000000 ) ) ;
#25630=DIRECTION ( 'NONE',  ( 0.8916010070293783896, -0.4528218681382319422, 0.000000000000000000 ) ) ;
#25631=DIRECTION ( 'NONE',  ( 0.000000000000000000, -1.000000000000000000, 0.000000000000000000 ) ) ;
#25632=CARTESIAN_POINT ( 'NONE',  ( 157.4999999999998579, 105.8916871584295478, 45.00000000000000000 ) ) ;
#25636=AXIS2_PLACEMENT_3D ( 'NONE', #2177, #17414, #326 ) ;
#25637=LINE ( 'NONE', #10143, #27587 ) ;
#25638=CARTESIAN_POINT ( 'NONE',  ( 158.0000000000005400, 158.3031248123239436, 45.00000000000000000 ) ) ;
#25639=LINE ( 'NONE', #28209, #4758 ) ;
#25645=( LENGTH_UNIT ( ) NAMED_UNIT ( * ) SI_UNIT ( .MILLI., .METRE. ) );
#25648=AXIS2_PLACEMENT_3D ( 'NONE', #11807, #20547, #872 ) ;
#25649=CARTESIAN_POINT ( 'NONE',  ( 157.9999999999996589, 278.6811251726610976, 45.00000000000000000 ) ) ;
#25652=ORIENTED_EDGE ( 'NONE', *, *, #16592, .T. ) ;
#25653=EDGE_LOOP ( 'NONE', ( #25439, #16099, #15214, #25486 ) ) ;
#25656=EDGE_CURVE ( 'NONE', #17953, #7888, #26867, .T. ) ;
#25659=ORIENTED_EDGE ( 'NONE', *, *, #7453, .F. ) ;
#25661=FACE_OUTER_BOUND ( 'NONE', #6427, .T. ) ;
#25669=LINE ( 'NONE', #5851, #8494 ) ;
#25673=CARTESIAN_POINT ( 'NONE',  ( 158.0000000000011653, 95.60624962464788723, 45.00000000000000000 ) ) ;
#25674=CARTESIAN_POINT ( 'NONE',  ( 157.9999999999996589, 276.6811251726610976, 45.00000000000000000 ) ) ;
#25675=LINE ( 'NONE', #6424, #70 ) ;
#25676=DIRECTION ( 'NONE',  ( -0.000000000000000000, 0.000000000000000000, -1.000000000000000000 ) ) ;
#25677=LINE ( 'NONE', #12766, #25384 ) ;
#25679=VECTOR ( 'NONE', #1367, 1000.000000000000114 ) ;
#25682=DIRECTION ( 'NONE',  ( 0.4528218681380503097, -0.8916010070294707601, 0.000000000000000000 ) ) ;
#25684=ORIENTED_EDGE ( 'NONE', *, *, #26446, .T. ) ;
#25685=EDGE_CURVE ( 'NONE', #4413, #3398, #17816, .T. ) ;
#25692=EDGE_LOOP ( 'NONE', ( #7694, #3804, #7262, #2433 ) ) ;
#25693=EDGE_CURVE ( 'NONE', #6606, #7851, #27804, .T. ) ;
#25694=VERTEX_POINT ( 'NONE', #21489 ) ;
#25696=DIRECTION ( 'NONE',  ( -0.8916010070293383105, -0.4528218681383106015, 0.000000000000000000 ) ) ;
#25697=VECTOR ( 'NONE', #12587, 1000.000000000000000 ) ;
#25700=VECTOR ( 'NONE', #24261, 1000.000000000000000 ) ;
#25701=CARTESIAN_POINT ( 'NONE',  ( 158.0000000000000000, 208.4606249624626457, 45.00000000000000000 ) ) ;
#25702=EDGE_CURVE ( 'NONE', #8924, #4742, #1531, .T. ) ;
#25703=LINE ( 'NONE', #25424, #23155 ) ;
#25704=FACE_OUTER_BOUND ( 'NONE', #13096, .T. ) ;
#25709=CARTESIAN_POINT ( 'NONE',  ( 158.0000000000000853, 200.9369999399436892, 45.00000000000000000 ) ) ;
#25718=EDGE_CURVE ( 'NONE', #3367, #28150, #23509, .T. ) ;
#25720=PLANE ( 'NONE',  #21666 ) ;
#25722=ORIENTED_EDGE ( 'NONE', *, *, #6195, .T. ) ;
#25723=ADVANCED_FACE ( 'NONE', ( #1671 ), #10439, .F. ) ;
#25725=LINE ( 'NONE', #10228, #25104 ) ;
#25733=DIRECTION ( 'NONE',  ( -0.8916010070297446521, -0.4528218681375106858, 0.000000000000000000 ) ) ;
#25734=LINE ( 'NONE', #6203, #12807 ) ;
#25742=CARTESIAN_POINT ( 'NONE',  ( 157.9999999999997158, 263.6338751276190351, 45.00000000000000000 ) ) ;
#25743=ORIENTED_EDGE ( 'NONE', *, *, #18917, .F. ) ;
#25746=PLANE ( 'NONE',  #11035 ) ;
#25751=ORIENTED_EDGE ( 'NONE', *, *, #2369, .T. ) ;
#25752=EDGE_CURVE ( 'NONE', #16142, #19893, #11801, .T. ) ;
#25754=VECTOR ( 'NONE', #14178, 1000.000000000000000 ) ;
#25758=ORIENTED_EDGE ( 'NONE', *, *, #24958, .F. ) ;
#25759=VECTOR ( 'NONE', #18697, 1000.000000000000000 ) ;
#25762=CARTESIAN_POINT ( 'NONE',  ( 158.0000000000013074, 83.06687458711267880, 45.00000000000000000 ) ) ;
#25763=ORIENTED_EDGE ( 'NONE', *, *, #14271, .F. ) ;
#25765=ORIENTED_EDGE ( 'NONE', *, *, #3719, .F. ) ;
#25776=PLANE ( 'NONE',  #12247 ) ;
#25783=EDGE_CURVE ( 'NONE', #170, #17429, #21634, .T. ) ;
#25786=DIRECTION ( 'NONE',  ( 0.8916010070294395629, -0.4528218681381114274, 0.000000000000000000 ) ) ;
#25789=PLANE ( 'NONE',  #13231 ) ;
#25791=ORIENTED_EDGE ( 'NONE', *, *, #5590, .F. ) ;
#25792=ADVANCED_FACE ( 'NONE', ( #12889 ), #4387, .F. ) ;
#25794=ORIENTED_EDGE ( 'NONE', *, *, #3861, .T. ) ;
#25795=EDGE_CURVE ( 'NONE', #18838, #9458, #10867, .T. ) ;
#25797=EDGE_LOOP ( 'NONE', ( #2511, #17765, #19898, #12528 ) ) ;
#25803=ORIENTED_EDGE ( 'NONE', *, *, #10935, .T. ) ;
#25804=CARTESIAN_POINT ( 'NONE',  ( 158.0000000000005969, 148.7794997898028271, 45.00000000000000000 ) ) ;
#25807=VECTOR ( 'NONE', #19965, 1000.000000000000000 ) ;
#25816=LINE ( 'NONE', #19074, #19323 ) ;
#25819=ORIENTED_EDGE ( 'NONE', *, *, #25877, .F. ) ;
#25821=EDGE_CURVE ( 'NONE', #15637, #9868, #8707, .T. ) ;
#25823=DIRECTION ( 'NONE',  ( -0.8916010070298868717, -0.4528218681372309651, 0.000000000000000000 ) ) ;
#25827=ORIENTED_EDGE ( 'NONE', *, *, #6916, .F. ) ;
#25828=ORIENTED_EDGE ( 'NONE', *, *, #8505, .T. ) ;
#25831=ORIENTED_EDGE ( 'NONE', *, *, #14468, .F. ) ;
#25834=EDGE_CURVE ( 'NONE', #19162, #23817, #4248, .T. ) ;
#25835=EDGE_LOOP ( 'NONE', ( #1338, #14475, #2512, #24171 ) ) ;
#25843=EDGE_CURVE ( 'NONE', #21211, #26462, #21918, .T. ) ;
#25846=CARTESIAN_POINT ( 'NONE',  ( 158.0000000000009379, 118.1771246922112653, -45.00000000000000000 ) ) ;
#25850=DIRECTION ( 'NONE',  ( 0.000000000000000000, -1.000000000000000000, 0.000000000000000000 ) ) ;
#25858=ORIENTED_EDGE ( 'NONE', *, *, #9420, .F. ) ;
#25860=VECTOR ( 'NONE', #6247, 1000.000000000000000 ) ;
#25864=EDGE_CURVE ( 'NONE', #5196, #19742, #9134, .T. ) ;
#25866=LINE ( 'NONE', #8205, #26423 ) ;
#25874=EDGE_LOOP ( 'NONE', ( #8322, #3322, #9237, #7080 ) ) ;
#25876=CARTESIAN_POINT ( 'NONE',  ( 157.4999999999998579, 128.4625622259929401, -45.00000000000000000 ) ) ;
#25877=EDGE_CURVE ( 'NONE', #19152, #26356, #15471, .T. ) ;
#25879=VECTOR ( 'NONE', #14109, 1000.000000000000000 ) ;
#25881=EDGE_CURVE ( 'NONE', #372, #12774, #4523, .T. ) ;
#25882=ADVANCED_FACE ( 'NONE', ( #22206 ), #26494, .F. ) ;
#25883=DIRECTION ( 'NONE',  ( 0.4528218681382319422, 0.8916010070293783896, -0.000000000000000000 ) ) ;
#25886=ADVANCED_FACE ( 'NONE', ( #19483 ), #24351, .F. ) ;
#25888=PLANE ( 'NONE',  #17976 ) ;
#25903=ORIENTED_EDGE ( 'NONE', *, *, #16572, .F. ) ;
#25904=CARTESIAN_POINT ( 'NONE',  ( 157.4999999999996589, 273.9193126614005678, 45.00000000000000000 ) ) ;
#25907=EDGE_LOOP ( 'NONE', ( #9948, #14302, #19567, #14193 ) ) ;
#25908=CARTESIAN_POINT ( 'NONE',  ( 158.0000000000000853, 198.9369999399436892, -45.00000000000000000 ) ) ;
#25911=DIRECTION ( 'NONE',  ( -0.000000000000000000, 0.000000000000000000, -1.000000000000000000 ) ) ;
#25914=EDGE_CURVE ( 'NONE', #19932, #17959, #11445, .T. ) ;
#25916=LINE ( 'NONE', #6099, #25697 ) ;
#25917=LINE ( 'NONE', #14881, #25492 ) ;
#25919=ORIENTED_EDGE ( 'NONE', *, *, #13358, .T. ) ;
#25922=LINE ( 'NONE', #17021, #17955 ) ;
#25924=CARTESIAN_POINT ( 'NONE',  ( 158.0000000000006537, 143.2558747672816821, -45.00000000000000000 ) ) ;
#25925=ORIENTED_EDGE ( 'NONE', *, *, #924, .F. ) ;
#25927=DIRECTION ( 'NONE',  ( 0.4528218681379903021, -0.8916010070295011802, 0.000000000000000000 ) ) ;
#25929=DIRECTION ( 'NONE',  ( 0.4528218681381501742, -0.8916010070294199119, 0.000000000000000000 ) ) ;
#25932=ORIENTED_EDGE ( 'NONE', *, *, #6713, .T. ) ;
#25935=ADVANCED_FACE ( 'NONE', ( #13744 ), #9428, .F. ) ;
#25936=CARTESIAN_POINT ( 'NONE',  ( 158.0000000000015916, 55.48024950453520177, -45.00000000000000000 ) ) ;
#25939=VECTOR ( 'NONE', #12865, 1000.000000000000000 ) ;
#25944=EDGE_CURVE ( 'NONE', #695, #12922, #3079, .T. ) ;
#25945=ORIENTED_EDGE ( 'NONE', *, *, #25013, .T. ) ;
#25946=VECTOR ( 'NONE', #10215, 1000.000000000000227 ) ;
#25950=DIRECTION ( 'NONE',  ( -0.000000000000000000, -0.000000000000000000, -1.000000000000000000 ) ) ;
#25953=ADVANCED_FACE ( 'NONE', ( #7122 ), #518, .F. ) ;
#25955=DIRECTION ( 'NONE',  ( -0.8916010070299172918, -0.4528218681371710685, 0.000000000000000000 ) ) ;
#25957=EDGE_CURVE ( 'NONE', #5675, #1568, #14162, .T. ) ;
#25962=PLANE ( 'NONE',  #5892 ) ;
#25964=VECTOR ( 'NONE', #17998, 1000.000000000000000 ) ;
#25965=VERTEX_POINT ( 'NONE', #18041 ) ;
#25966=DIRECTION ( 'NONE',  ( -0.8916010070293383105, -0.4528218681383106015, 0.000000000000000000 ) ) ;
#25967=PLANE ( 'NONE',  #21774 ) ;
#25968=DIRECTION ( 'NONE',  ( -0.8916010070293383105, -0.4528218681383106015, 0.000000000000000000 ) ) ;
#25977=ORIENTED_EDGE ( 'NONE', *, *, #14866, .F. ) ;
#25978=ORIENTED_EDGE ( 'NONE', *, *, #19903, .T. ) ;
#25979=VECTOR ( 'NONE', #25302, 1000.000000000000114 ) ;
#25982=DIRECTION ( 'NONE',  ( -0.8916010070298968637, -0.4528218681372109811, 0.000000000000000000 ) ) ;
#25983=VECTOR ( 'NONE', #18344, 1000.000000000000000 ) ;
#25986=EDGE_CURVE ( 'NONE', #1215, #14420, #11871, .T. ) ;
#25988=CARTESIAN_POINT ( 'NONE',  ( 157.4999999999998579, 221.2539375037535194, 45.00000000000000000 ) ) ;
#25990=EDGE_CURVE ( 'NONE', #27621, #25194, #26800, .T. ) ;
#25993=DIRECTION ( 'NONE',  ( 0.8916010070317489378, -0.4528218681335642315, 0.000000000000000000 ) ) ;
#26000=ORIENTED_EDGE ( 'NONE', *, *, #24863, .F. ) ;
#26004=FACE_OUTER_BOUND ( 'NONE', #2110, .T. ) ;
#26005=VERTEX_POINT ( 'NONE', #4951 ) ;
#26014=VECTOR ( 'NONE', #17853, 1000.000000000000000 ) ;
#26022=ADVANCED_FACE ( 'NONE', ( #1076 ), #9844, .F. ) ;
#26024=DIRECTION ( 'NONE',  ( 1.000000000000000000, 0.000000000000000000, -0.000000000000000000 ) ) ;
#26025=LINE ( 'NONE', #24029, #571 ) ;
#26026=DIRECTION ( 'NONE',  ( -0.8916010070299376089, -0.4528218681371311005, 0.000000000000000000 ) ) ;
#26027=EDGE_LOOP ( 'NONE', ( #26598, #16936, #2540, #20843 ) ) ;
#26028=CARTESIAN_POINT ( 'NONE',  ( 157.4999999999998579, 186.1436873986549188, 45.00000000000000000 ) ) ;
#26030=DIRECTION ( 'NONE',  ( 0.4528218681370523302, 0.8916010070299774659, -0.000000000000000000 ) ) ;
#26031=CARTESIAN_POINT ( 'NONE',  ( 157.9999999999996874, 268.6496251426330559, 45.00000000000000000 ) ) ;
#26035=LINE ( 'NONE', #6356, #6082 ) ;
#26036=ORIENTED_EDGE ( 'NONE', *, *, #21618, .T. ) ;
#26040=FACE_OUTER_BOUND ( 'NONE', #17637, .T. ) ;
#26042=ORIENTED_EDGE ( 'NONE', *, *, #1911, .F. ) ;
#26043=VERTEX_POINT ( 'NONE', #25762 ) ;
#26045=ORIENTED_EDGE ( 'NONE', *, *, #1779, .T. ) ;
#26046=CARTESIAN_POINT ( 'NONE',  ( 158.0000000000017337, 40.94087446699997912, 45.00000000000000000 ) ) ;
#26049=VERTEX_POINT ( 'NONE', #14721 ) ;
#26055=CARTESIAN_POINT ( 'NONE',  ( 158.0000000000008811, 121.1928747072253572, 45.00000000000000000 ) ) ;
#26061=CARTESIAN_POINT ( 'NONE',  ( 158.0000000000006253, 148.2716247822957882, -45.00000000000000000 ) ) ;
#26064=ORIENTED_EDGE ( 'NONE', *, *, #4505, .F. ) ;
#26067=DIRECTION ( 'NONE',  ( 0.8916010070295011802, 0.4528218681379903021, 0.000000000000000000 ) ) ;
#26072=VERTEX_POINT ( 'NONE', #7690 ) ;
#26076=VECTOR ( 'NONE', #14005, 1000.000000000000114 ) ;
#26077=EDGE_LOOP ( 'NONE', ( #2053, #1489, #23419, #4348 ) ) ;
#26078=ORIENTED_EDGE ( 'NONE', *, *, #21438, .F. ) ;
#26079=EDGE_CURVE ( 'NONE', #16458, #10433, #1217, .T. ) ;
#26081=ORIENTED_EDGE ( 'NONE', *, *, #26497, .F. ) ;
#26085=CARTESIAN_POINT ( 'NONE',  ( 158.0000000000008527, 125.7007497147323818, 45.00000000000000000 ) ) ;
#26086=LINE ( 'NONE', #23946, #21806 ) ;
#26087=PLANE ( 'NONE',  #892 ) ;
#26089=VECTOR ( 'NONE', #26624, 1000.000000000000114 ) ;
#26091=CARTESIAN_POINT ( 'NONE',  ( 158.0000000000005969, 150.7794997898028271, 45.00000000000000000 ) ) ;
#26094=DIRECTION ( 'NONE',  ( 0.4528218681370324572, 0.8916010070299876800, -0.000000000000000000 ) ) ;
#26098=ORIENTED_EDGE ( 'NONE', *, *, #22661, .F. ) ;
#26099=FACE_OUTER_BOUND ( 'NONE', #8992, .T. ) ;
#26100=VECTOR ( 'NONE', #4887, 1000.000000000000114 ) ;
#26113=ADVANCED_FACE ( 'NONE', ( #10267 ), #10404, .F. ) ;
#26121=VECTOR ( 'NONE', #16668, 999.9999999999998863 ) ;
#26125=LINE ( 'NONE', #2271, #18398 ) ;
#26126=PLANE ( 'NONE',  #8988 ) ;
#26131=DIRECTION ( 'NONE',  ( -0.000000000000000000, -0.000000000000000000, -1.000000000000000000 ) ) ;
#26133=AXIS2_PLACEMENT_3D ( 'NONE', #26519, #19781, #106 ) ;
#26137=FACE_OUTER_BOUND ( 'NONE', #27687, .T. ) ;
#26138=ORIENTED_EDGE ( 'NONE', *, *, #514, .T. ) ;
#26145=PRODUCT_CONTEXT ( 'NONE', #18281, 'mechanical' ) ;
#26146=ORIENTED_EDGE ( 'NONE', *, *, #9614, .F. ) ;
#26149=VECTOR ( 'NONE', #13608, 1000.000000000000000 ) ;
#26150=DIRECTION ( 'NONE',  ( 0.4528218681383305855, -0.8916010070293283185, 0.000000000000000000 ) ) ;
#26151=EDGE_CURVE ( 'NONE', #16250, #8798, #20895, .T. ) ;
#26165=ORIENTED_EDGE ( 'NONE', *, *, #15183, .F. ) ;
#26166=VECTOR ( 'NONE', #14589, 1000.000000000000000 ) ;
#26168=CARTESIAN_POINT ( 'NONE',  ( 157.4999999999998579, 146.0176872785422404, 45.00000000000000000 ) ) ;
#26169=DIRECTION ( 'NONE',  ( -0.8916010070299679180, -0.4528218681370710375, 0.000000000000000000 ) ) ;
#26171=ORIENTED_EDGE ( 'NONE', *, *, #16147, .F. ) ;
#26178=VERTEX_POINT ( 'NONE', #21316 ) ;
#26179=ORIENTED_EDGE ( 'NONE', *, *, #19794, .T. ) ;
#26182=ORIENTED_EDGE ( 'NONE', *, *, #10352, .T. ) ;
#26186=VECTOR ( 'NONE', #14557, 1000.000000000000000 ) ;
#26187=EDGE_CURVE ( 'NONE', #20000, #21343, #1633, .T. ) ;
#26192=CARTESIAN_POINT ( 'NONE',  ( 158.0000000000016200, 50.97237449702815582, 45.00000000000000000 ) ) ;
#26195=EDGE_CURVE ( 'NONE', #12815, #5308, #19300, .T. ) ;
#26197=DIRECTION ( 'NONE',  ( 0.8916010070297643031, -0.4528218681374719945, 0.000000000000000000 ) ) ;
#26201=FACE_OUTER_BOUND ( 'NONE', #22080, .T. ) ;
#26202=CARTESIAN_POINT ( 'NONE',  ( 158.0000000000009095, 120.6849996997183183, 45.00000000000000000 ) ) ;
#26209=CARTESIAN_POINT ( 'NONE',  ( 157.9999999999998295, 231.0315000300280417, 45.00000000000000000 ) ) ;
#26210=FACE_OUTER_BOUND ( 'NONE', #26941, .T. ) ;
#26211=LINE ( 'NONE', #22049, #1438 ) ;
#26214=VECTOR ( 'NONE', #6152, 1000.000000000000000 ) ;
#26221=CARTESIAN_POINT ( 'NONE',  ( 157.4999999999998579, 188.6515624061619576, 45.00000000000000000 ) ) ;
#26223=EDGE_LOOP ( 'NONE', ( #25419, #23495, #20960, #21096 ) ) ;
#26224=ORIENTED_EDGE ( 'NONE', *, *, #2678, .F. ) ;
#26228=AXIS2_PLACEMENT_3D ( 'NONE', #24063, #15310, #2487 ) ;
#26229=CARTESIAN_POINT ( 'NONE',  ( 158.0000000000001137, 193.9212499249295831, -45.00000000000000000 ) ) ;
#26238=CARTESIAN_POINT ( 'NONE',  ( 217.4999999999996305, 258.6181251126050711, 1.387778780781445676E-14 ) ) ;
#26239=LINE ( 'NONE', #6566, #12654 ) ;
#26240=CARTESIAN_POINT ( 'NONE',  ( 157.9999999999996874, 269.1575001501400379, 45.00000000000000000 ) ) ;
#26243=EDGE_CURVE ( 'NONE', #226, #19699, #4063, .T. ) ;
#26244=ORIENTED_EDGE ( 'NONE', *, *, #12385, .F. ) ;
#26250=DIRECTION ( 'NONE',  ( 0.4528218681371523058, 0.8916010070299268397, -0.000000000000000000 ) ) ;
#26257=EDGE_LOOP ( 'NONE', ( #21019, #21240, #25385, #4518 ) ) ;
#26259=VERTEX_POINT ( 'NONE', #17285 ) ;
#26263=ORIENTED_EDGE ( 'NONE', *, *, #3358, .F. ) ;
#26270=DIRECTION ( 'NONE',  ( 0.8916010070293783896, 0.4528218681382319422, 0.000000000000000000 ) ) ;
#26271=VECTOR ( 'NONE', #4441, 1000.000000000000000 ) ;
#26273=DIRECTION ( 'NONE',  ( -0.000000000000000000, -0.000000000000000000, -1.000000000000000000 ) ) ;
#26276=CARTESIAN_POINT ( 'NONE',  ( 158.0000000000011369, 98.11412463215494029, 45.00000000000000000 ) ) ;
#26277=CARTESIAN_POINT ( 'NONE',  ( 158.0000000000001705, 190.9054999099155054, 45.00000000000000000 ) ) ;
#26292=EDGE_LOOP ( 'NONE', ( #6755, #10670, #27943, #5031 ) ) ;
#26293=DIRECTION ( 'NONE',  ( 0.8916010070293783896, -0.4528218681382319422, 0.000000000000000000 ) ) ;
#26294=LINE ( 'NONE', #13239, #21848 ) ;
#26296=VECTOR ( 'NONE', #1688, 1000.000000000000000 ) ;
#26298=CARTESIAN_POINT ( 'NONE',  ( 157.9999999999996874, 266.6496251426330559, -45.00000000000000000 ) ) ;
#26301=CARTESIAN_POINT ( 'NONE',  ( 157.9999999999998010, 241.0630000600560550, -45.00000000000000000 ) ) ;
#26302=CARTESIAN_POINT ( 'NONE',  ( 158.0000000000016200, 52.97237449702815582, 45.00000000000000000 ) ) ;
#26306=VERTEX_POINT ( 'NONE', #21746 ) ;
#26309=EDGE_CURVE ( 'NONE', #548, #7521, #19446, .T. ) ;
#26310=DIRECTION ( 'NONE',  ( -0.000000000000000000, 0.000000000000000000, -1.000000000000000000 ) ) ;
#26311=DIRECTION ( 'NONE',  ( 0.000000000000000000, -1.000000000000000000, 0.000000000000000000 ) ) ;
#26313=DIRECTION ( 'NONE',  ( -0.8916010070293995948, -0.4528218681381900867, 0.000000000000000000 ) ) ;
#26314=ORIENTED_EDGE ( 'NONE', *, *, #15351, .F. ) ;
#26318=EDGE_LOOP ( 'NONE', ( #15562, #17001, #16738, #24849 ) ) ;
#26327=ORIENTED_EDGE ( 'NONE', *, *, #1975, .F. ) ;
#26328=ADVANCED_FACE ( 'NONE', ( #2054 ), #13413, .F. ) ;
#26336=PLANE ( 'NONE',  #4044 ) ;
#26337=LINE ( 'NONE', #15305, #12882 ) ;
#26339=ORIENTED_EDGE ( 'NONE', *, *, #15960, .T. ) ;
#26340=PLANE ( 'NONE',  #6261 ) ;
#26343=CARTESIAN_POINT ( 'NONE',  ( 157.9999999999998579, 219.0000000000000284, 45.00000000000000000 ) ) ;
#26344=ORIENTED_EDGE ( 'NONE', *, *, #3413, .T. ) ;
#26345=CARTESIAN_POINT ( 'NONE',  ( 157.9999999999997158, 263.6338751276190351, 45.00000000000000000 ) ) ;
#26346=ORIENTED_EDGE ( 'NONE', *, *, #19088, .F. ) ;
#26347=EDGE_CURVE ( 'NONE', #28117, #8556, #5347, .T. ) ;
#26353=VECTOR ( 'NONE', #959, 1000.000000000000000 ) ;
#26354=ORIENTED_EDGE ( 'NONE', *, *, #23476, .T. ) ;
#26356=VERTEX_POINT ( 'NONE', #898 ) ;
#26362=ORIENTED_EDGE ( 'NONE', *, *, #23533, .T. ) ;
#26363=ORIENTED_EDGE ( 'NONE', *, *, #19261, .T. ) ;
#26369=FACE_OUTER_BOUND ( 'NONE', #8430, .T. ) ;
#26370=VECTOR ( 'NONE', #23605, 1000.000000000000114 ) ;
#26371=CARTESIAN_POINT ( 'NONE',  ( 157.4999999999998579, 173.6043123611196961, -45.00000000000000000 ) ) ;
#26372=LINE ( 'NONE', #6420, #23627 ) ;
#26376=DIRECTION ( 'NONE',  ( 0.000000000000000000, -1.000000000000000000, 0.000000000000000000 ) ) ;
#26377=DIRECTION ( 'NONE',  ( -0.000000000000000000, -0.000000000000000000, -1.000000000000000000 ) ) ;
#26381=LINE ( 'NONE', #6709, #19451 ) ;
#26386=DIRECTION ( 'NONE',  ( -0.8916010070294402290, -0.4528218681381102062, 0.000000000000000000 ) ) ;
#26387=VERTEX_POINT ( 'NONE', #15863 ) ;
#26392=ADVANCED_FACE ( 'NONE', ( #7371 ), #16001, .F. ) ;
#26394=ORIENTED_EDGE ( 'NONE', *, *, #6300, .T. ) ;
#26396=ORIENTED_EDGE ( 'NONE', *, *, #546, .T. ) ;
#26398=EDGE_CURVE ( 'NONE', #24882, #26528, #11695, .T. ) ;
#26403=VECTOR ( 'NONE', #11256, 1000.000000000000000 ) ;
#26404=FACE_OUTER_BOUND ( 'NONE', #16388, .T. ) ;
#26406=LINE ( 'NONE', #28131, #25700 ) ;
#26407=DIRECTION ( 'NONE',  ( 0.4528218681371722343, 0.8916010070299166257, -0.000000000000000000 ) ) ;
#26409=CARTESIAN_POINT ( 'NONE',  ( 157.9999999999998295, 226.5236250225210313, -45.00000000000000000 ) ) ;
#26411=FACE_OUTER_BOUND ( 'NONE', #15417, .T. ) ;
#26412=LINE ( 'NONE', #10628, #7004 ) ;
#26413=CARTESIAN_POINT ( 'NONE',  ( 157.4999999999998579, 118.4310621959647563, 45.00000000000000000 ) ) ;
#26416=DIRECTION ( 'NONE',  ( 0.000000000000000000, -1.000000000000000000, 0.000000000000000000 ) ) ;
#26418=EDGE_LOOP ( 'NONE', ( #9280, #11483, #12773, #10078 ) ) ;
#26421=VERTEX_POINT ( 'NONE', #22311 ) ;
#26423=VECTOR ( 'NONE', #19120, 1000.000000000000114 ) ;
#26436=PLANE ( 'NONE',  #7566 ) ;
#26438=AXIS2_PLACEMENT_3D ( 'NONE', #15903, #5383, #9279 ) ;
#26440=DIRECTION ( 'NONE',  ( 0.4528218681374120425, 0.8916010070297948342, -0.000000000000000000 ) ) ;
#26442=CARTESIAN_POINT ( 'NONE',  ( 158.0000000000011084, 100.6219996396619791, 45.00000000000000000 ) ) ;
#26446=EDGE_CURVE ( 'NONE', #24140, #3327, #22874, .T. ) ;
#26450=ORIENTED_EDGE ( 'NONE', *, *, #4531, .F. ) ;
#26451=DIRECTION ( 'NONE',  ( -0.000000000000000000, -0.000000000000000000, -1.000000000000000000 ) ) ;
#26458=CARTESIAN_POINT ( 'NONE',  ( 157.4999999999998579, 146.0176872785422404, -45.00000000000000000 ) ) ;
#26462=VERTEX_POINT ( 'NONE', #16832 ) ;
#26463=EDGE_LOOP ( 'NONE', ( #14181, #18632, #27576, #25444 ) ) ;
#26464=CARTESIAN_POINT ( 'NONE',  ( 157.4999999999998579, 108.3995621659365867, -45.00000000000000000 ) ) ;
#26465=DIRECTION ( 'NONE',  ( -0.000000000000000000, -0.000000000000000000, -1.000000000000000000 ) ) ;
#26466=DIRECTION ( 'NONE',  ( -0.8916010070298563406, -0.4528218681372909171, 0.000000000000000000 ) ) ;
#26470=LINE ( 'NONE', #24059, #24742 ) ;
#26473=DIRECTION ( 'NONE',  ( -0.000000000000000000, -0.000000000000000000, -1.000000000000000000 ) ) ;
#26477=EDGE_LOOP ( 'NONE', ( #27633, #13736, #17526, #1979 ) ) ;
#26484=FACE_OUTER_BOUND ( 'NONE', #8288, .T. ) ;
#26486=ORIENTED_EDGE ( 'NONE', *, *, #15315, .T. ) ;
#26487=EDGE_CURVE ( 'NONE', #2726, #1215, #20992, .T. ) ;
#26488=ADVANCED_FACE ( 'NONE', ( #27730 ), #25447, .F. ) ;
#26490=ORIENTED_EDGE ( 'NONE', *, *, #15463, .F. ) ;
#26492=VERTEX_POINT ( 'NONE', #8069 ) ;
#26493=EDGE_LOOP ( 'NONE', ( #7158, #27201, #23112, #5092 ) ) ;
#26494=PLANE ( 'NONE',  #4406 ) ;
#26497=EDGE_CURVE ( 'NONE', #4389, #11934, #18840, .T. ) ;
#26498=CIRCLE ( 'NONE', #20562, 6.000000000000005329 ) ;
#26499=ORIENTED_EDGE ( 'NONE', *, *, #13609, .F. ) ;
#26505=LINE ( 'NONE', #2376, #11010 ) ;
#26506=DIRECTION ( 'NONE',  ( -0.000000000000000000, -0.000000000000000000, -1.000000000000000000 ) ) ;
#26508=CARTESIAN_POINT ( 'NONE',  ( 157.9999999999997726, 246.0787500750700474, 45.00000000000000000 ) ) ;
#26512=DIRECTION ( 'NONE',  ( -0.8916010070297244461, -0.4528218681375507093, 0.000000000000000000 ) ) ;
#26517=VECTOR ( 'NONE', #21653, 1000.000000000000000 ) ;
#26519=CARTESIAN_POINT ( 'NONE',  ( 157.9999999999997442, 249.0945000900840398, 45.00000000000000000 ) ) ;
#26520=FACE_OUTER_BOUND ( 'NONE', #3790, .T. ) ;
#26522=ORIENTED_EDGE ( 'NONE', *, *, #23941, .T. ) ;
#26523=EDGE_CURVE ( 'NONE', #25624, #1908, #9807, .T. ) ;
#26524=ADVANCED_FACE ( 'NONE', ( #23012 ), #18984, .F. ) ;
#26526=ORIENTED_EDGE ( 'NONE', *, *, #9732, .F. ) ;
#26528=VERTEX_POINT ( 'NONE', #1597 ) ;
#26531=ORIENTED_EDGE ( 'NONE', *, *, #11493, .T. ) ;
#26533=ORIENTED_EDGE ( 'NONE', *, *, #12174, .F. ) ;
#26538=EDGE_CURVE ( 'NONE', #1356, #12421, #5904, .T. ) ;
#26541=FACE_OUTER_BOUND ( 'NONE', #22731, .T. ) ;
#26543=AXIS2_PLACEMENT_3D ( 'NONE', #28159, #12400, #8499 ) ;
#26546=DIRECTION ( 'NONE',  ( 0.4528218681383106015, -0.8916010070293384215, 0.000000000000000000 ) ) ;
#26547=DIRECTION ( 'NONE',  ( 1.000000000000000000, 0.000000000000000000, -0.000000000000000000 ) ) ;
#26549=LINE ( 'NONE', #2995, #11390 ) ;
#26551=EDGE_CURVE ( 'NONE', #18428, #23530, #12114, .T. ) ;
#26552=ADVANCED_FACE ( 'NONE', ( #3323 ), #10368, .F. ) ;
#26559=ORIENTED_EDGE ( 'NONE', *, *, #18672, .T. ) ;
#26562=VECTOR ( 'NONE', #18240, 1000.000000000000114 ) ;
#26563=DIRECTION ( 'NONE',  ( -0.000000000000000000, 0.000000000000000000, -1.000000000000000000 ) ) ;
#26565=ORIENTED_EDGE ( 'NONE', *, *, #13132, .F. ) ;
#26566=VERTEX_POINT ( 'NONE', #5629 ) ;
#26570=PLANE ( 'NONE',  #25340 ) ;
#26573=EDGE_LOOP ( 'NONE', ( #8745, #23059, #26919, #11467 ) ) ;
#26575=EDGE_CURVE ( 'NONE', #22496, #13270, #25725, .T. ) ;
#26578=VERTEX_POINT ( 'NONE', #7653 ) ;
#26579=CARTESIAN_POINT ( 'NONE',  ( 158.0000000000005969, 148.7794997898028271, 45.00000000000000000 ) ) ;
#26580=CARTESIAN_POINT ( 'NONE',  ( 157.9999999999997158, 261.6338751276190351, 45.00000000000000000 ) ) ;
#26581=AXIS2_PLACEMENT_3D ( 'NONE', #3099, #13624, #15922 ) ;
#26585=VECTOR ( 'NONE', #92, 1000.000000000000114 ) ;
#26586=VERTEX_POINT ( 'NONE', #16554 ) ;
#26587=CARTESIAN_POINT ( 'NONE',  ( 158.0000000000016769, 45.95662448201407102, -45.00000000000000000 ) ) ;
#26592=EDGE_CURVE ( 'NONE', #23775, #23149, #23581, .T. ) ;
#26596=DIRECTION ( 'NONE',  ( -0.8916010070295112833, -0.4528218681379702626, 0.000000000000000000 ) ) ;
#26598=ORIENTED_EDGE ( 'NONE', *, *, #25234, .T. ) ;
#26600=ORIENTED_EDGE ( 'NONE', *, *, #18562, .T. ) ;
#26603=DIRECTION ( 'NONE',  ( 1.000000000000000000, 0.000000000000000000, -0.000000000000000000 ) ) ;
#26604=VECTOR ( 'NONE', #27009, 1000.000000000000000 ) ;
#26608=FACE_OUTER_BOUND ( 'NONE', #15905, .T. ) ;
#26610=ORIENTED_EDGE ( 'NONE', *, *, #9225, .F. ) ;
#26614=CARTESIAN_POINT ( 'NONE',  ( 157.4999999999995453, 206.2066874587088989, 45.00000000000000000 ) ) ;
#26620=ORIENTED_EDGE ( 'NONE', *, *, #8156, .F. ) ;
#26621=DIRECTION ( 'NONE',  ( 0.8916010070296226386, 0.4528218681377511601, 0.000000000000000000 ) ) ;
#26622=EDGE_CURVE ( 'NONE', #61, #1444, #15539, .T. ) ;
#26623=LINE ( 'NONE', #8689, #14313 ) ;
#26624=DIRECTION ( 'NONE',  ( -0.8916010070297244461, -0.4528218681375507093, 0.000000000000000000 ) ) ;
#26626=VERTEX_POINT ( 'NONE', #734 ) ;
#26627=LINE ( 'NONE', #19608, #27034 ) ;
#26628=EDGE_CURVE ( 'NONE', #15242, #1653, #24432, .T. ) ;
#26629=ORIENTED_EDGE ( 'NONE', *, *, #2197, .T. ) ;
#26635=CARTESIAN_POINT ( 'NONE',  ( 158.0000000000016769, 45.95662448201407102, 45.00000000000000000 ) ) ;
#26639=EDGE_LOOP ( 'NONE', ( #17995, #5208, #5706, #20369 ) ) ;
#26646=ORIENTED_EDGE ( 'NONE', *, *, #27303, .T. ) ;
#26649=CARTESIAN_POINT ( 'NONE',  ( 157.4999999999998579, 45.70268697826052318, 45.00000000000000000 ) ) ;
#26650=PLANE ( 'NONE',  #6429 ) ;
#26651=ADVANCED_FACE ( 'NONE', ( #11523 ), #19977, .F. ) ;
#26653=EDGE_CURVE ( 'NONE', #9022, #13594, #450, .T. ) ;
#26655=DIRECTION ( 'NONE',  ( 0.4528218681383106015, -0.8916010070293384215, 0.000000000000000000 ) ) ;
#26656=AXIS2_PLACEMENT_3D ( 'NONE', #7137, #11164, #26659 ) ;
#26657=LINE ( 'NONE', #17475, #14078 ) ;
#26659=DIRECTION ( 'NONE',  ( -0.000000000000000000, 0.000000000000000000, -1.000000000000000000 ) ) ;
#26660=CARTESIAN_POINT ( 'NONE',  ( 157.4999999999995453, 206.2066874587088989, 45.00000000000000000 ) ) ;
#26663=PLANE ( 'NONE',  #27540 ) ;
#26664=EDGE_CURVE ( 'NONE', #170, #24882, #17969, .T. ) ;
#26666=ADVANCED_FACE ( 'NONE', ( #20261 ), #9063, .F. ) ;
#26667=DIRECTION ( 'NONE',  ( 1.000000000000000000, 0.000000000000000000, -0.000000000000000000 ) ) ;
#26668=CARTESIAN_POINT ( 'NONE',  ( 158.0000000000015916, 55.48024950453520177, 45.00000000000000000 ) ) ;
#26671=LINE ( 'NONE', #17636, #13924 ) ;
#26672=ORIENTED_EDGE ( 'NONE', *, *, #8102, .T. ) ;
#26676=VECTOR ( 'NONE', #4367, 1000.000000000000000 ) ;
#26683=FACE_OUTER_BOUND ( 'NONE', #12782, .T. ) ;
#26684=CARTESIAN_POINT ( 'NONE',  ( 158.0000000000000853, 198.4291249324366504, 45.00000000000000000 ) ) ;
#26685=VECTOR ( 'NONE', #14602, 1000.000000000000000 ) ;
#26686=CARTESIAN_POINT ( 'NONE',  ( 158.0000000000012506, 88.08262460212675649, 45.00000000000000000 ) ) ;
#26690=LINE ( 'NONE', #17940, #17361 ) ;
#26692=DIRECTION ( 'NONE',  ( -0.8916010070294098089, -0.4528218681381701027, 0.000000000000000000 ) ) ;
#26693=CARTESIAN_POINT ( 'NONE',  ( 157.4999999999998579, 143.5098122710352015, -45.00000000000000000 ) ) ;
#26694=CARTESIAN_POINT ( 'NONE',  ( 157.4999999999996305, 288.9665627064425735, 45.00000000000000000 ) ) ;
#26695=FACE_OUTER_BOUND ( 'NONE', #16579, .T. ) ;
#26698=VECTOR ( 'NONE', #24448, 1000.000000000000000 ) ;
#26699=CARTESIAN_POINT ( 'NONE',  ( 157.4999999999998579, 85.82868709837320864, -45.00000000000000000 ) ) ;
#26700=EDGE_CURVE ( 'NONE', #19053, #969, #2588, .T. ) ;
#26704=VECTOR ( 'NONE', #15966, 1000.000000000000000 ) ;
#26705=EDGE_LOOP ( 'NONE', ( #11848, #20214, #2658, #22456 ) ) ;
#26706=VERTEX_POINT ( 'NONE', #9641 ) ;
#26709=VECTOR ( 'NONE', #8526, 1000.000000000000000 ) ;
#26711=DIRECTION ( 'NONE',  ( 0.4528218681378317068, 0.8916010070295816714, -0.000000000000000000 ) ) ;
#26715=ORIENTED_EDGE ( 'NONE', *, *, #15595, .T. ) ;
#26716=CARTESIAN_POINT ( 'NONE',  ( 158.0000000000001421, 191.4133749174225443, 45.00000000000000000 ) ) ;
#26726=VERTEX_POINT ( 'NONE', #22420 ) ;
#26730=LINE ( 'NONE', #26301, #26766 ) ;
#26733=DIRECTION ( 'NONE',  ( 0.000000000000000000, -1.000000000000000000, 0.000000000000000000 ) ) ;
#26737=PLANE ( 'NONE',  #3604 ) ;
#26739=DIRECTION ( 'NONE',  ( -0.8916010070296732648, 0.4528218681376511845, 0.000000000000000000 ) ) ;
#26740=DIRECTION ( 'NONE',  ( -0.8916010070298360235, -0.4528218681373308852, 0.000000000000000000 ) ) ;
#26743=CARTESIAN_POINT ( 'NONE',  ( 157.4999999999998579, 128.4625622259929401, 45.00000000000000000 ) ) ;
#26744=ADVANCED_FACE ( 'NONE', ( #13818 ), #22569, .F. ) ;
#26746=VECTOR ( 'NONE', #1203, 1000.000000000000000 ) ;
#26751=AXIS2_PLACEMENT_3D ( 'NONE', #21049, #9584, #20771 ) ;
#26753=VECTOR ( 'NONE', #19897, 1000.000000000000000 ) ;
#26754=DIRECTION ( 'NONE',  ( -0.8916010070299882351, -0.4528218681370311249, 0.000000000000000000 ) ) ;
#26756=ORIENTED_EDGE ( 'NONE', *, *, #25457, .F. ) ;
#26757=VECTOR ( 'NONE', #11709, 1000.000000000000000 ) ;
#26758=ORIENTED_EDGE ( 'NONE', *, *, #20723, .F. ) ;
#26761=DIRECTION ( 'NONE',  ( -0.000000000000000000, -0.000000000000000000, -1.000000000000000000 ) ) ;
#26762=ORIENTED_EDGE ( 'NONE', *, *, #25553, .T. ) ;
#26764=VERTEX_POINT ( 'NONE', #3150 ) ;
#26766=VECTOR ( 'NONE', #17826, 1000.000000000000000 ) ;
#26768=EDGE_CURVE ( 'NONE', #19061, #11111, #5452, .T. ) ;
#26772=CARTESIAN_POINT ( 'NONE',  ( 157.9999999999998863, 218.4921249924925348, 45.00000000000000000 ) ) ;
#26774=VECTOR ( 'NONE', #10284, 1000.000000000000114 ) ;
#26775=CARTESIAN_POINT ( 'NONE',  ( 158.0000000000004263, 166.3346248423521274, -45.00000000000000000 ) ) ;
#26778=VERTEX_POINT ( 'NONE', #14374 ) ;
#26781=CARTESIAN_POINT ( 'NONE',  ( 158.0000000000009948, 108.6534996696901345, 45.00000000000000000 ) ) ;
#26783=ORIENTED_EDGE ( 'NONE', *, *, #19889, .F. ) ;
#26786=LINE ( 'NONE', #17733, #3317 ) ;
#26787=CARTESIAN_POINT ( 'NONE',  ( 158.0000000000013358, 78.55899957960562574, -45.00000000000000000 ) ) ;
#26789=VERTEX_POINT ( 'NONE', #20828 ) ;
#26794=LINE ( 'NONE', #19752, #20316 ) ;
#26797=ORIENTED_EDGE ( 'NONE', *, *, #17238, .T. ) ;
#26798=VECTOR ( 'NONE', #8517, 1000.000000000000000 ) ;
#26800=LINE ( 'NONE', #935, #14528 ) ;
#26810=AXIS2_PLACEMENT_3D ( 'NONE', #23306, #21570, #1883 ) ;
#26812=LINE ( 'NONE', #2958, #17223 ) ;
#26815=CARTESIAN_POINT ( 'NONE',  ( 158.0000000000011369, 96.11412463215494029, -45.00000000000000000 ) ) ;
#26817=DIRECTION ( 'NONE',  ( -0.000000000000000000, -0.000000000000000000, -1.000000000000000000 ) ) ;
#26819=CARTESIAN_POINT ( 'NONE',  ( 158.0000000000016769, 45.95662448201407102, 45.00000000000000000 ) ) ;
#26820=ORIENTED_EDGE ( 'NONE', *, *, #26243, .T. ) ;
#26822=ADVANCED_FACE ( 'NONE', ( #27416 ), #10056, .F. ) ;
#26824=LINE ( 'NONE', #9159, #9395 ) ;
#26826=EDGE_LOOP ( 'NONE', ( #7252, #293, #18665, #17896 ) ) ;
#26827=CARTESIAN_POINT ( 'NONE',  ( 158.0000000000014211, 68.52749954957745615, -45.00000000000000000 ) ) ;
#26828=ORIENTED_EDGE ( 'NONE', *, *, #17431, .T. ) ;
#26832=ORIENTED_EDGE ( 'NONE', *, *, #25355, .T. ) ;
#26837=LINE ( 'NONE', #7305, #12304 ) ;
#26840=EDGE_CURVE ( 'NONE', #9674, #4623, #5734, .T. ) ;
#26844=CARTESIAN_POINT ( 'NONE',  ( 157.4999999999998579, 163.5728123310915407, 45.00000000000000000 ) ) ;
#26845=DIRECTION ( 'NONE',  ( -0.000000000000000000, -0.000000000000000000, -1.000000000000000000 ) ) ;
#26847=VECTOR ( 'NONE', #19491, 1000.000000000000000 ) ;
#26849=CARTESIAN_POINT ( 'NONE',  ( 158.0000000000013074, 81.06687458711267880, -45.00000000000000000 ) ) ;
#26850=PLANE ( 'NONE',  #18716 ) ;
#26852=VECTOR ( 'NONE', #20204, 1000.000000000000000 ) ;
#26854=CARTESIAN_POINT ( 'NONE',  ( 167.4999999999996589, 258.6181251126050711, 6.000000000000019540 ) ) ;
#26856=DIRECTION ( 'NONE',  ( 0.8916010070290389944, -0.4528218681389001854, 0.000000000000000000 ) ) ;
#26862=ORIENTED_EDGE ( 'NONE', *, *, #5827, .F. ) ;
#26864=ORIENTED_EDGE ( 'NONE', *, *, #20118, .F. ) ;
#26866=LINE ( 'NONE', #20399, #26704 ) ;
#26867=LINE ( 'NONE', #588, #18187 ) ;
#26868=VERTEX_POINT ( 'NONE', #27701 ) ;
#26870=ORIENTED_EDGE ( 'NONE', *, *, #15072, .F. ) ;
#26873=VECTOR ( 'NONE', #24644, 1000.000000000000000 ) ;
#26880=CARTESIAN_POINT ( 'NONE',  ( 157.4999999999998295, 231.2854375337815327, 45.00000000000000000 ) ) ;
#26882=DIRECTION ( 'NONE',  ( -0.8916010070299882351, -0.4528218681370311249, 0.000000000000000000 ) ) ;
#26886=LINE ( 'NONE', #13539, #858 ) ;
#26887=VECTOR ( 'NONE', #26845, 1000.000000000000000 ) ;
#26890=CARTESIAN_POINT ( 'NONE',  ( 158.0000000000008242, 128.2086247222394206, -45.00000000000000000 ) ) ;
#26892=VECTOR ( 'NONE', #18981, 1000.000000000000000 ) ;
#26896=VERTEX_POINT ( 'NONE', #16803 ) ;
#26900=LINE ( 'NONE', #27307, #24870 ) ;
#26901=CARTESIAN_POINT ( 'NONE',  ( 157.9999999999996874, 269.1575001501400379, -45.00000000000000000 ) ) ;
#26907=ORIENTED_EDGE ( 'NONE', *, *, #6659, .F. ) ;
#26909=CARTESIAN_POINT ( 'NONE',  ( 157.4999999999998579, 221.2539375037535194, -45.00000000000000000 ) ) ;
#26910=ADVANCED_FACE ( 'NONE', ( #25001 ), #14097, .F. ) ;
#26911=EDGE_CURVE ( 'NONE', #5065, #1176, #12926, .T. ) ;
#26912=CARTESIAN_POINT ( 'NONE',  ( 157.9999999999996874, 266.6496251426330559, 45.00000000000000000 ) ) ;
#26913=DIRECTION ( 'NONE',  ( 0.8916010070298860946, -0.4528218681372321863, 0.000000000000000000 ) ) ;
#26917=LINE ( 'NONE', #24623, #4142 ) ;
#26918=DIRECTION ( 'NONE',  ( 1.000000000000000000, 0.000000000000000000, -0.000000000000000000 ) ) ;
#26919=ORIENTED_EDGE ( 'NONE', *, *, #19261, .F. ) ;
#26921=FACE_OUTER_BOUND ( 'NONE', #7829, .T. ) ;
#26922=LINE ( 'NONE', #7101, #26089 ) ;
#26925=ADVANCED_FACE ( 'NONE', ( #3860 ), #8747, .F. ) ;
#26929=LINE ( 'NONE', #16165, #4273 ) ;
#26934=ORIENTED_EDGE ( 'NONE', *, *, #2297, .F. ) ;
#26938=PLANE ( 'NONE',  #17244 ) ;
#26940=EDGE_CURVE ( 'NONE', #16172, #15403, #27981, .T. ) ;
#26941=EDGE_LOOP ( 'NONE', ( #8535, #6657, #16787, #17992 ) ) ;
#26943=VERTEX_POINT ( 'NONE', #19659 ) ;
#26962=CARTESIAN_POINT ( 'NONE',  ( 158.0000000000005116, 158.8109998198309825, 45.00000000000000000 ) ) ;
#26964=EDGE_CURVE ( 'NONE', #12431, #19520, #6017, .T. ) ;
#26966=DIRECTION ( 'NONE',  ( 0.8916010070298658885, -0.4528218681372722099, 0.000000000000000000 ) ) ;
#26967=ORIENTED_EDGE ( 'NONE', *, *, #25656, .T. ) ;
#26969=EDGE_CURVE ( 'NONE', #17314, #883, #14795, .T. ) ;
#26971=ORIENTED_EDGE ( 'NONE', *, *, #24973, .F. ) ;
#26979=VECTOR ( 'NONE', #4149, 1000.000000000000000 ) ;
#26980=LINE ( 'NONE', #7020, #4819 ) ;
#26982=EDGE_CURVE ( 'NONE', #13811, #23117, #6298, .T. ) ;
#26983=LINE ( 'NONE', #9756, #17249 ) ;
#26985=DIRECTION ( 'NONE',  ( 0.000000000000000000, -1.000000000000000000, 0.000000000000000000 ) ) ;
#26986=FACE_OUTER_BOUND ( 'NONE', #17440, .T. ) ;
#26995=ORIENTED_EDGE ( 'NONE', *, *, #16660, .F. ) ;
#26999=CARTESIAN_POINT ( 'NONE',  ( 157.4999999999994600, 216.2381874887387880, 45.00000000000000000 ) ) ;
#27000=EDGE_CURVE ( 'NONE', #2647, #14369, #23835, .T. ) ;
#27007=ORIENTED_EDGE ( 'NONE', *, *, #14742, .F. ) ;
#27009=DIRECTION ( 'NONE',  ( 0.8916010070293783896, -0.4528218681382319422, 0.000000000000000000 ) ) ;
#27010=CARTESIAN_POINT ( 'NONE',  ( 187.4999999999996305, 288.9665627064425166, 45.00000000000000000 ) ) ;
#27011=DIRECTION ( 'NONE',  ( -0.000000000000000000, -0.000000000000000000, -1.000000000000000000 ) ) ;
#27014=VECTOR ( 'NONE', #7105, 1000.000000000000227 ) ;
#27015=DIRECTION ( 'NONE',  ( 0.8916010070298766577, 0.4528218681372509491, 0.000000000000000000 ) ) ;
#27016=LINE ( 'NONE', #13972, #25174 ) ;
#27021=ADVANCED_BREP_SHAPE_REPRESENTATION ( '', ( #28013, #10637 ), #15244 ) ;
#27022=LINE ( 'NONE', #17985, #8324 ) ;
#27025=ORIENTED_EDGE ( 'NONE', *, *, #11675, .T. ) ;
#27030=CARTESIAN_POINT ( 'NONE',  ( 157.9999999999998295, 226.0157500150140208, 45.00000000000000000 ) ) ;
#27031=ORIENTED_EDGE ( 'NONE', *, *, #12376, .T. ) ;
#27032=VERTEX_POINT ( 'NONE', #6445 ) ;
#27033=CARTESIAN_POINT ( 'NONE',  ( 157.9999999999996874, 266.1417501351260171, -45.00000000000000000 ) ) ;
#27034=VECTOR ( 'NONE', #17876, 1000.000000000000000 ) ;
#27035=LINE ( 'NONE', #4621, #8062 ) ;
#27037=VECTOR ( 'NONE', #27183, 1000.000000000000000 ) ;
#27038=ORIENTED_EDGE ( 'NONE', *, *, #1996, .T. ) ;
#27042=DIRECTION ( 'NONE',  ( -0.000000000000000000, -0.000000000000000000, -1.000000000000000000 ) ) ;
#27043=ORIENTED_EDGE ( 'NONE', *, *, #22299, .T. ) ;
#27044=FACE_OUTER_BOUND ( 'NONE', #14013, .T. ) ;
#27045=ORIENTED_EDGE ( 'NONE', *, *, #14019, .F. ) ;
#27047=VECTOR ( 'NONE', #10199, 1000.000000000000000 ) ;
#27048=CARTESIAN_POINT ( 'NONE',  ( 157.4999999999998579, 80.81293708335913095, 45.00000000000000000 ) ) ;
#27049=LINE ( 'NONE', #20722, #3870 ) ;
#27052=CARTESIAN_POINT ( 'NONE',  ( 157.9999999999996305, 286.7126252026890256, 45.00000000000000000 ) ) ;
#27053=CARTESIAN_POINT ( 'NONE',  ( 157.4999999999998579, 83.32081209086616980, 45.00000000000000000 ) ) ;
#27057=CARTESIAN_POINT ( 'NONE',  ( 157.9999999999996589, 271.6653751576470768, -45.00000000000000000 ) ) ;
#27059=DIRECTION ( 'NONE',  ( 0.000000000000000000, -1.000000000000000000, 0.000000000000000000 ) ) ;
#27060=CARTESIAN_POINT ( 'NONE',  ( 157.4999999999998579, 143.5098122710352015, 45.00000000000000000 ) ) ;
#27061=ORIENTED_EDGE ( 'NONE', *, *, #16016, .T. ) ;
#27063=VECTOR ( 'NONE', #25966, 1000.000000000000114 ) ;
#27066=CARTESIAN_POINT ( 'NONE',  ( 157.4999999999998579, 88.33656210588026170, -45.00000000000000000 ) ) ;
#27069=PLANE ( 'NONE',  #17960 ) ;
#27070=FACE_OUTER_BOUND ( 'NONE', #5373, .T. ) ;
#27071=VERTEX_POINT ( 'NONE', #23693 ) ;
#27073=CARTESIAN_POINT ( 'NONE',  ( 157.9999999999997442, 251.0945000900840398, 45.00000000000000000 ) ) ;
#27078=DIRECTION ( 'NONE',  ( 1.000000000000000000, 0.000000000000000000, -0.000000000000000000 ) ) ;
#27079=ORIENTED_EDGE ( 'NONE', *, *, #13652, .T. ) ;
#27083=EDGE_CURVE ( 'NONE', #19656, #9422, #20081, .T. ) ;
#27086=EDGE_CURVE ( 'NONE', #152, #11767, #19943, .T. ) ;
#27087=DIRECTION ( 'NONE',  ( 0.4528218681382713551, -0.8916010070293584056, 0.000000000000000000 ) ) ;
#27088=CARTESIAN_POINT ( 'NONE',  ( 157.4999999999998579, 115.9231871884577174, -45.00000000000000000 ) ) ;
#27089=CARTESIAN_POINT ( 'NONE',  ( 157.4999999999998579, 68.27356204582390831, 45.00000000000000000 ) ) ;
#27091=DIRECTION ( 'NONE',  ( -0.000000000000000000, 0.000000000000000000, -1.000000000000000000 ) ) ;
#27093=LINE ( 'NONE', #26815, #20901 ) ;
#27097=VERTEX_POINT ( 'NONE', #2696 ) ;
#27099=DIRECTION ( 'NONE',  ( 0.4528218681378110011, 0.8916010070295922185, -0.000000000000000000 ) ) ;
#27100=PLANE ( 'NONE',  #25433 ) ;
#27101=CARTESIAN_POINT ( 'NONE',  ( 158.0000000000003126, 176.3661248723802828, 45.00000000000000000 ) ) ;
#27105=EDGE_CURVE ( 'NONE', #18947, #23572, #9468, .T. ) ;
#27110=ORIENTED_EDGE ( 'NONE', *, *, #2928, .F. ) ;
#27112=ORIENTED_EDGE ( 'NONE', *, *, #8640, .T. ) ;
#27113=DIRECTION ( 'NONE',  ( -0.000000000000000000, -0.000000000000000000, -1.000000000000000000 ) ) ;
#27116=FACE_OUTER_BOUND ( 'NONE', #18034, .T. ) ;
#27117=VECTOR ( 'NONE', #6061, 999.9999999999998863 ) ;
#27118=CARTESIAN_POINT ( 'NONE',  ( 157.4999999999996589, 281.4429376839215138, 45.00000000000000000 ) ) ;
#27120=LINE ( 'NONE', #2702, #25414 ) ;
#27124=CARTESIAN_POINT ( 'NONE',  ( 157.9999999999998010, 238.5551250525490161, 45.00000000000000000 ) ) ;
#27129=LINE ( 'NONE', #2994, #10594 ) ;
#27130=CARTESIAN_POINT ( 'NONE',  ( 157.4999999999998579, 130.9704372334999789, 45.00000000000000000 ) ) ;
#27135=ORIENTED_EDGE ( 'NONE', *, *, #11378, .T. ) ;
#27146=EDGE_LOOP ( 'NONE', ( #9092, #13782, #9466, #11799 ) ) ;
#27148=PLANE ( 'NONE',  #10115 ) ;
#27152=ADVANCED_FACE ( 'NONE', ( #22385 ), #9173, .F. ) ;
#27153=ADVANCED_FACE ( 'NONE', ( #26683 ), #412, .F. ) ;
#27157=DIRECTION ( 'NONE',  ( 0.000000000000000000, -1.000000000000000000, 0.000000000000000000 ) ) ;
#27160=FACE_OUTER_BOUND ( 'NONE', #1307, .T. ) ;
#27161=DIRECTION ( 'NONE',  ( 0.4528218681374320820, 0.8916010070297846202, -0.000000000000000000 ) ) ;
#27162=CARTESIAN_POINT ( 'NONE',  ( 157.4999999999998579, 138.4940622560211239, 45.00000000000000000 ) ) ;
#27167=DIRECTION ( 'NONE',  ( -0.000000000000000000, -0.000000000000000000, -1.000000000000000000 ) ) ;
#27168=ORIENTED_EDGE ( 'NONE', *, *, #1380, .T. ) ;
#27171=AXIS2_PLACEMENT_3D ( 'NONE', #18470, #3084, #12014 ) ;
#27175=ORIENTED_EDGE ( 'NONE', *, *, #6111, .T. ) ;
#27179=AXIS2_PLACEMENT_3D ( 'NONE', #4875, #26711, #12989 ) ;
#27183=DIRECTION ( 'NONE',  ( 0.000000000000000000, -1.000000000000000000, 0.000000000000000000 ) ) ;
#27184=VERTEX_POINT ( 'NONE', #9319 ) ;
#27185=PLANE ( 'NONE',  #9324 ) ;
#27186=EDGE_CURVE ( 'NONE', #1602, #25624, #18081, .T. ) ;
#27187=EDGE_CURVE ( 'NONE', #23117, #28088, #26837, .T. ) ;
#27191=DIRECTION ( 'NONE',  ( 1.000000000000000000, 0.000000000000000000, -0.000000000000000000 ) ) ;
#27195=ORIENTED_EDGE ( 'NONE', *, *, #22299, .F. ) ;
#27197=DIRECTION ( 'NONE',  ( -0.8916010070298049373, 0.4528218681373921140, 0.000000000000000000 ) ) ;
#27201=ORIENTED_EDGE ( 'NONE', *, *, #21835, .F. ) ;
#27203=VECTOR ( 'NONE', #18907, 1000.000000000000000 ) ;
#27208=ORIENTED_EDGE ( 'NONE', *, *, #10005, .T. ) ;
#27209=CARTESIAN_POINT ( 'NONE',  ( 157.4999999999998579, 43.19481197075347723, 45.00000000000000000 ) ) ;
#27210=ORIENTED_EDGE ( 'NONE', *, *, #11547, .T. ) ;
#27211=DIRECTION ( 'NONE',  ( -0.8916010070293783896, 0.4528218681382319422, 0.000000000000000000 ) ) ;
#27213=ORIENTED_EDGE ( 'NONE', *, *, #27346, .T. ) ;
#27216=CARTESIAN_POINT ( 'NONE',  ( 158.0000000000014779, 63.51174953456337136, 45.00000000000000000 ) ) ;
#27219=ORIENTED_EDGE ( 'NONE', *, *, #16229, .F. ) ;
#27223=EDGE_CURVE ( 'NONE', #24562, #3282, #22532, .T. ) ;
#27225=DIRECTION ( 'NONE',  ( -0.8916010070293383105, -0.4528218681383106015, 0.000000000000000000 ) ) ;
#27226=CARTESIAN_POINT ( 'NONE',  ( 158.0000000000000284, 203.9527499549551806, -45.00000000000000000 ) ) ;
#27227=CARTESIAN_POINT ( 'NONE',  ( 157.9999999999998579, 221.0000000000000284, -45.00000000000000000 ) ) ;
#27228=LINE ( 'NONE', #20909, #23512 ) ;
#27230=DIRECTION ( 'NONE',  ( -0.000000000000000000, -0.000000000000000000, -1.000000000000000000 ) ) ;
#27231=CARTESIAN_POINT ( 'NONE',  ( 157.9999999999999716, 208.9684999699701393, 45.00000000000000000 ) ) ;
#27235=VECTOR ( 'NONE', #22851, 1000.000000000000114 ) ;
#27238=DIRECTION ( 'NONE',  ( 0.8916010070294808632, 0.4528218681380302146, 0.000000000000000000 ) ) ;
#27242=CARTESIAN_POINT ( 'NONE',  ( 157.4999999999998579, 108.3995621659365867, 45.00000000000000000 ) ) ;
#27246=ADVANCED_FACE ( 'NONE', ( #12050 ), #11912, .F. ) ;
#27247=ORIENTED_EDGE ( 'NONE', *, *, #22662, .F. ) ;
#27248=ORIENTED_EDGE ( 'NONE', *, *, #23941, .F. ) ;
#27249=EDGE_LOOP ( 'NONE', ( #6926, #11394, #2261, #25568 ) ) ;
#27252=DIRECTION ( 'NONE',  ( -0.000000000000000000, -0.000000000000000000, -1.000000000000000000 ) ) ;
#27255=VECTOR ( 'NONE', #4901, 999.9999999999998863 ) ;
#27258=DIRECTION ( 'NONE',  ( -0.8916010070296936929, -0.4528218681376112165, 0.000000000000000000 ) ) ;
#27264=DIRECTION ( 'NONE',  ( 1.000000000000000000, 0.000000000000000000, -0.000000000000000000 ) ) ;
#27266=LINE ( 'NONE', #19077, #13943 ) ;
#27267=DIRECTION ( 'NONE',  ( -0.000000000000000000, -0.000000000000000000, -1.000000000000000000 ) ) ;
#27274=ADVANCED_FACE ( 'NONE', ( #27386 ), #23098, .F. ) ;
#27275=LINE ( 'NONE', #18663, #17540 ) ;
#27277=VECTOR ( 'NONE', #15923, 1000.000000000000000 ) ;
#27283=FACE_OUTER_BOUND ( 'NONE', #13633, .T. ) ;
#27284=DIRECTION ( 'NONE',  ( -0.000000000000000000, -0.000000000000000000, -1.000000000000000000 ) ) ;
#27285=DIRECTION ( 'NONE',  ( -0.8916010070299172918, -0.4528218681371710685, 0.000000000000000000 ) ) ;
#27287=CARTESIAN_POINT ( 'NONE',  ( 157.4999999999994884, 211.2224374737238577, 45.00000000000000000 ) ) ;
#27289=CARTESIAN_POINT ( 'NONE',  ( 157.4999999999996305, 283.9508126914284958, 45.00000000000000000 ) ) ;
#27290=VECTOR ( 'NONE', #21018, 1000.000000000000000 ) ;
#27291=FACE_OUTER_BOUND ( 'NONE', #4772, .T. ) ;
#27296=CARTESIAN_POINT ( 'NONE',  ( 157.9999999999996589, 276.6811251726610976, 45.00000000000000000 ) ) ;
#27297=VERTEX_POINT ( 'NONE', #20794 ) ;
#27298=CARTESIAN_POINT ( 'NONE',  ( 158.0000000000010800, 101.1298746471690038, -45.00000000000000000 ) ) ;
#27300=CARTESIAN_POINT ( 'NONE',  ( 157.4999999999998579, 168.5885623461056184, 45.00000000000000000 ) ) ;
#27303=EDGE_CURVE ( 'NONE', #8771, #20071, #5418, .T. ) ;
#27306=EDGE_CURVE ( 'NONE', #12327, #11955, #14201, .T. ) ;
#27307=CARTESIAN_POINT ( 'NONE',  ( 158.0000000000014211, 68.52749954957745615, 45.00000000000000000 ) ) ;
#27308=LINE ( 'NONE', #23431, #14962 ) ;
#27311=VERTEX_POINT ( 'NONE', #25389 ) ;
#27313=CARTESIAN_POINT ( 'NONE',  ( 157.9999999999997442, 253.6023750975910502, 45.00000000000000000 ) ) ;
#27314=DIRECTION ( 'NONE',  ( -0.000000000000000000, 0.000000000000000000, -1.000000000000000000 ) ) ;
#27319=CARTESIAN_POINT ( 'NONE',  ( 157.4999999999998579, 50.71843699327460797, -45.00000000000000000 ) ) ;
#27323=CARTESIAN_POINT ( 'NONE',  ( 158.0000000000003411, 173.8582498648732440, 45.00000000000000000 ) ) ;
#27326=LINE ( 'NONE', #24908, #22163 ) ;
#27327=VERTEX_POINT ( 'NONE', #18507 ) ;
#27328=EDGE_CURVE ( 'NONE', #991, #21625, #3684, .T. ) ;
#27331=LINE ( 'NONE', #7246, #16164 ) ;
#27334=CARTESIAN_POINT ( 'NONE',  ( 157.9999999999997726, 246.5866250825770294, 45.00000000000000000 ) ) ;
#27335=ORIENTED_EDGE ( 'NONE', *, *, #27000, .T. ) ;
#27346=EDGE_CURVE ( 'NONE', #12421, #378, #27667, .T. ) ;
#27349=VECTOR ( 'NONE', #28292, 1000.000000000000114 ) ;
#27351=DIRECTION ( 'NONE',  ( 1.000000000000000000, 0.000000000000000000, -0.000000000000000000 ) ) ;
#27352=ORIENTED_EDGE ( 'NONE', *, *, #4436, .F. ) ;
#27357=CARTESIAN_POINT ( 'NONE',  ( 157.4999999999998579, 191.1594374136689964, 45.00000000000000000 ) ) ;
#27359=CARTESIAN_POINT ( 'NONE',  ( 158.0000000000005400, 158.3031248123239436, 45.00000000000000000 ) ) ;
#27366=EDGE_LOOP ( 'NONE', ( #14262, #27195, #3136, #15594 ) ) ;
#27367=EDGE_CURVE ( 'NONE', #21137, #620, #836, .T. ) ;
#27370=CARTESIAN_POINT ( 'NONE',  ( 157.4999999999998579, 43.19481197075347723, -45.00000000000000000 ) ) ;
#27379=ORIENTED_EDGE ( 'NONE', *, *, #15112, .T. ) ;
#27381=EDGE_LOOP ( 'NONE', ( #25828, #1587, #4370, #10225 ) ) ;
#27382=ORIENTED_EDGE ( 'NONE', *, *, #24971, .T. ) ;
#27386=FACE_OUTER_BOUND ( 'NONE', #2622, .T. ) ;
#27391=CARTESIAN_POINT ( 'NONE',  ( 158.0000000000015348, 60.49599951954928656, 45.00000000000000000 ) ) ;
#27392=DIRECTION ( 'NONE',  ( 0.4528218681375107413, -0.8916010070297447632, 0.000000000000000000 ) ) ;
#27393=LINE ( 'NONE', #14213, #28254 ) ;
#27394=DIRECTION ( 'NONE',  ( -0.8916010070293383105, -0.4528218681383106015, 0.000000000000000000 ) ) ;
#27395=PLANE ( 'NONE',  #24691 ) ;
#27398=AXIS2_PLACEMENT_3D ( 'NONE', #22286, #7630, #9509 ) ;
#27399=EDGE_CURVE ( 'NONE', #3490, #13244, #1952, .T. ) ;
#27403=ORIENTED_EDGE ( 'NONE', *, *, #20136, .F. ) ;
#27408=ORIENTED_EDGE ( 'NONE', *, *, #16572, .T. ) ;
#27409=ORIENTED_EDGE ( 'NONE', *, *, #5590, .T. ) ;
#27410=VERTEX_POINT ( 'NONE', #28232 ) ;
#27412=EDGE_CURVE ( 'NONE', #16446, #7676, #3828, .T. ) ;
#27414=VERTEX_POINT ( 'NONE', #8713 ) ;
#27415=DIRECTION ( 'NONE',  ( 0.8916010070294909662, 0.4528218681380102306, 0.000000000000000000 ) ) ;
#27416=FACE_OUTER_BOUND ( 'NONE', #27737, .T. ) ;
#27419=PLANE ( 'NONE',  #25648 ) ;
#27420=LINE ( 'NONE', #28269, #167 ) ;
#27425=DIRECTION ( 'NONE',  ( -0.000000000000000000, 0.000000000000000000, -1.000000000000000000 ) ) ;
#27429=DIRECTION ( 'NONE',  ( -0.8916010070298766577, -0.4528218681372509491, 0.000000000000000000 ) ) ;
#27430=CARTESIAN_POINT ( 'NONE',  ( 157.4999999999998579, 78.30506207585207790, -45.00000000000000000 ) ) ;
#27433=CARTESIAN_POINT ( 'NONE',  ( 157.9999999999998863, 218.4921249924925348, -45.00000000000000000 ) ) ;
#27435=VECTOR ( 'NONE', #10172, 1000.000000000000227 ) ;
#27439=ORIENTED_EDGE ( 'NONE', *, *, #22946, .T. ) ;
#27441=EDGE_CURVE ( 'NONE', #1982, #9667, #21214, .T. ) ;
#27448=VECTOR ( 'NONE', #12313, 1000.000000000000000 ) ;
#27453=CARTESIAN_POINT ( 'NONE',  ( 157.9999999999997726, 244.0787500750700474, -45.00000000000000000 ) ) ;
#27454=VECTOR ( 'NONE', #27059, 1000.000000000000000 ) ;
#27457=LINE ( 'NONE', #25177, #11693 ) ;
#27459=DIRECTION ( 'NONE',  ( -1.000000000000000000, 1.850371707708594366E-15, 0.000000000000000000 ) ) ;
#27461=ADVANCED_FACE ( 'NONE', ( #767 ), #20156, .F. ) ;
#27464=ORIENTED_EDGE ( 'NONE', *, *, #20047, .F. ) ;
#27468=DIRECTION ( 'NONE',  ( -0.000000000000000000, -0.000000000000000000, -1.000000000000000000 ) ) ;
#27474=LINE ( 'NONE', #7814, #2437 ) ;
#27478=LINE ( 'NONE', #9835, #10169 ) ;
#27480=LINE ( 'NONE', #19151, #9288 ) ;
#27482=VECTOR ( 'NONE', #27267, 1000.000000000000000 ) ;
#27484=LINE ( 'NONE', #14575, #23675 ) ;
#27491=VERTEX_POINT ( 'NONE', #22314 ) ;
#27493=AXIS2_PLACEMENT_3D ( 'NONE', #4259, #19492, #15339 ) ;
#27495=ADVANCED_FACE ( 'NONE', ( #16005 ), #18429, .F. ) ;
#27498=EDGE_CURVE ( 'NONE', #17489, #226, #24613, .T. ) ;
#27499=CARTESIAN_POINT ( 'NONE',  ( 158.0000000000006821, 140.7479997597746433, 45.00000000000000000 ) ) ;
#27504=DIRECTION ( 'NONE',  ( 0.000000000000000000, -1.000000000000000000, 0.000000000000000000 ) ) ;
#27514=VERTEX_POINT ( 'NONE', #9673 ) ;
#27515=VECTOR ( 'NONE', #27225, 1000.000000000000114 ) ;
#27516=LINE ( 'NONE', #14328, #1507 ) ;
#27519=VERTEX_POINT ( 'NONE', #24758 ) ;
#27522=ORIENTED_EDGE ( 'NONE', *, *, #21568, .F. ) ;
#27524=DIRECTION ( 'NONE',  ( 0.000000000000000000, -1.000000000000000000, 0.000000000000000000 ) ) ;
#27525=CARTESIAN_POINT ( 'NONE',  ( 157.4999999999998579, 113.4153121809506786, 45.00000000000000000 ) ) ;
#27526=EDGE_CURVE ( 'NONE', #19430, #19942, #14130, .T. ) ;
#27527=CARTESIAN_POINT ( 'NONE',  ( 158.0000000000010516, 103.6377496546760568, 45.00000000000000000 ) ) ;
#27531=LINE ( 'NONE', #9613, #7164 ) ;
#27536=CARTESIAN_POINT ( 'NONE',  ( 157.9999999999997158, 258.6181251126050711, 45.00000000000000000 ) ) ;
#27538=CARTESIAN_POINT ( 'NONE',  ( 158.0000000000011084, 98.62199963966197913, -45.00000000000000000 ) ) ;
#27539=ORIENTED_EDGE ( 'NONE', *, *, #16032, .F. ) ;
#27540=AXIS2_PLACEMENT_3D ( 'NONE', #19924, #17766, #15349 ) ;
#27543=ORIENTED_EDGE ( 'NONE', *, *, #19187, .T. ) ;
#27544=VERTEX_POINT ( 'NONE', #18293 ) ;
#27551=EDGE_CURVE ( 'NONE', #25965, #12172, #904, .T. ) ;
#27556=VECTOR ( 'NONE', #21692, 1000.000000000000000 ) ;
#27557=ADVANCED_FACE ( 'NONE', ( #27044 ), #2914, .F. ) ;
#27559=LINE ( 'NONE', #27986, #28123 ) ;
#27562=DIRECTION ( 'NONE',  ( 0.000000000000000000, -1.000000000000000000, 0.000000000000000000 ) ) ;
#27563=DIRECTION ( 'NONE',  ( -0.000000000000000000, 0.000000000000000000, -1.000000000000000000 ) ) ;
#27569=LINE ( 'NONE', #14525, #1424 ) ;
#27572=AXIS2_PLACEMENT_3D ( 'NONE', #14294, #10396, #12146 ) ;
#27575=PLANE ( 'NONE',  #6220 ) ;
#27576=ORIENTED_EDGE ( 'NONE', *, *, #18562, .F. ) ;
#27582=LINE ( 'NONE', #14538, #5781 ) ;
#27585=DIRECTION ( 'NONE',  ( -0.8916010070295213863, -0.4528218681379502786, 0.000000000000000000 ) ) ;
#27587=VECTOR ( 'NONE', #5963, 1000.000000000000000 ) ;
#27589=DIRECTION ( 'NONE',  ( -0.8916010070293383105, -0.4528218681383106015, 0.000000000000000000 ) ) ;
#27591=CARTESIAN_POINT ( 'NONE',  ( 157.9999999999996589, 276.1732501651540588, -45.00000000000000000 ) ) ;
#27598=CARTESIAN_POINT ( 'NONE',  ( 158.0000000000011084, 98.62199963966197913, 45.00000000000000000 ) ) ;
#27600=DIRECTION ( 'NONE',  ( 1.000000000000000000, 0.000000000000000000, -0.000000000000000000 ) ) ;
#27601=EDGE_CURVE ( 'NONE', #19699, #4657, #8359, .T. ) ;
#27603=LINE ( 'NONE', #16570, #23203 ) ;
#27604=EDGE_LOOP ( 'NONE', ( #16932, #18832, #27464, #10753 ) ) ;
#27606=CARTESIAN_POINT ( 'NONE',  ( 157.9999999999997726, 246.0787500750700474, 45.00000000000000000 ) ) ;
#27608=FACE_OUTER_BOUND ( 'NONE', #25835, .T. ) ;
#27610=VERTEX_POINT ( 'NONE', #27591 ) ;
#27611=VECTOR ( 'NONE', #901, 1000.000000000000000 ) ;
#27615=CARTESIAN_POINT ( 'NONE',  ( 157.4999999999998579, 90.84443711338730054, -45.00000000000000000 ) ) ;
#27616=DIRECTION ( 'NONE',  ( 0.8916010070293710621, -0.4528218681382463195, 0.000000000000000000 ) ) ;
#27617=CARTESIAN_POINT ( 'NONE',  ( 157.9999999999996305, 283.6968751876750616, 45.00000000000000000 ) ) ;
#27620=LINE ( 'NONE', #21306, #3324 ) ;
#27621=VERTEX_POINT ( 'NONE', #5490 ) ;
#27623=AXIS2_PLACEMENT_3D ( 'NONE', #16997, #18732, #23465 ) ;
#27624=DIRECTION ( 'NONE',  ( -0.000000000000000000, -0.000000000000000000, -1.000000000000000000 ) ) ;
#27625=FACE_OUTER_BOUND ( 'NONE', #27146, .T. ) ;
#27632=VERTEX_POINT ( 'NONE', #16836 ) ;
#27633=ORIENTED_EDGE ( 'NONE', *, *, #28125, .T. ) ;
#27634=VECTOR ( 'NONE', #11486, 1000.000000000000000 ) ;
#27636=VECTOR ( 'NONE', #25786, 1000.000000000000227 ) ;
#27640=DIRECTION ( 'NONE',  ( 0.8916010070294498879, -0.4528218681380914434, 0.000000000000000000 ) ) ;
#27644=LINE ( 'NONE', #26061, #13874 ) ;
#27647=ORIENTED_EDGE ( 'NONE', *, *, #3719, .T. ) ;
#27649=DIRECTION ( 'NONE',  ( -0.8916010070293384215, 0.4528218681383106015, 0.000000000000000000 ) ) ;
#27652=CARTESIAN_POINT ( 'NONE',  ( 158.0000000000011937, 93.09837461714084839, 45.00000000000000000 ) ) ;
#27655=VECTOR ( 'NONE', #503, 1000.000000000000000 ) ;
#27656=LINE ( 'NONE', #6257, #27203 ) ;
#27667=LINE ( 'NONE', #8008, #16948 ) ;
#27674=AXIS2_PLACEMENT_3D ( 'NONE', #13561, #23903, #15434 ) ;
#27681=LINE ( 'NONE', #25401, #8633 ) ;
#27685=CARTESIAN_POINT ( 'NONE',  ( 158.0000000000014211, 68.52749954957745615, -45.00000000000000000 ) ) ;
#27687=EDGE_LOOP ( 'NONE', ( #8420, #8001, #8496, #9828 ) ) ;
#27692=EDGE_CURVE ( 'NONE', #3711, #8035, #17825, .T. ) ;
#27700=ORIENTED_EDGE ( 'NONE', *, *, #19042, .F. ) ;
#27701=CARTESIAN_POINT ( 'NONE',  ( 157.9999999999998010, 241.0630000600560550, -45.00000000000000000 ) ) ;
#27706=DIRECTION ( 'NONE',  ( -0.000000000000000000, -0.000000000000000000, -1.000000000000000000 ) ) ;
#27707=CARTESIAN_POINT ( 'NONE',  ( 157.4999999999998579, 83.32081209086616980, -45.00000000000000000 ) ) ;
#27711=CARTESIAN_POINT ( 'NONE',  ( 158.0000000000007958, 130.7164997297464595, 45.00000000000000000 ) ) ;
#27713=VECTOR ( 'NONE', #12315, 1000.000000000000000 ) ;
#27716=EDGE_CURVE ( 'NONE', #15041, #11767, #2883, .T. ) ;
#27719=EDGE_LOOP ( 'NONE', ( #22422, #7892, #12706, #8172 ) ) ;
#27721=ORIENTED_EDGE ( 'NONE', *, *, #11937, .T. ) ;
#27722=EDGE_LOOP ( 'NONE', ( #10723, #28310, #3506, #12541 ) ) ;
#27723=LINE ( 'NONE', #8064, #25759 ) ;
#27727=VECTOR ( 'NONE', #18336, 1000.000000000000000 ) ;
#27730=FACE_OUTER_BOUND ( 'NONE', #23858, .T. ) ;
#27733=PLANE ( 'NONE',  #1499 ) ;
#27737=EDGE_LOOP ( 'NONE', ( #21307, #25564, #5801, #23898 ) ) ;
#27742=CARTESIAN_POINT ( 'NONE',  ( 158.0000000000004263, 168.3346248423521274, 45.00000000000000000 ) ) ;
#27743=PLANE ( 'NONE',  #9130 ) ;
#27744=LINE ( 'NONE', #10523, #2795 ) ;
#27746=ORIENTED_EDGE ( 'NONE', *, *, #13524, .F. ) ;
#27747=CARTESIAN_POINT ( 'NONE',  ( 158.0000000000002274, 183.8897498949014278, -45.00000000000000000 ) ) ;
#27750=CARTESIAN_POINT ( 'NONE',  ( 158.0000000000007958, 130.7164997297464595, 45.00000000000000000 ) ) ;
#27753=CARTESIAN_POINT ( 'NONE',  ( 157.4999999999997442, 251.3484375938375024, 45.00000000000000000 ) ) ;
#27756=PLANE ( 'NONE',  #1078 ) ;
#27759=ORIENTED_EDGE ( 'NONE', *, *, #7742, .F. ) ;
#27765=DIRECTION ( 'NONE',  ( -0.8916010070295004031, 0.4528218681379916344, 0.000000000000000000 ) ) ;
#27769=ORIENTED_EDGE ( 'NONE', *, *, #28335, .T. ) ;
#27770=ADVANCED_FACE ( 'NONE', ( #17638 ), #2541, .F. ) ;
#27773=ORIENTED_EDGE ( 'NONE', *, *, #26700, .F. ) ;
#27774=ORIENTED_EDGE ( 'NONE', *, *, #4257, .T. ) ;
#27779=LINE ( 'NONE', #7976, #1827 ) ;
#27780=VECTOR ( 'NONE', #1262, 999.9999999999998863 ) ;
#27781=EDGE_CURVE ( 'NONE', #20027, #14958, #13480, .T. ) ;
#27787=DIRECTION ( 'NONE',  ( -0.8916010070293584056, -0.4528218681382712996, 0.000000000000000000 ) ) ;
#27790=ORIENTED_EDGE ( 'NONE', *, *, #11547, .F. ) ;
#27792=PLANE ( 'NONE',  #4577 ) ;
#27793=CARTESIAN_POINT ( 'NONE',  ( 158.0000000000013358, 80.55899957960563995, 45.00000000000000000 ) ) ;
#27795=CARTESIAN_POINT ( 'NONE',  ( 157.4999999999998579, 151.0334372935563465, -45.00000000000000000 ) ) ;
#27804=LINE ( 'NONE', #5840, #11777 ) ;
#27805=VERTEX_POINT ( 'NONE', #6859 ) ;
#27807=CARTESIAN_POINT ( 'NONE',  ( 158.0000000000010516, 103.6377496546760568, 45.00000000000000000 ) ) ;
#27812=DIRECTION ( 'NONE',  ( -0.000000000000000000, -0.000000000000000000, -1.000000000000000000 ) ) ;
#27819=FACE_OUTER_BOUND ( 'NONE', #26573, .T. ) ;
#27824=LINE ( 'NONE', #27685, #22909 ) ;
#27827=ORIENTED_EDGE ( 'NONE', *, *, #24606, .F. ) ;
#27831=ORIENTED_EDGE ( 'NONE', *, *, #5826, .T. ) ;
#27832=VECTOR ( 'NONE', #9209, 1000.000000000000000 ) ;
#27833=EDGE_LOOP ( 'NONE', ( #18038, #16179, #11830, #7441 ) ) ;
#27835=ORIENTED_EDGE ( 'NONE', *, *, #2197, .F. ) ;
#27837=ORIENTED_EDGE ( 'NONE', *, *, #8053, .T. ) ;
#27839=LINE ( 'NONE', #27984, #13765 ) ;
#27840=DIRECTION ( 'NONE',  ( 1.000000000000000000, 0.000000000000000000, -0.000000000000000000 ) ) ;
#27843=EDGE_CURVE ( 'NONE', #8245, #18572, #7298, .T. ) ;
#27853=DIRECTION ( 'NONE',  ( 0.000000000000000000, -1.000000000000000000, 0.000000000000000000 ) ) ;
#27854=VERTEX_POINT ( 'NONE', #13632 ) ;
#27855=DIRECTION ( 'NONE',  ( -0.000000000000000000, -0.000000000000000000, -1.000000000000000000 ) ) ;
#27862=CARTESIAN_POINT ( 'NONE',  ( 157.4999999999998579, 70.78143705333094715, -45.00000000000000000 ) ) ;
#27864=ORIENTED_EDGE ( 'NONE', *, *, #24633, .T. ) ;
#27865=ORIENTED_EDGE ( 'NONE', *, *, #8729, .T. ) ;
#27869=ORIENTED_EDGE ( 'NONE', *, *, #22198, .T. ) ;
#27871=VERTEX_POINT ( 'NONE', #13921 ) ;
#27873=ADVANCED_FACE ( 'NONE', ( #3250 ), #18074, .F. ) ;
#27877=CARTESIAN_POINT ( 'NONE',  ( 158.0000000000007390, 133.7322497447605656, 45.00000000000000000 ) ) ;
#27881=DIRECTION ( 'NONE',  ( 0.000000000000000000, -1.000000000000000000, 0.000000000000000000 ) ) ;
#27882=VECTOR ( 'NONE', #3661, 1000.000000000000000 ) ;
#27884=DIRECTION ( 'NONE',  ( 0.000000000000000000, 0.000000000000000000, -1.000000000000000000 ) ) ;
#27887=DIRECTION ( 'NONE',  ( -0.000000000000000000, 0.000000000000000000, -1.000000000000000000 ) ) ;
#27888=CARTESIAN_POINT ( 'NONE',  ( 158.0000000000001705, 190.9054999099155054, 45.00000000000000000 ) ) ;
#27890=ORIENTED_EDGE ( 'NONE', *, *, #13350, .F. ) ;
#27891=LINE ( 'NONE', #12277, #12371 ) ;
#27893=DIRECTION ( 'NONE',  ( 0.000000000000000000, -1.000000000000000000, 0.000000000000000000 ) ) ;
#27896=PLANE ( 'NONE',  #27623 ) ;
#27897=VERTEX_POINT ( 'NONE', #20504 ) ;
#27898=CARTESIAN_POINT ( 'NONE',  ( 157.9999999999996305, 281.6968751876750616, -45.00000000000000000 ) ) ;
#27899=CARTESIAN_POINT ( 'NONE',  ( 158.0000000000014495, 68.01962454207041731, -45.00000000000000000 ) ) ;
#27901=VERTEX_POINT ( 'NONE', #2974 ) ;
#27903=EDGE_LOOP ( 'NONE', ( #17480, #1781, #20019, #24252 ) ) ;
#27904=VECTOR ( 'NONE', #19175, 1000.000000000000000 ) ;
#27905=AXIS2_PLACEMENT_3D ( 'NONE', #18578, #27191, #4924 ) ;
#27907=ORIENTED_EDGE ( 'NONE', *, *, #18143, .F. ) ;
#27910=EDGE_CURVE ( 'NONE', #5522, #14116, #5411, .T. ) ;
#27911=PLANE ( 'NONE',  #19507 ) ;
#27912=LINE ( 'NONE', #4218, #22197 ) ;
#27919=VECTOR ( 'NONE', #18449, 1000.000000000000227 ) ;
#27921=CARTESIAN_POINT ( 'NONE',  ( 157.4999999999998579, 98.36806213590843129, 45.00000000000000000 ) ) ;
#27924=ORIENTED_EDGE ( 'NONE', *, *, #5449, .F. ) ;
#27925=DIRECTION ( 'NONE',  ( 0.000000000000000000, -1.000000000000000000, 0.000000000000000000 ) ) ;
#27926=AXIS2_PLACEMENT_3D ( 'NONE', #8162, #21374, #1690 ) ;
#27927=EDGE_CURVE ( 'NONE', #3903, #4479, #12040, .T. ) ;
#27931=CARTESIAN_POINT ( 'NONE',  ( 157.9999999999996589, 279.1890001801680796, -45.00000000000000000 ) ) ;
#27937=ORIENTED_EDGE ( 'NONE', *, *, #23856, .T. ) ;
#27940=DIRECTION ( 'NONE',  ( 1.000000000000000000, 0.000000000000000000, -0.000000000000000000 ) ) ;
#27943=ORIENTED_EDGE ( 'NONE', *, *, #16810, .F. ) ;
#27946=DIRECTION ( 'NONE',  ( -0.8916010070293409751, -0.4528218681383056610, 0.000000000000000000 ) ) ;
#27948=EDGE_CURVE ( 'NONE', #6335, #620, #24961, .T. ) ;
#27952=CARTESIAN_POINT ( 'NONE',  ( 158.0000000000016200, 50.97237449702815582, 45.00000000000000000 ) ) ;
#27957=DIRECTION ( 'NONE',  ( -0.000000000000000000, -0.000000000000000000, -1.000000000000000000 ) ) ;
#27963=VECTOR ( 'NONE', #27812, 1000.000000000000000 ) ;
#27972=ORIENTED_EDGE ( 'NONE', *, *, #23541, .T. ) ;
#27974=ORIENTED_EDGE ( 'NONE', *, *, #18190, .F. ) ;
#27978=ORIENTED_EDGE ( 'NONE', *, *, #4780, .F. ) ;
#27981=LINE ( 'NONE', #21392, #25559 ) ;
#27982=EDGE_CURVE ( 'NONE', #12064, #19409, #8131, .T. ) ;
#27983=VECTOR ( 'NONE', #20052, 1000.000000000000000 ) ;
#27984=CARTESIAN_POINT ( 'NONE',  ( 157.4999999999996589, 276.4271876689075498, -45.00000000000000000 ) ) ;
#27986=CARTESIAN_POINT ( 'NONE',  ( 158.0000000000000853, 196.4291249324366504, 45.00000000000000000 ) ) ;
#27987=VECTOR ( 'NONE', #3766, 1000.000000000000000 ) ;
#27993=LINE ( 'NONE', #20976, #11437 ) ;
#28000=DIRECTION ( 'NONE',  ( -0.000000000000000000, -0.000000000000000000, -1.000000000000000000 ) ) ;
#28004=ORIENTED_EDGE ( 'NONE', *, *, #10419, .F. ) ;
#28009=VERTEX_POINT ( 'NONE', #25372 ) ;
#28013=MANIFOLD_SOLID_BREP ( '\X2\00d8\X0\12.0mm Dowel Hole3[1]', #1702 ) ;
#28015=DIRECTION ( 'NONE',  ( -0.000000000000000000, -0.000000000000000000, -1.000000000000000000 ) ) ;
#28018=ORIENTED_EDGE ( 'NONE', *, *, #3997, .T. ) ;
#28020=PLANE ( 'NONE',  #26810 ) ;
#28026=ADVANCED_FACE ( 'NONE', ( #26484 ), #25789, .F. ) ;
#28027=LINE ( 'NONE', #17547, #17011 ) ;
#28031=DIRECTION ( 'NONE',  ( 0.8916010070299571488, -0.4528218681370922982, 0.000000000000000000 ) ) ;
#28033=DIRECTION ( 'NONE',  ( -0.000000000000000000, 0.000000000000000000, -1.000000000000000000 ) ) ;
#28034=CARTESIAN_POINT ( 'NONE',  ( 157.4999999999998579, 181.1279373836408411, -45.00000000000000000 ) ) ;
#28036=FACE_OUTER_BOUND ( 'NONE', #7054, .T. ) ;
#28037=ORIENTED_EDGE ( 'NONE', *, *, #13599, .F. ) ;
#28041=ORIENTED_EDGE ( 'NONE', *, *, #17709, .T. ) ;
#28042=EDGE_CURVE ( 'NONE', #7826, #1981, #12740, .T. ) ;
#28046=EDGE_CURVE ( 'NONE', #5196, #4740, #10999, .T. ) ;
#28055=FACE_OUTER_BOUND ( 'NONE', #6090, .T. ) ;
#28060=EDGE_LOOP ( 'NONE', ( #20110, #25122, #19607, #756 ) ) ;
#28061=AXIS2_PLACEMENT_3D ( 'NONE', #6769, #22002, #8936 ) ;
#28062=FACE_OUTER_BOUND ( 'NONE', #3315, .T. ) ;
#28064=AXIS2_PLACEMENT_3D ( 'NONE', #18202, #26655, #17619 ) ;
#28068=ORIENTED_EDGE ( 'NONE', *, *, #4272, .T. ) ;
#28069=CARTESIAN_POINT ( 'NONE',  ( 157.9999999999998010, 236.5551250525490161, 45.00000000000000000 ) ) ;
#28070=VECTOR ( 'NONE', #17311, 1000.000000000000000 ) ;
#28074=CARTESIAN_POINT ( 'NONE',  ( 158.0000000000000284, 205.9527499549551806, -45.00000000000000000 ) ) ;
#28076=VERTEX_POINT ( 'NONE', #21623 ) ;
#28077=EDGE_CURVE ( 'NONE', #5655, #477, #6253, .T. ) ;
#28081=ORIENTED_EDGE ( 'NONE', *, *, #4959, .T. ) ;
#28083=EDGE_LOOP ( 'NONE', ( #21708, #3347, #11534, #25477 ) ) ;
#28088=VERTEX_POINT ( 'NONE', #28074 ) ;
#28093=VECTOR ( 'NONE', #14711, 1000.000000000000000 ) ;
#28094=EDGE_CURVE ( 'NONE', #1213, #8138, #4513, .T. ) ;
#28103=DIRECTION ( 'NONE',  ( 0.8916010070295715684, -0.4528218681378516353, 0.000000000000000000 ) ) ;
#28105=EDGE_CURVE ( 'NONE', #8173, #23544, #26211, .T. ) ;
#28113=ORIENTED_EDGE ( 'NONE', *, *, #11888, .F. ) ;
#28117=VERTEX_POINT ( 'NONE', #15319 ) ;
#28121=ORIENTED_EDGE ( 'NONE', *, *, #4531, .T. ) ;
#28123=VECTOR ( 'NONE', #5739, 1000.000000000000000 ) ;
#28125=EDGE_CURVE ( 'NONE', #4623, #22496, #4375, .T. ) ;
#28126=VECTOR ( 'NONE', #23460, 1000.000000000000000 ) ;
#28128=CARTESIAN_POINT ( 'NONE',  ( 158.0000000000002842, 180.8739998798873501, 45.00000000000000000 ) ) ;
#28129=AXIS2_PLACEMENT_3D ( 'NONE', #14318, #16473, #5688 ) ;
#28131=CARTESIAN_POINT ( 'NONE',  ( 158.0000000000000568, 201.4448749474510407, 45.00000000000000000 ) ) ;
#28139=CARTESIAN_POINT ( 'NONE',  ( 158.0000000000005684, 151.2873747973098659, -45.00000000000000000 ) ) ;
#28140=CARTESIAN_POINT ( 'NONE',  ( 157.4999999999996589, 281.4429376839215138, 45.00000000000000000 ) ) ;
#28142=VECTOR ( 'NONE', #4996, 1000.000000000000000 ) ;
#28146=ORIENTED_EDGE ( 'NONE', *, *, #9816, .F. ) ;
#28148=AXIS2_PLACEMENT_3D ( 'NONE', #22584, #11818, #20557 ) ;
#28150=VERTEX_POINT ( 'NONE', #15459 ) ;
#28152=DIRECTION ( 'NONE',  ( -0.000000000000000000, 0.000000000000000000, -1.000000000000000000 ) ) ;
#28153=ORIENTED_EDGE ( 'NONE', *, *, #9786, .T. ) ;
#28158=CARTESIAN_POINT ( 'NONE',  ( 158.0000000000012790, 83.57474959461971764, -45.00000000000000000 ) ) ;
#28159=CARTESIAN_POINT ( 'NONE',  ( 158.0000000000005400, 156.3031248123239436, 45.00000000000000000 ) ) ;
#28160=ORIENTED_EDGE ( 'NONE', *, *, #10483, .T. ) ;
#28162=ORIENTED_EDGE ( 'NONE', *, *, #28046, .T. ) ;
#28165=DIRECTION ( 'NONE',  ( -0.000000000000000000, 0.000000000000000000, -1.000000000000000000 ) ) ;
#28168=LINE ( 'NONE', #20094, #19771 ) ;
#28170=LINE ( 'NONE', #24027, #10933 ) ;
#28171=DIRECTION ( 'NONE',  ( 1.000000000000000000, 0.000000000000000000, -0.000000000000000000 ) ) ;
#28172=DIRECTION ( 'NONE',  ( 0.8916010070300181001, -0.4528218681369723941, 0.000000000000000000 ) ) ;
#28173=DIRECTION ( 'NONE',  ( -0.000000000000000000, -0.000000000000000000, -1.000000000000000000 ) ) ;
#28176=EDGE_CURVE ( 'NONE', #2326, #9517, #24208, .T. ) ;
#28179=CARTESIAN_POINT ( 'NONE',  ( 157.9999999999998010, 233.5393750375350237, 45.00000000000000000 ) ) ;
#28180=ORIENTED_EDGE ( 'NONE', *, *, #27399, .F. ) ;
#28181=CARTESIAN_POINT ( 'NONE',  ( 158.0000000000002842, 178.8739998798873216, 45.00000000000000000 ) ) ;
#28187=VECTOR ( 'NONE', #1829, 1000.000000000000227 ) ;
#28188=ORIENTED_EDGE ( 'NONE', *, *, #3209, .F. ) ;
#28191=ORIENTED_EDGE ( 'NONE', *, *, #21511, .T. ) ;
#28194=ADVANCED_FACE ( 'NONE', ( #24343 ), #27069, .F. ) ;
#28195=CARTESIAN_POINT ( 'NONE',  ( 157.9999999999999147, 215.9842499849850697, -45.00000000000000000 ) ) ;
#28196=LINE ( 'NONE', #8542, #7060 ) ;
#28198=VECTOR ( 'NONE', #19769, 1000.000000000000000 ) ;
#28199=AXIS2_PLACEMENT_3D ( 'NONE', #8302, #5575, #14491 ) ;
#28203=ORIENTED_EDGE ( 'NONE', *, *, #7062, .T. ) ;
#28206=VECTOR ( 'NONE', #9381, 1000.000000000000000 ) ;
#28207=FACE_OUTER_BOUND ( 'NONE', #23424, .T. ) ;
#28208=DIRECTION ( 'NONE',  ( 0.4528218681380914989, 0.8916010070294497769, -0.000000000000000000 ) ) ;
#28209=CARTESIAN_POINT ( 'NONE',  ( 157.9999999999998295, 229.0315000300280417, -45.00000000000000000 ) ) ;
#28211=EDGE_CURVE ( 'NONE', #19047, #24186, #9695, .T. ) ;
#28213=ADVANCED_FACE ( 'NONE', ( #9122 ), #17883, .F. ) ;
#28215=DIRECTION ( 'NONE',  ( -0.000000000000000000, -0.000000000000000000, -1.000000000000000000 ) ) ;
#28217=CARTESIAN_POINT ( 'NONE',  ( 158.0000000000007674, 131.2243747372535267, -45.00000000000000000 ) ) ;
#28218=DIRECTION ( 'NONE',  ( 0.000000000000000000, -1.000000000000000000, 0.000000000000000000 ) ) ;
#28219=LINE ( 'NONE', #4096, #12499 ) ;
#28222=ORIENTED_EDGE ( 'NONE', *, *, #9327, .T. ) ;
#28227=DIRECTION ( 'NONE',  ( -0.000000000000000000, -0.000000000000000000, -1.000000000000000000 ) ) ;
#28228=ORIENTED_EDGE ( 'NONE', *, *, #5449, .T. ) ;
#28232=CARTESIAN_POINT ( 'NONE',  ( 158.0000000000012790, 83.57474959461971764, 45.00000000000000000 ) ) ;
#28234=CARTESIAN_POINT ( 'NONE',  ( 158.0000000000017337, 40.94087446699997912, -45.00000000000000000 ) ) ;
#28243=LINE ( 'NONE', #11314, #11739 ) ;
#28250=EDGE_CURVE ( 'NONE', #15878, #3625, #22772, .T. ) ;
#28254=VECTOR ( 'NONE', #22963, 1000.000000000000000 ) ;
#28255=ORIENTED_EDGE ( 'NONE', *, *, #25375, .F. ) ;
#28260=ORIENTED_EDGE ( 'NONE', *, *, #15595, .F. ) ;
#28263=EDGE_LOOP ( 'NONE', ( #17641, #25183, #21952, #2547 ) ) ;
#28264=ORIENTED_EDGE ( 'NONE', *, *, #16537, .T. ) ;
#28265=AXIS2_PLACEMENT_3D ( 'NONE', #24008, #6046, #23864 ) ;
#28267=PLANE ( 'NONE',  #21078 ) ;
#28269=CARTESIAN_POINT ( 'NONE',  ( 157.9999999999997158, 258.6181251126050711, 45.00000000000000000 ) ) ;
#28272=FACE_OUTER_BOUND ( 'NONE', #21103, .T. ) ;
#28278=LINE ( 'NONE', #6176, #27556 ) ;
#28281=EDGE_LOOP ( 'NONE', ( #18075, #26000, #7041, #16243 ) ) ;
#28285=EDGE_CURVE ( 'NONE', #25380, #1111, #11725, .T. ) ;
#28292=DIRECTION ( 'NONE',  ( -0.8916010070293383105, -0.4528218681383106015, 0.000000000000000000 ) ) ;
#28296=EDGE_CURVE ( 'NONE', #8138, #8166, #16584, .T. ) ;
#28297=DIRECTION ( 'NONE',  ( -0.8916010070297244461, -0.4528218681375507093, 0.000000000000000000 ) ) ;
#28298=ORIENTED_EDGE ( 'NONE', *, *, #19, .T. ) ;
#28305=ORIENTED_EDGE ( 'NONE', *, *, #25834, .T. ) ;
#28307=CARTESIAN_POINT ( 'NONE',  ( 157.9999999999997442, 251.6023750975910218, -45.00000000000000000 ) ) ;
#28308=CARTESIAN_POINT ( 'NONE',  ( 157.4999999999996589, 276.4271876689075498, 45.00000000000000000 ) ) ;
#28309=CARTESIAN_POINT ( 'NONE',  ( 157.4999999999998579, 53.22631200078164682, -45.00000000000000000 ) ) ;
#28310=ORIENTED_EDGE ( 'NONE', *, *, #17289, .F. ) ;
#28312=EDGE_CURVE ( 'NONE', #8626, #5381, #25609, .T. ) ;
#28317=ORIENTED_EDGE ( 'NONE', *, *, #20357, .F. ) ;
#28319=VECTOR ( 'NONE', #25526, 1000.000000000000000 ) ;
#28322=EDGE_LOOP ( 'NONE', ( #1898, #16183, #10349, #12714 ) ) ;
#28323=ADVANCED_FACE ( 'NONE', ( #25195 ), #12283, .F. ) ;
#28327=ORIENTED_EDGE ( 'NONE', *, *, #15350, .F. ) ;
#28329=ADVANCED_FACE ( 'NONE', ( #14433 ), #23045, .F. ) ;
#28331=EDGE_CURVE ( 'NONE', #3105, #18450, #14710, .T. ) ;
#28335=EDGE_CURVE ( 'NONE', #1943, #23236, #27478, .T. ) ;
#28339=DIRECTION ( 'NONE',  ( 0.4528218681383056610, -0.8916010070293409751, 0.000000000000000000 ) ) ;
#28341=PLANE ( 'NONE',  #13628 ) ;
#28342=CARTESIAN_POINT ( 'NONE',  ( 157.4999999999996589, 273.9193126614005678, -45.00000000000000000 ) ) ;
#28343=CARTESIAN_POINT ( 'NONE',  ( 157.9999999999998010, 231.5393750375350237, 45.00000000000000000 ) ) ;
#28344=CARTESIAN_POINT ( 'NONE',  ( 157.9999999999998295, 228.5236250225210313, -45.00000000000000000 ) ) ;
#28345=ORIENTED_EDGE ( 'NONE', *, *, #22006, .F. ) ;
#28346=LINE ( 'NONE', #6951, #20143 ) ;
#28349=DIRECTION ( 'NONE',  ( 0.4528218681376312005, -0.8916010070296835899, 0.000000000000000000 ) ) ;
#28350=DIRECTION ( 'NONE',  ( -0.8916010070299273949, -0.4528218681371510845, 0.000000000000000000 ) ) ;
#28353=CARTESIAN_POINT ( 'NONE',  ( 157.9999999999997158, 261.1260001201120531, -45.00000000000000000 ) ) ;
#28354=EDGE_LOOP ( 'NONE', ( #18312, #10900, #17875, #8455 ) ) ;
#28359=DIRECTION ( 'NONE',  ( 0.8916010070295309342, -0.4528218681379315713, 0.000000000000000000 ) ) ;
#28360=ORIENTED_EDGE ( 'NONE', *, *, #24154, .F. ) ;
#28361=EDGE_CURVE ( 'NONE', #19423, #1670, #1069, .T. ) ;
#28372=LINE ( 'NONE', #17618, #14473 ) ;
#28375=VECTOR ( 'NONE', #17088, 1000.000000000000000 ) ;
#28379=DIRECTION ( 'NONE',  ( 0.000000000000000000, -1.000000000000000000, 0.000000000000000000 ) ) ;
#28381=CARTESIAN_POINT ( 'NONE',  ( 158.0000000000003695, 173.3503748573662051, 45.00000000000000000 ) ) ;
#28383=CARTESIAN_POINT ( 'NONE',  ( 158.0000000000009663, 111.1613746771971876, -45.00000000000000000 ) ) ;
#28385=ORIENTED_EDGE ( 'NONE', *, *, #794, .F. ) ;
#28388=EDGE_LOOP ( 'NONE', ( #9959, #9024, #17149, #2942 ) ) ;
#28397=ORIENTED_EDGE ( 'NONE', *, *, #23602, .F. ) ;
#28421=COLOUR_RGB('Light Blue',0.38,0.62,0.78);
#28422=FILL_AREA_STYLE_COLOUR('',#28421);
#28423=FILL_AREA_STYLE('',(#28422));
#28424=SURFACE_STYLE_FILL_AREA(#28423);
#28425=SURFACE_SIDE_STYLE('',(#28424));
#28426=SURFACE_STYLE_USAGE(.BOTH.,#28425);
#28427=PRESENTATION_STYLE_ASSIGNMENT((#28426));
ENDSEC;
END-ISO-10303-21;
